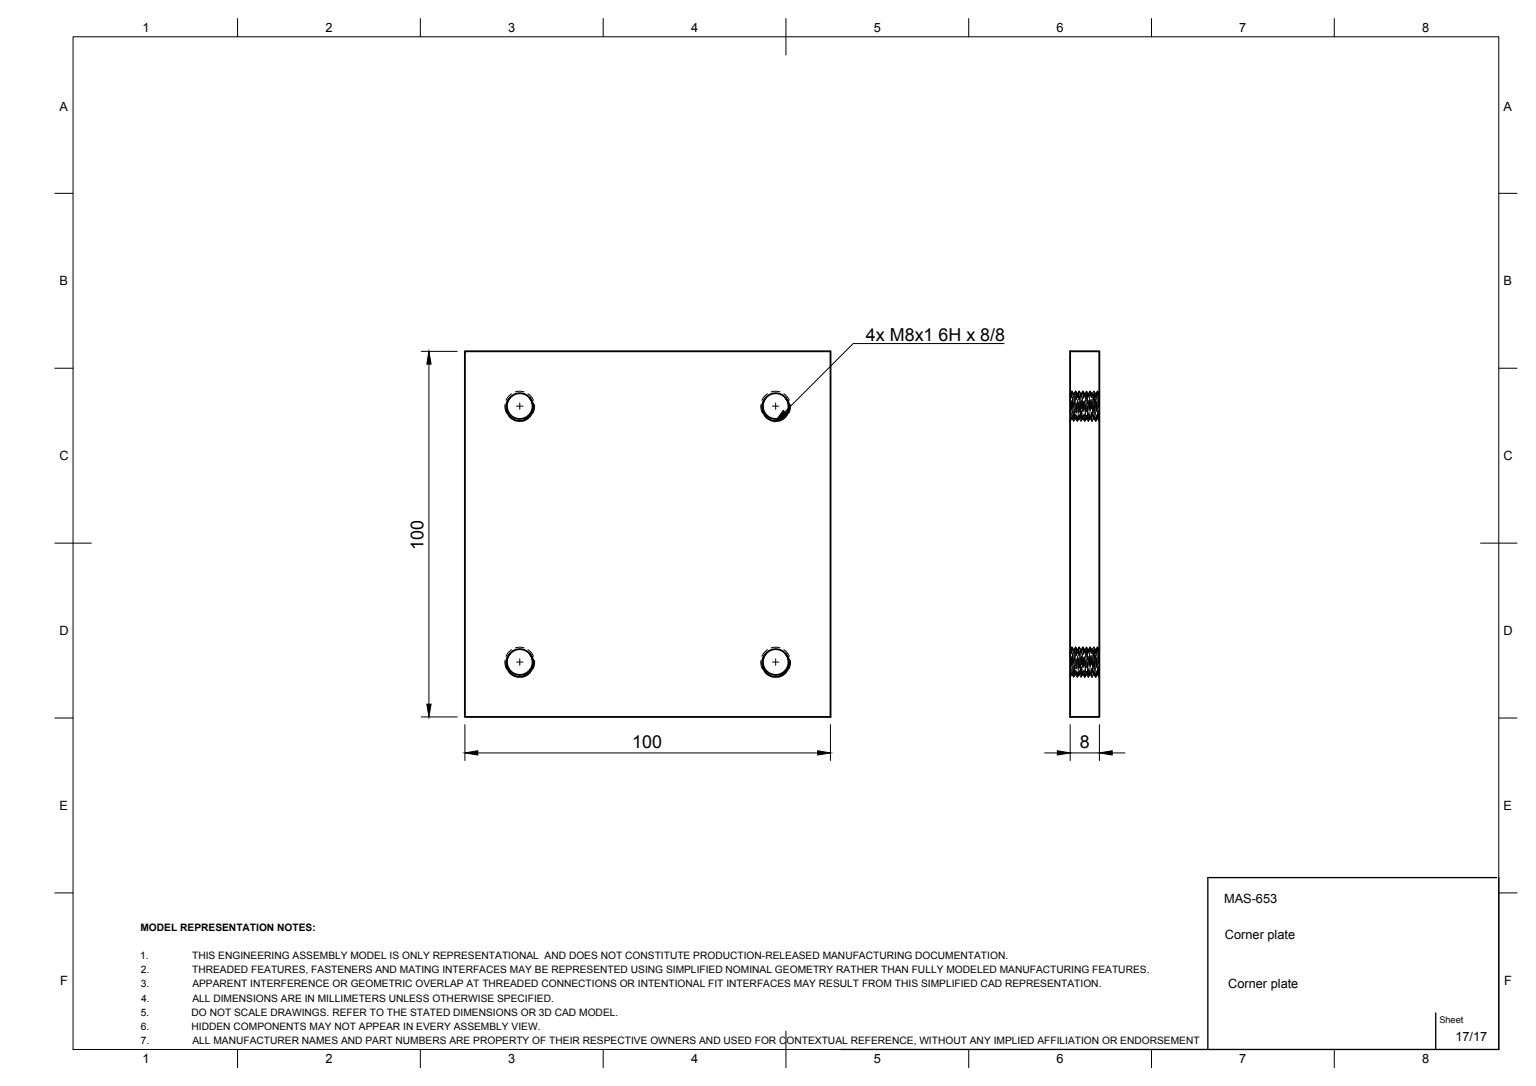
ISO-10303-21;
HEADER;
/* Generated by software containing ST-Developer
 * from STEP Tools, Inc. (www.steptools.com) 
 */

FILE_DESCRIPTION(
/* description */ ('Independent compact industrial fixture table, bolted aluminum worktop
 on connected adjustable support base. Whole-mm nominal dimensions. No
 load rating assigned.'),
/* implementation_level */ '2;1');

FILE_NAME(
/* name */ 'Corner plate.step',
/* time_stamp */ '2026-11-07T17:47:58-08:00',
/* author */ (''),
/* organization */ (''),
/* preprocessor_version */ 'ST-DEVELOPER v20.2',
/* originating_system */ 'Autodesk Translation Framework v15.17.0.0',
/* authorisation */ '');

FILE_SCHEMA (('AUTOMOTIVE_DESIGN { 1 0 10303 214 3 1 1 }'));
ENDSEC;

DATA;
#10=MECHANICAL_DESIGN_GEOMETRIC_PRESENTATION_REPRESENTATION('',(#2252),#97475);
#334=B_SPLINE_SURFACE_WITH_KNOTS('',3,3,((#29999,#30000,#30001,#30002,#30003,
#30004,#30005,#30006,#30007,#30008,#30009,#30010,#30011,#30012,#30013,#30014,
#30015,#30016,#30017,#30018,#30019,#30020,#30021,#30022,#30023,#30024,#30025,
#30026,#30027,#30028,#30029,#30030,#30031,#30032,#30033,#30034,#30035,#30036,
#30037,#30038,#30039,#30040,#30041,#30042,#30043,#30044,#30045,#30046,#30047,
#30048,#30049,#30050,#30051,#30052,#30053,#30054),(#30055,#30056,#30057,
#30058,#30059,#30060,#30061,#30062,#30063,#30064,#30065,#30066,#30067,#30068,
#30069,#30070,#30071,#30072,#30073,#30074,#30075,#30076,#30077,#30078,#30079,
#30080,#30081,#30082,#30083,#30084,#30085,#30086,#30087,#30088,#30089,#30090,
#30091,#30092,#30093,#30094,#30095,#30096,#30097,#30098,#30099,#30100,#30101,
#30102,#30103,#30104,#30105,#30106,#30107,#30108,#30109,#30110),(#30111,
#30112,#30113,#30114,#30115,#30116,#30117,#30118,#30119,#30120,#30121,#30122,
#30123,#30124,#30125,#30126,#30127,#30128,#30129,#30130,#30131,#30132,#30133,
#30134,#30135,#30136,#30137,#30138,#30139,#30140,#30141,#30142,#30143,#30144,
#30145,#30146,#30147,#30148,#30149,#30150,#30151,#30152,#30153,#30154,#30155,
#30156,#30157,#30158,#30159,#30160,#30161,#30162,#30163,#30164,#30165,#30166),
(#30167,#30168,#30169,#30170,#30171,#30172,#30173,#30174,#30175,#30176,
#30177,#30178,#30179,#30180,#30181,#30182,#30183,#30184,#30185,#30186,#30187,
#30188,#30189,#30190,#30191,#30192,#30193,#30194,#30195,#30196,#30197,#30198,
#30199,#30200,#30201,#30202,#30203,#30204,#30205,#30206,#30207,#30208,#30209,
#30210,#30211,#30212,#30213,#30214,#30215,#30216,#30217,#30218,#30219,#30220,
#30221,#30222)),.UNSPECIFIED.,.F.,.F.,.F.,(4,4),(4,1,1,1,1,1,1,1,1,1,1,
1,1,1,1,1,1,1,1,1,1,1,1,1,1,1,1,1,1,1,1,1,1,1,1,1,1,1,1,1,1,1,1,1,1,1,1,
1,1,1,1,1,1,4),(0.,0.0642013499338865),(11.8589888623078,12.8454497557128,
13.8319106491178,14.8183715425228,15.8048324359278,16.7912933293328,17.7777542227378,
18.7642151161428,19.7506760095478,20.7371369029528,21.7235977963578,22.7100586897628,
23.6965195831678,24.6829804765728,25.6694413699778,26.6559022633828,27.6423631567878,
28.6288240501928,29.6152849435978,30.6017458370028,31.5882067304078,32.5746676238129,
33.5611285172179,34.5475894106229,35.5340503040279,36.5205111974329,37.5069720908379,
38.4934329842429,39.4798938776479,40.4663547710529,41.4528156644579,42.4392765578629,
43.4257374512679,44.4121983446729,45.3986592380779,46.3851201314829,47.3715810248879,
48.3580419182929,49.3445028116979,50.3309637051029,51.3174245985079,52.3038854919129,
53.2903463853179,54.2768072787229,55.2632681721279,56.2497290655329,57.2361899589379,
58.2226508523429,59.2091117457479,60.1955726391529,61.1820335325579,62.1684944259629,
63.1549553193679,64.1414162127729),.UNSPECIFIED.);
#335=B_SPLINE_SURFACE_WITH_KNOTS('',3,3,((#30439,#30440,#30441,#30442,#30443,
#30444,#30445,#30446,#30447,#30448,#30449,#30450,#30451,#30452,#30453,#30454,
#30455,#30456,#30457,#30458,#30459,#30460,#30461,#30462,#30463,#30464,#30465,
#30466,#30467,#30468,#30469,#30470,#30471,#30472,#30473,#30474,#30475,#30476,
#30477,#30478,#30479,#30480,#30481,#30482,#30483,#30484,#30485,#30486,#30487,
#30488,#30489,#30490,#30491,#30492,#30493,#30494),(#30495,#30496,#30497,
#30498,#30499,#30500,#30501,#30502,#30503,#30504,#30505,#30506,#30507,#30508,
#30509,#30510,#30511,#30512,#30513,#30514,#30515,#30516,#30517,#30518,#30519,
#30520,#30521,#30522,#30523,#30524,#30525,#30526,#30527,#30528,#30529,#30530,
#30531,#30532,#30533,#30534,#30535,#30536,#30537,#30538,#30539,#30540,#30541,
#30542,#30543,#30544,#30545,#30546,#30547,#30548,#30549,#30550),(#30551,
#30552,#30553,#30554,#30555,#30556,#30557,#30558,#30559,#30560,#30561,#30562,
#30563,#30564,#30565,#30566,#30567,#30568,#30569,#30570,#30571,#30572,#30573,
#30574,#30575,#30576,#30577,#30578,#30579,#30580,#30581,#30582,#30583,#30584,
#30585,#30586,#30587,#30588,#30589,#30590,#30591,#30592,#30593,#30594,#30595,
#30596,#30597,#30598,#30599,#30600,#30601,#30602,#30603,#30604,#30605,#30606),
(#30607,#30608,#30609,#30610,#30611,#30612,#30613,#30614,#30615,#30616,
#30617,#30618,#30619,#30620,#30621,#30622,#30623,#30624,#30625,#30626,#30627,
#30628,#30629,#30630,#30631,#30632,#30633,#30634,#30635,#30636,#30637,#30638,
#30639,#30640,#30641,#30642,#30643,#30644,#30645,#30646,#30647,#30648,#30649,
#30650,#30651,#30652,#30653,#30654,#30655,#30656,#30657,#30658,#30659,#30660,
#30661,#30662)),.UNSPECIFIED.,.F.,.F.,.F.,(4,4),(4,1,1,1,1,1,1,1,1,1,1,
1,1,1,1,1,1,1,1,1,1,1,1,1,1,1,1,1,1,1,1,1,1,1,1,1,1,1,1,1,1,1,1,1,1,1,1,
1,1,1,1,1,1,4),(0.,0.0642013499338865),(14.3984001269718,15.3848610203768,
16.3713219137818,17.3577828071868,18.3442437005918,19.3307045939968,20.3171654874019,
21.3036263808069,22.2900872742119,23.2765481676169,24.2630090610219,25.2494699544269,
26.2359308478319,27.2223917412369,28.2088526346419,29.1953135280469,30.1817744214519,
31.1682353148569,32.1546962082619,33.1411571016669,34.1276179950719,35.1140788884769,
36.1005397818819,37.0870006752869,38.0734615686919,39.0599224620969,40.0463833555019,
41.0328442489069,42.0193051423119,43.0057660357169,43.9922269291219,44.9786878225269,
45.9651487159319,46.9516096093369,47.9380705027419,48.9245313961469,49.9109922895519,
50.8974531829569,51.8839140763619,52.8703749697669,53.856835863172,54.843296756577,
55.829757649982,56.816218543387,57.802679436792,58.789140330197,59.775601223602,
60.762062117007,61.748523010412,62.734983903817,63.721444797222,64.707905690627,
65.694366584032,66.680827477437),.UNSPECIFIED.);
#336=B_SPLINE_SURFACE_WITH_KNOTS('',3,3,((#31483,#31484,#31485,#31486,#31487,
#31488,#31489,#31490,#31491,#31492,#31493,#31494,#31495,#31496,#31497,#31498,
#31499,#31500,#31501,#31502,#31503,#31504,#31505,#31506,#31507,#31508,#31509,
#31510,#31511,#31512,#31513,#31514,#31515,#31516,#31517,#31518,#31519,#31520,
#31521,#31522,#31523,#31524,#31525,#31526,#31527,#31528,#31529,#31530,#31531,
#31532,#31533,#31534,#31535,#31536,#31537,#31538),(#31539,#31540,#31541,
#31542,#31543,#31544,#31545,#31546,#31547,#31548,#31549,#31550,#31551,#31552,
#31553,#31554,#31555,#31556,#31557,#31558,#31559,#31560,#31561,#31562,#31563,
#31564,#31565,#31566,#31567,#31568,#31569,#31570,#31571,#31572,#31573,#31574,
#31575,#31576,#31577,#31578,#31579,#31580,#31581,#31582,#31583,#31584,#31585,
#31586,#31587,#31588,#31589,#31590,#31591,#31592,#31593,#31594),(#31595,
#31596,#31597,#31598,#31599,#31600,#31601,#31602,#31603,#31604,#31605,#31606,
#31607,#31608,#31609,#31610,#31611,#31612,#31613,#31614,#31615,#31616,#31617,
#31618,#31619,#31620,#31621,#31622,#31623,#31624,#31625,#31626,#31627,#31628,
#31629,#31630,#31631,#31632,#31633,#31634,#31635,#31636,#31637,#31638,#31639,
#31640,#31641,#31642,#31643,#31644,#31645,#31646,#31647,#31648,#31649,#31650),
(#31651,#31652,#31653,#31654,#31655,#31656,#31657,#31658,#31659,#31660,
#31661,#31662,#31663,#31664,#31665,#31666,#31667,#31668,#31669,#31670,#31671,
#31672,#31673,#31674,#31675,#31676,#31677,#31678,#31679,#31680,#31681,#31682,
#31683,#31684,#31685,#31686,#31687,#31688,#31689,#31690,#31691,#31692,#31693,
#31694,#31695,#31696,#31697,#31698,#31699,#31700,#31701,#31702,#31703,#31704,
#31705,#31706)),.UNSPECIFIED.,.F.,.F.,.F.,(4,4),(4,1,1,1,1,1,1,1,1,1,1,
1,1,1,1,1,1,1,1,1,1,1,1,1,1,1,1,1,1,1,1,1,1,1,1,1,1,1,1,1,1,1,1,1,1,1,1,
1,1,1,1,1,1,4),(0.,0.0642013499338865),(11.8589888623078,12.8454497557128,
13.8319106491178,14.8183715425228,15.8048324359278,16.7912933293328,17.7777542227378,
18.7642151161428,19.7506760095478,20.7371369029528,21.7235977963578,22.7100586897628,
23.6965195831678,24.6829804765728,25.6694413699778,26.6559022633828,27.6423631567879,
28.6288240501929,29.6152849435979,30.6017458370029,31.5882067304079,32.5746676238129,
33.5611285172179,34.5475894106229,35.5340503040279,36.5205111974329,37.5069720908379,
38.4934329842429,39.4798938776479,40.4663547710529,41.4528156644579,42.4392765578629,
43.4257374512679,44.4121983446729,45.3986592380779,46.3851201314829,47.3715810248879,
48.3580419182929,49.3445028116979,50.3309637051029,51.3174245985079,52.3038854919129,
53.2903463853179,54.2768072787229,55.2632681721279,56.2497290655329,57.2361899589379,
58.2226508523429,59.2091117457479,60.1955726391529,61.1820335325579,62.1684944259629,
63.154955319368,64.141416212773),.UNSPECIFIED.);
#337=B_SPLINE_SURFACE_WITH_KNOTS('',3,3,((#31829,#31830,#31831,#31832,#31833,
#31834,#31835,#31836,#31837,#31838,#31839,#31840,#31841,#31842,#31843,#31844,
#31845,#31846,#31847,#31848,#31849,#31850,#31851,#31852,#31853,#31854,#31855,
#31856,#31857,#31858,#31859,#31860,#31861,#31862,#31863,#31864,#31865,#31866,
#31867,#31868,#31869,#31870,#31871,#31872,#31873,#31874,#31875,#31876,#31877,
#31878,#31879,#31880,#31881,#31882,#31883,#31884),(#31885,#31886,#31887,
#31888,#31889,#31890,#31891,#31892,#31893,#31894,#31895,#31896,#31897,#31898,
#31899,#31900,#31901,#31902,#31903,#31904,#31905,#31906,#31907,#31908,#31909,
#31910,#31911,#31912,#31913,#31914,#31915,#31916,#31917,#31918,#31919,#31920,
#31921,#31922,#31923,#31924,#31925,#31926,#31927,#31928,#31929,#31930,#31931,
#31932,#31933,#31934,#31935,#31936,#31937,#31938,#31939,#31940),(#31941,
#31942,#31943,#31944,#31945,#31946,#31947,#31948,#31949,#31950,#31951,#31952,
#31953,#31954,#31955,#31956,#31957,#31958,#31959,#31960,#31961,#31962,#31963,
#31964,#31965,#31966,#31967,#31968,#31969,#31970,#31971,#31972,#31973,#31974,
#31975,#31976,#31977,#31978,#31979,#31980,#31981,#31982,#31983,#31984,#31985,
#31986,#31987,#31988,#31989,#31990,#31991,#31992,#31993,#31994,#31995,#31996),
(#31997,#31998,#31999,#32000,#32001,#32002,#32003,#32004,#32005,#32006,
#32007,#32008,#32009,#32010,#32011,#32012,#32013,#32014,#32015,#32016,#32017,
#32018,#32019,#32020,#32021,#32022,#32023,#32024,#32025,#32026,#32027,#32028,
#32029,#32030,#32031,#32032,#32033,#32034,#32035,#32036,#32037,#32038,#32039,
#32040,#32041,#32042,#32043,#32044,#32045,#32046,#32047,#32048,#32049,#32050,
#32051,#32052)),.UNSPECIFIED.,.F.,.F.,.F.,(4,4),(4,1,1,1,1,1,1,1,1,1,1,
1,1,1,1,1,1,1,1,1,1,1,1,1,1,1,1,1,1,1,1,1,1,1,1,1,1,1,1,1,1,1,1,1,1,1,1,
1,1,1,1,1,1,4),(0.,0.0642013499338865),(14.3984001269718,15.3848610203768,
16.3713219137818,17.3577828071869,18.3442437005919,19.3307045939969,20.3171654874019,
21.3036263808069,22.2900872742119,23.2765481676169,24.2630090610219,25.2494699544269,
26.2359308478319,27.2223917412369,28.2088526346419,29.1953135280469,30.1817744214519,
31.1682353148569,32.1546962082619,33.1411571016669,34.1276179950719,35.1140788884769,
36.1005397818819,37.0870006752869,38.0734615686919,39.0599224620969,40.0463833555019,
41.0328442489069,42.0193051423119,43.0057660357169,43.9922269291219,44.9786878225269,
45.9651487159319,46.9516096093369,47.9380705027419,48.9245313961469,49.9109922895519,
50.8974531829569,51.8839140763619,52.8703749697669,53.856835863172,54.843296756577,
55.829757649982,56.816218543387,57.802679436792,58.789140330197,59.775601223602,
60.762062117007,61.748523010412,62.734983903817,63.721444797222,64.707905690627,
65.694366584032,66.680827477437),.UNSPECIFIED.);
#338=B_SPLINE_SURFACE_WITH_KNOTS('',3,3,((#32194,#32195,#32196,#32197,#32198,
#32199,#32200,#32201,#32202,#32203,#32204,#32205,#32206,#32207,#32208,#32209,
#32210,#32211,#32212,#32213,#32214,#32215,#32216,#32217,#32218,#32219,#32220,
#32221,#32222,#32223,#32224,#32225,#32226,#32227,#32228,#32229,#32230,#32231,
#32232,#32233,#32234,#32235,#32236,#32237,#32238,#32239,#32240,#32241,#32242,
#32243,#32244,#32245,#32246,#32247,#32248,#32249),(#32250,#32251,#32252,
#32253,#32254,#32255,#32256,#32257,#32258,#32259,#32260,#32261,#32262,#32263,
#32264,#32265,#32266,#32267,#32268,#32269,#32270,#32271,#32272,#32273,#32274,
#32275,#32276,#32277,#32278,#32279,#32280,#32281,#32282,#32283,#32284,#32285,
#32286,#32287,#32288,#32289,#32290,#32291,#32292,#32293,#32294,#32295,#32296,
#32297,#32298,#32299,#32300,#32301,#32302,#32303,#32304,#32305),(#32306,
#32307,#32308,#32309,#32310,#32311,#32312,#32313,#32314,#32315,#32316,#32317,
#32318,#32319,#32320,#32321,#32322,#32323,#32324,#32325,#32326,#32327,#32328,
#32329,#32330,#32331,#32332,#32333,#32334,#32335,#32336,#32337,#32338,#32339,
#32340,#32341,#32342,#32343,#32344,#32345,#32346,#32347,#32348,#32349,#32350,
#32351,#32352,#32353,#32354,#32355,#32356,#32357,#32358,#32359,#32360,#32361),
(#32362,#32363,#32364,#32365,#32366,#32367,#32368,#32369,#32370,#32371,
#32372,#32373,#32374,#32375,#32376,#32377,#32378,#32379,#32380,#32381,#32382,
#32383,#32384,#32385,#32386,#32387,#32388,#32389,#32390,#32391,#32392,#32393,
#32394,#32395,#32396,#32397,#32398,#32399,#32400,#32401,#32402,#32403,#32404,
#32405,#32406,#32407,#32408,#32409,#32410,#32411,#32412,#32413,#32414,#32415,
#32416,#32417)),.UNSPECIFIED.,.F.,.F.,.F.,(4,4),(4,1,1,1,1,1,1,1,1,1,1,
1,1,1,1,1,1,1,1,1,1,1,1,1,1,1,1,1,1,1,1,1,1,1,1,1,1,1,1,1,1,1,1,1,1,1,1,
1,1,1,1,1,1,4),(0.,0.0642013499338865),(11.8589888623078,12.8454497557128,
13.8319106491178,14.8183715425228,15.8048324359278,16.7912933293328,17.7777542227378,
18.7642151161428,19.7506760095478,20.7371369029528,21.7235977963578,22.7100586897628,
23.6965195831678,24.6829804765728,25.6694413699778,26.6559022633828,27.6423631567878,
28.6288240501928,29.6152849435978,30.6017458370028,31.5882067304078,32.5746676238129,
33.5611285172179,34.5475894106229,35.5340503040279,36.5205111974329,37.5069720908379,
38.4934329842429,39.4798938776479,40.4663547710529,41.4528156644579,42.4392765578629,
43.4257374512679,44.4121983446729,45.3986592380779,46.3851201314829,47.3715810248879,
48.3580419182929,49.3445028116979,50.3309637051029,51.3174245985079,52.3038854919129,
53.2903463853179,54.2768072787229,55.2632681721279,56.2497290655329,57.2361899589379,
58.2226508523429,59.2091117457479,60.1955726391529,61.1820335325579,62.1684944259629,
63.1549553193679,64.1414162127729),.UNSPECIFIED.);
#339=B_SPLINE_SURFACE_WITH_KNOTS('',3,3,((#32540,#32541,#32542,#32543,#32544,
#32545,#32546,#32547,#32548,#32549,#32550,#32551,#32552,#32553,#32554,#32555,
#32556,#32557,#32558,#32559,#32560,#32561,#32562,#32563,#32564,#32565,#32566,
#32567,#32568,#32569,#32570,#32571,#32572,#32573,#32574,#32575,#32576,#32577,
#32578,#32579,#32580,#32581,#32582,#32583,#32584,#32585,#32586,#32587,#32588,
#32589,#32590,#32591,#32592,#32593,#32594,#32595),(#32596,#32597,#32598,
#32599,#32600,#32601,#32602,#32603,#32604,#32605,#32606,#32607,#32608,#32609,
#32610,#32611,#32612,#32613,#32614,#32615,#32616,#32617,#32618,#32619,#32620,
#32621,#32622,#32623,#32624,#32625,#32626,#32627,#32628,#32629,#32630,#32631,
#32632,#32633,#32634,#32635,#32636,#32637,#32638,#32639,#32640,#32641,#32642,
#32643,#32644,#32645,#32646,#32647,#32648,#32649,#32650,#32651),(#32652,
#32653,#32654,#32655,#32656,#32657,#32658,#32659,#32660,#32661,#32662,#32663,
#32664,#32665,#32666,#32667,#32668,#32669,#32670,#32671,#32672,#32673,#32674,
#32675,#32676,#32677,#32678,#32679,#32680,#32681,#32682,#32683,#32684,#32685,
#32686,#32687,#32688,#32689,#32690,#32691,#32692,#32693,#32694,#32695,#32696,
#32697,#32698,#32699,#32700,#32701,#32702,#32703,#32704,#32705,#32706,#32707),
(#32708,#32709,#32710,#32711,#32712,#32713,#32714,#32715,#32716,#32717,
#32718,#32719,#32720,#32721,#32722,#32723,#32724,#32725,#32726,#32727,#32728,
#32729,#32730,#32731,#32732,#32733,#32734,#32735,#32736,#32737,#32738,#32739,
#32740,#32741,#32742,#32743,#32744,#32745,#32746,#32747,#32748,#32749,#32750,
#32751,#32752,#32753,#32754,#32755,#32756,#32757,#32758,#32759,#32760,#32761,
#32762,#32763)),.UNSPECIFIED.,.F.,.F.,.F.,(4,4),(4,1,1,1,1,1,1,1,1,1,1,
1,1,1,1,1,1,1,1,1,1,1,1,1,1,1,1,1,1,1,1,1,1,1,1,1,1,1,1,1,1,1,1,1,1,1,1,
1,1,1,1,1,1,4),(0.,0.0642013499338865),(14.3984001269718,15.3848610203768,
16.3713219137818,17.3577828071868,18.3442437005918,19.3307045939968,20.3171654874019,
21.3036263808069,22.2900872742119,23.2765481676169,24.2630090610219,25.2494699544269,
26.2359308478319,27.2223917412369,28.2088526346419,29.1953135280469,30.1817744214519,
31.1682353148569,32.1546962082619,33.1411571016669,34.1276179950719,35.1140788884769,
36.1005397818819,37.0870006752869,38.0734615686919,39.0599224620969,40.0463833555019,
41.0328442489069,42.0193051423119,43.0057660357169,43.9922269291219,44.9786878225269,
45.9651487159319,46.9516096093369,47.9380705027419,48.9245313961469,49.9109922895519,
50.8974531829569,51.8839140763619,52.8703749697669,53.856835863172,54.843296756577,
55.829757649982,56.816218543387,57.802679436792,58.789140330197,59.775601223602,
60.762062117007,61.748523010412,62.734983903817,63.721444797222,64.707905690627,
65.694366584032,66.680827477437),.UNSPECIFIED.);
#340=B_SPLINE_SURFACE_WITH_KNOTS('',3,3,((#32905,#32906,#32907,#32908,#32909,
#32910,#32911,#32912,#32913,#32914,#32915,#32916,#32917,#32918,#32919,#32920,
#32921,#32922,#32923,#32924,#32925,#32926,#32927,#32928,#32929,#32930,#32931,
#32932,#32933,#32934,#32935,#32936,#32937,#32938,#32939,#32940,#32941,#32942,
#32943,#32944,#32945,#32946,#32947,#32948,#32949,#32950,#32951,#32952,#32953,
#32954,#32955,#32956,#32957,#32958,#32959,#32960),(#32961,#32962,#32963,
#32964,#32965,#32966,#32967,#32968,#32969,#32970,#32971,#32972,#32973,#32974,
#32975,#32976,#32977,#32978,#32979,#32980,#32981,#32982,#32983,#32984,#32985,
#32986,#32987,#32988,#32989,#32990,#32991,#32992,#32993,#32994,#32995,#32996,
#32997,#32998,#32999,#33000,#33001,#33002,#33003,#33004,#33005,#33006,#33007,
#33008,#33009,#33010,#33011,#33012,#33013,#33014,#33015,#33016),(#33017,
#33018,#33019,#33020,#33021,#33022,#33023,#33024,#33025,#33026,#33027,#33028,
#33029,#33030,#33031,#33032,#33033,#33034,#33035,#33036,#33037,#33038,#33039,
#33040,#33041,#33042,#33043,#33044,#33045,#33046,#33047,#33048,#33049,#33050,
#33051,#33052,#33053,#33054,#33055,#33056,#33057,#33058,#33059,#33060,#33061,
#33062,#33063,#33064,#33065,#33066,#33067,#33068,#33069,#33070,#33071,#33072),
(#33073,#33074,#33075,#33076,#33077,#33078,#33079,#33080,#33081,#33082,
#33083,#33084,#33085,#33086,#33087,#33088,#33089,#33090,#33091,#33092,#33093,
#33094,#33095,#33096,#33097,#33098,#33099,#33100,#33101,#33102,#33103,#33104,
#33105,#33106,#33107,#33108,#33109,#33110,#33111,#33112,#33113,#33114,#33115,
#33116,#33117,#33118,#33119,#33120,#33121,#33122,#33123,#33124,#33125,#33126,
#33127,#33128)),.UNSPECIFIED.,.F.,.F.,.F.,(4,4),(4,1,1,1,1,1,1,1,1,1,1,
1,1,1,1,1,1,1,1,1,1,1,1,1,1,1,1,1,1,1,1,1,1,1,1,1,1,1,1,1,1,1,1,1,1,1,1,
1,1,1,1,1,1,4),(0.,0.0642013499338865),(11.8589888623078,12.8454497557128,
13.8319106491178,14.8183715425228,15.8048324359278,16.7912933293328,17.7777542227378,
18.7642151161428,19.7506760095478,20.7371369029528,21.7235977963578,22.7100586897628,
23.6965195831678,24.6829804765728,25.6694413699778,26.6559022633828,27.6423631567879,
28.6288240501929,29.6152849435979,30.6017458370029,31.5882067304079,32.5746676238129,
33.5611285172179,34.5475894106229,35.5340503040279,36.5205111974329,37.5069720908379,
38.4934329842429,39.4798938776479,40.4663547710529,41.4528156644579,42.4392765578629,
43.4257374512679,44.4121983446729,45.3986592380779,46.3851201314829,47.3715810248879,
48.3580419182929,49.3445028116979,50.3309637051029,51.3174245985079,52.3038854919129,
53.2903463853179,54.2768072787229,55.2632681721279,56.2497290655329,57.2361899589379,
58.2226508523429,59.2091117457479,60.1955726391529,61.1820335325579,62.1684944259629,
63.154955319368,64.141416212773),.UNSPECIFIED.);
#341=B_SPLINE_SURFACE_WITH_KNOTS('',3,3,((#33251,#33252,#33253,#33254,#33255,
#33256,#33257,#33258,#33259,#33260,#33261,#33262,#33263,#33264,#33265,#33266,
#33267,#33268,#33269,#33270,#33271,#33272,#33273,#33274,#33275,#33276,#33277,
#33278,#33279,#33280,#33281,#33282,#33283,#33284,#33285,#33286,#33287,#33288,
#33289,#33290,#33291,#33292,#33293,#33294,#33295,#33296,#33297,#33298,#33299,
#33300,#33301,#33302,#33303,#33304,#33305,#33306),(#33307,#33308,#33309,
#33310,#33311,#33312,#33313,#33314,#33315,#33316,#33317,#33318,#33319,#33320,
#33321,#33322,#33323,#33324,#33325,#33326,#33327,#33328,#33329,#33330,#33331,
#33332,#33333,#33334,#33335,#33336,#33337,#33338,#33339,#33340,#33341,#33342,
#33343,#33344,#33345,#33346,#33347,#33348,#33349,#33350,#33351,#33352,#33353,
#33354,#33355,#33356,#33357,#33358,#33359,#33360,#33361,#33362),(#33363,
#33364,#33365,#33366,#33367,#33368,#33369,#33370,#33371,#33372,#33373,#33374,
#33375,#33376,#33377,#33378,#33379,#33380,#33381,#33382,#33383,#33384,#33385,
#33386,#33387,#33388,#33389,#33390,#33391,#33392,#33393,#33394,#33395,#33396,
#33397,#33398,#33399,#33400,#33401,#33402,#33403,#33404,#33405,#33406,#33407,
#33408,#33409,#33410,#33411,#33412,#33413,#33414,#33415,#33416,#33417,#33418),
(#33419,#33420,#33421,#33422,#33423,#33424,#33425,#33426,#33427,#33428,
#33429,#33430,#33431,#33432,#33433,#33434,#33435,#33436,#33437,#33438,#33439,
#33440,#33441,#33442,#33443,#33444,#33445,#33446,#33447,#33448,#33449,#33450,
#33451,#33452,#33453,#33454,#33455,#33456,#33457,#33458,#33459,#33460,#33461,
#33462,#33463,#33464,#33465,#33466,#33467,#33468,#33469,#33470,#33471,#33472,
#33473,#33474)),.UNSPECIFIED.,.F.,.F.,.F.,(4,4),(4,1,1,1,1,1,1,1,1,1,1,
1,1,1,1,1,1,1,1,1,1,1,1,1,1,1,1,1,1,1,1,1,1,1,1,1,1,1,1,1,1,1,1,1,1,1,1,
1,1,1,1,1,1,4),(0.,0.0642013499338865),(14.3984001269718,15.3848610203768,
16.3713219137818,17.3577828071869,18.3442437005919,19.3307045939969,20.3171654874019,
21.3036263808069,22.2900872742119,23.2765481676169,24.2630090610219,25.2494699544269,
26.2359308478319,27.2223917412369,28.2088526346419,29.1953135280469,30.1817744214519,
31.1682353148569,32.1546962082619,33.1411571016669,34.1276179950719,35.1140788884769,
36.1005397818819,37.0870006752869,38.0734615686919,39.0599224620969,40.0463833555019,
41.0328442489069,42.0193051423119,43.0057660357169,43.9922269291219,44.9786878225269,
45.9651487159319,46.9516096093369,47.9380705027419,48.9245313961469,49.9109922895519,
50.8974531829569,51.8839140763619,52.8703749697669,53.856835863172,54.843296756577,
55.829757649982,56.816218543387,57.802679436792,58.789140330197,59.775601223602,
60.762062117007,61.748523010412,62.734983903817,63.721444797222,64.707905690627,
65.694366584032,66.680827477437),.UNSPECIFIED.);
#376=B_SPLINE_CURVE_WITH_KNOTS('',3,(#27786,#27787,#27788,#27789),
 .UNSPECIFIED.,.F.,.F.,(4,4),(51.5750455984138,52.2824273504652),
 .UNSPECIFIED.);
#377=B_SPLINE_CURVE_WITH_KNOTS('',3,(#27792,#27793,#27794,#27795,#27796,
#27797,#27798,#27799,#27800,#27801),.UNSPECIFIED.,.F.,.F.,(4,3,3,4),(-50.2654824574367,
-49.3230446702501,-48.3365837768451,-47.8312715558983),.UNSPECIFIED.);
#378=B_SPLINE_CURVE_WITH_KNOTS('',3,(#27806,#27807,#27808,#27809,#27810,
#27811,#27812,#27813,#27814,#27815,#27816,#27817,#27818,#27819,#27820,#27821,
#27822,#27823,#27824,#27825,#27826,#27827,#27828,#27829,#27830),
 .UNSPECIFIED.,.F.,.F.,(4,3,3,3,3,3,3,3,4),(45.2918602912342,45.3772010966301,
46.3636619900351,47.3501228834401,48.3365837768452,49.3230446702501,50.3095055636552,
51.2959664570602,51.5750455984138),.UNSPECIFIED.);
#379=B_SPLINE_CURVE_WITH_KNOTS('',3,(#27831,#27832,#27833,#27834,#27835,
#27836,#27837,#27838,#27839,#27840,#27841,#27842,#27843,#27844,#27845,#27846,
#27847,#27848,#27849,#27850,#27851,#27852),.UNSPECIFIED.,.F.,.F.,(4,3,3,
3,3,3,3,4),(-47.8312715558983,-47.3501228834401,-46.3636619900351,-45.3772010966301,
-44.3907402032251,-43.4042793098201,-42.4178184164151,-41.5480862487187),
 .UNSPECIFIED.);
#380=B_SPLINE_CURVE_WITH_KNOTS('',3,(#27857,#27858,#27859,#27860,#27861,
#27862,#27863,#27864,#27865,#27866,#27867,#27868,#27869,#27870,#27871,#27872,
#27873,#27874,#27875,#27876,#27877,#27878),.UNSPECIFIED.,.F.,.F.,(4,3,3,
3,3,3,3,4),(39.0086749840546,39.4584357362001,40.4448966296051,41.4313575230101,
42.4178184164151,43.4042793098201,44.3907402032251,45.2918602912342),
 .UNSPECIFIED.);
#381=B_SPLINE_CURVE_WITH_KNOTS('',3,(#27879,#27880,#27881,#27882,#27883,
#27884,#27885,#27886,#27887,#27888,#27889,#27890,#27891,#27892,#27893,#27894,
#27895,#27896,#27897,#27898,#27899,#27900,#27901,#27902,#27903),
 .UNSPECIFIED.,.F.,.F.,(4,3,3,3,3,3,3,3,4),(-41.5480862487187,-41.4313575230101,
-40.4448966296051,-39.4584357362001,-38.4719748427951,-37.4855139493901,
-36.4990530559851,-35.5125921625801,-35.2649009415391),.UNSPECIFIED.);
#382=B_SPLINE_CURVE_WITH_KNOTS('',3,(#27908,#27909,#27910,#27911,#27912,
#27913,#27914,#27915,#27916,#27917,#27918,#27919,#27920,#27921,#27922,#27923,
#27924,#27925,#27926,#27927,#27928,#27929),.UNSPECIFIED.,.F.,.F.,(4,3,3,
3,3,3,3,4),(32.725489676875,33.5396703757701,34.5261312691751,35.5125921625801,
36.4990530559851,37.4855139493901,38.4719748427951,39.0086749840546),
 .UNSPECIFIED.);
#383=B_SPLINE_CURVE_WITH_KNOTS('',3,(#27930,#27931,#27932,#27933,#27934,
#27935,#27936,#27937,#27938,#27939,#27940,#27941,#27942,#27943,#27944,#27945,
#27946,#27947,#27948,#27949,#27950,#27951),.UNSPECIFIED.,.F.,.F.,(4,3,3,
3,3,3,3,4),(-35.2649009415391,-34.5261312691751,-33.5396703757701,-32.5532094823651,
-31.5667485889601,-30.5802876955551,-29.5938268021501,-28.9817156343595),
 .UNSPECIFIED.);
#384=B_SPLINE_CURVE_WITH_KNOTS('',3,(#27956,#27957,#27958,#27959,#27960,
#27961,#27962,#27963,#27964,#27965,#27966,#27967,#27968,#27969,#27970,#27971,
#27972,#27973,#27974,#27975,#27976,#27977,#27978,#27979,#27980),
 .UNSPECIFIED.,.F.,.F.,(4,3,3,3,3,3,3,3,4),(26.4423043696954,26.6344441219351,
27.6209050153401,28.6073659087451,29.5938268021501,30.5802876955551,31.5667485889601,
32.5532094823651,32.725489676875),.UNSPECIFIED.);
#385=B_SPLINE_CURVE_WITH_KNOTS('',3,(#27981,#27982,#27983,#27984,#27985,
#27986,#27987,#27988,#27989,#27990,#27991,#27992,#27993,#27994,#27995,#27996,
#27997,#27998,#27999,#28000,#28001,#28002),.UNSPECIFIED.,.F.,.F.,(4,3,3,
3,3,3,3,4),(-28.9817156343595,-28.6073659087451,-27.6209050153401,-26.6344441219351,
-25.6479832285301,-24.6615223351251,-23.6750614417201,-22.6985303271799),
 .UNSPECIFIED.);
#386=B_SPLINE_CURVE_WITH_KNOTS('',3,(#28007,#28008,#28009,#28010,#28011,
#28012,#28013,#28014,#28015,#28016,#28017,#28018,#28019,#28020,#28021,#28022,
#28023,#28024,#28025,#28026,#28027,#28028),.UNSPECIFIED.,.F.,.F.,(4,3,3,
3,3,3,3,4),(20.1591190625159,20.7156787615051,21.7021396549101,22.6886005483151,
23.6750614417201,24.6615223351251,25.6479832285301,26.4423043696954),
 .UNSPECIFIED.);
#387=B_SPLINE_CURVE_WITH_KNOTS('',3,(#28029,#28030,#28031,#28032,#28033,
#28034,#28035,#28036,#28037,#28038,#28039,#28040,#28041,#28042,#28043,#28044,
#28045,#28046,#28047,#28048,#28049,#28050,#28051,#28052,#28053),
 .UNSPECIFIED.,.F.,.F.,(4,3,3,3,3,3,3,3,4),(-22.6985303271799,-22.6886005483151,
-21.7021396549101,-20.7156787615051,-19.7292178681001,-18.7427569746951,
-17.7562960812901,-16.7698351878851,-16.4153450200003),.UNSPECIFIED.);
#388=B_SPLINE_CURVE_WITH_KNOTS('',3,(#28058,#28059,#28060,#28061,#28062,
#28063,#28064,#28065,#28066,#28067,#28068,#28069,#28070,#28071,#28072,#28073,
#28074,#28075,#28076,#28077,#28078,#28079),.UNSPECIFIED.,.F.,.F.,(4,3,3,
3,3,3,3,4),(13.8759337553363,14.7969134010751,15.78337429448,16.7698351878851,
17.75629608129,18.7427569746951,19.7292178681001,20.1591190625159),
 .UNSPECIFIED.);
#389=B_SPLINE_CURVE_WITH_KNOTS('',3,(#28080,#28081,#28082,#28083,#28084,
#28085,#28086,#28087,#28088,#28089,#28090,#28091,#28092,#28093,#28094,#28095,
#28096,#28097,#28098,#28099,#28100,#28101),.UNSPECIFIED.,.F.,.F.,(4,3,3,
3,3,3,3,4),(-16.4153450200003,-15.78337429448,-14.796913401075,-13.81045250767,
-12.823991614265,-11.83753072086,-10.851069827455,-10.1321597128207),
 .UNSPECIFIED.);
#390=B_SPLINE_CURVE_WITH_KNOTS('',3,(#28107,#28108,#28109,#28110,#28111,
#28112,#28113,#28114,#28115,#28116,#28117,#28118,#28119),.UNSPECIFIED.,
 .F.,.F.,(4,3,3,3,4),(-3.84897440564115,-2.95938268021501,-1.97292178681001,
-0.986460893405001,0.),.UNSPECIFIED.);
#391=B_SPLINE_CURVE_WITH_KNOTS('',3,(#28122,#28123,#28124,#28125,#28126,
#28127,#28128,#28129,#28130,#28131,#28132,#28133,#28134,#28135,#28136,#28137,
#28138,#28139,#28140),.UNSPECIFIED.,.F.,.F.,(4,3,3,3,3,3,4),(2.01694489302848,
2.95938268021501,3.94584357362001,4.93230446702502,5.91876536043002,6.90522625383502,
7.59274844815668),.UNSPECIFIED.);
#392=B_SPLINE_CURVE_WITH_KNOTS('',3,(#28146,#28147,#28148,#28149),
 .UNSPECIFIED.,.F.,.F.,(4,4),(51.5750455984138,52.2824273504652),
 .UNSPECIFIED.);
#393=B_SPLINE_CURVE_WITH_KNOTS('',3,(#28152,#28153,#28154,#28155,#28156,
#28157,#28158,#28159,#28160,#28161),.UNSPECIFIED.,.F.,.F.,(4,3,3,4),(-50.2654824574367,
-49.3230446702501,-48.3365837768451,-47.8312715558982),.UNSPECIFIED.);
#394=B_SPLINE_CURVE_WITH_KNOTS('',3,(#28166,#28167,#28168,#28169,#28170,
#28171,#28172,#28173,#28174,#28175,#28176,#28177,#28178,#28179,#28180,#28181,
#28182,#28183,#28184,#28185,#28186,#28187,#28188,#28189,#28190),
 .UNSPECIFIED.,.F.,.F.,(4,3,3,3,3,3,3,3,4),(45.2918602912342,45.3772010966301,
46.3636619900351,47.3501228834401,48.3365837768451,49.3230446702501,50.3095055636551,
51.2959664570602,51.5750455984138),.UNSPECIFIED.);
#395=B_SPLINE_CURVE_WITH_KNOTS('',3,(#28191,#28192,#28193,#28194,#28195,
#28196,#28197,#28198,#28199,#28200,#28201,#28202,#28203,#28204,#28205,#28206,
#28207,#28208,#28209,#28210,#28211,#28212),.UNSPECIFIED.,.F.,.F.,(4,3,3,
3,3,3,3,4),(-47.8312715558982,-47.3501228834401,-46.3636619900351,-45.3772010966301,
-44.3907402032251,-43.4042793098201,-42.4178184164151,-41.5480862487187),
 .UNSPECIFIED.);
#396=B_SPLINE_CURVE_WITH_KNOTS('',3,(#28217,#28218,#28219,#28220,#28221,
#28222,#28223,#28224,#28225,#28226,#28227,#28228,#28229,#28230,#28231,#28232,
#28233,#28234,#28235,#28236,#28237,#28238),.UNSPECIFIED.,.F.,.F.,(4,3,3,
3,3,3,3,4),(39.0086749840546,39.4584357362001,40.4448966296051,41.4313575230101,
42.4178184164151,43.4042793098201,44.3907402032251,45.2918602912342),
 .UNSPECIFIED.);
#397=B_SPLINE_CURVE_WITH_KNOTS('',3,(#28239,#28240,#28241,#28242,#28243,
#28244,#28245,#28246,#28247,#28248,#28249,#28250,#28251,#28252,#28253,#28254,
#28255,#28256,#28257,#28258,#28259,#28260,#28261,#28262,#28263),
 .UNSPECIFIED.,.F.,.F.,(4,3,3,3,3,3,3,3,4),(-41.5480862487187,-41.4313575230101,
-40.4448966296051,-39.4584357362001,-38.4719748427951,-37.4855139493901,
-36.4990530559851,-35.5125921625801,-35.2649009415391),.UNSPECIFIED.);
#398=B_SPLINE_CURVE_WITH_KNOTS('',3,(#28268,#28269,#28270,#28271,#28272,
#28273,#28274,#28275,#28276,#28277,#28278,#28279,#28280,#28281,#28282,#28283,
#28284,#28285,#28286,#28287,#28288,#28289),.UNSPECIFIED.,.F.,.F.,(4,3,3,
3,3,3,3,4),(32.725489676875,33.5396703757701,34.5261312691751,35.5125921625801,
36.4990530559851,37.4855139493901,38.4719748427951,39.0086749840546),
 .UNSPECIFIED.);
#399=B_SPLINE_CURVE_WITH_KNOTS('',3,(#28290,#28291,#28292,#28293,#28294,
#28295,#28296,#28297,#28298,#28299,#28300,#28301,#28302,#28303,#28304,#28305,
#28306,#28307,#28308,#28309,#28310,#28311),.UNSPECIFIED.,.F.,.F.,(4,3,3,
3,3,3,3,4),(-35.2649009415391,-34.5261312691751,-33.5396703757701,-32.5532094823651,
-31.5667485889601,-30.5802876955551,-29.5938268021501,-28.9817156343595),
 .UNSPECIFIED.);
#400=B_SPLINE_CURVE_WITH_KNOTS('',3,(#28316,#28317,#28318,#28319,#28320,
#28321,#28322,#28323,#28324,#28325,#28326,#28327,#28328,#28329,#28330,#28331,
#28332,#28333,#28334,#28335,#28336,#28337,#28338,#28339,#28340),
 .UNSPECIFIED.,.F.,.F.,(4,3,3,3,3,3,3,3,4),(26.4423043696954,26.6344441219351,
27.6209050153401,28.6073659087451,29.5938268021501,30.5802876955551,31.5667485889601,
32.5532094823651,32.725489676875),.UNSPECIFIED.);
#401=B_SPLINE_CURVE_WITH_KNOTS('',3,(#28341,#28342,#28343,#28344,#28345,
#28346,#28347,#28348,#28349,#28350,#28351,#28352,#28353,#28354,#28355,#28356,
#28357,#28358,#28359,#28360,#28361,#28362),.UNSPECIFIED.,.F.,.F.,(4,3,3,
3,3,3,3,4),(-28.9817156343595,-28.6073659087451,-27.6209050153401,-26.6344441219351,
-25.6479832285301,-24.6615223351251,-23.6750614417201,-22.6985303271799),
 .UNSPECIFIED.);
#402=B_SPLINE_CURVE_WITH_KNOTS('',3,(#28367,#28368,#28369,#28370,#28371,
#28372,#28373,#28374,#28375,#28376,#28377,#28378,#28379,#28380,#28381,#28382,
#28383,#28384,#28385,#28386,#28387,#28388),.UNSPECIFIED.,.F.,.F.,(4,3,3,
3,3,3,3,4),(20.1591190625158,20.7156787615051,21.7021396549101,22.6886005483151,
23.6750614417201,24.6615223351251,25.6479832285301,26.4423043696954),
 .UNSPECIFIED.);
#403=B_SPLINE_CURVE_WITH_KNOTS('',3,(#28389,#28390,#28391,#28392,#28393,
#28394,#28395,#28396,#28397,#28398,#28399,#28400,#28401,#28402,#28403,#28404,
#28405,#28406,#28407,#28408,#28409,#28410,#28411,#28412,#28413),
 .UNSPECIFIED.,.F.,.F.,(4,3,3,3,3,3,3,3,4),(-22.6985303271799,-22.6886005483151,
-21.7021396549101,-20.7156787615051,-19.7292178681001,-18.7427569746951,
-17.7562960812901,-16.7698351878851,-16.4153450200003),.UNSPECIFIED.);
#404=B_SPLINE_CURVE_WITH_KNOTS('',3,(#28418,#28419,#28420,#28421,#28422,
#28423,#28424,#28425,#28426,#28427,#28428,#28429,#28430,#28431,#28432,#28433,
#28434,#28435,#28436,#28437,#28438,#28439),.UNSPECIFIED.,.F.,.F.,(4,3,3,
3,3,3,3,4),(13.8759337553363,14.796913401075,15.78337429448,16.7698351878851,
17.7562960812901,18.7427569746951,19.7292178681001,20.1591190625158),
 .UNSPECIFIED.);
#405=B_SPLINE_CURVE_WITH_KNOTS('',3,(#28440,#28441,#28442,#28443,#28444,
#28445,#28446,#28447,#28448,#28449,#28450,#28451,#28452,#28453,#28454,#28455,
#28456,#28457,#28458,#28459,#28460,#28461),.UNSPECIFIED.,.F.,.F.,(4,3,3,
3,3,3,3,4),(-16.4153450200003,-15.7833742944801,-14.796913401075,-13.81045250767,
-12.823991614265,-11.83753072086,-10.851069827455,-10.1321597128207),
 .UNSPECIFIED.);
#406=B_SPLINE_CURVE_WITH_KNOTS('',3,(#28467,#28468,#28469,#28470,#28471,
#28472,#28473,#28474,#28475,#28476,#28477,#28478,#28479),.UNSPECIFIED.,
 .F.,.F.,(4,3,3,3,4),(-3.84897440564114,-2.95938268021501,-1.97292178681001,
-0.986460893405001,0.),.UNSPECIFIED.);
#407=B_SPLINE_CURVE_WITH_KNOTS('',3,(#28482,#28483,#28484,#28485,#28486,
#28487,#28488,#28489,#28490,#28491,#28492,#28493,#28494,#28495,#28496,#28497,
#28498,#28499,#28500),.UNSPECIFIED.,.F.,.F.,(4,3,3,3,3,3,4),(2.01694489302845,
2.95938268021501,3.94584357362001,4.93230446702501,5.91876536043001,6.90522625383501,
7.59274844815667),.UNSPECIFIED.);
#408=B_SPLINE_CURVE_WITH_KNOTS('',3,(#28506,#28507,#28508,#28509),
 .UNSPECIFIED.,.F.,.F.,(4,4),(51.5750455984138,52.2824273504652),
 .UNSPECIFIED.);
#409=B_SPLINE_CURVE_WITH_KNOTS('',3,(#28512,#28513,#28514,#28515,#28516,
#28517,#28518,#28519,#28520,#28521),.UNSPECIFIED.,.F.,.F.,(4,3,3,4),(-50.2654824574367,
-49.3230446702501,-48.3365837768451,-47.8312715558982),.UNSPECIFIED.);
#410=B_SPLINE_CURVE_WITH_KNOTS('',3,(#28526,#28527,#28528,#28529,#28530,
#28531,#28532,#28533,#28534,#28535,#28536,#28537,#28538,#28539,#28540,#28541,
#28542,#28543,#28544,#28545,#28546,#28547,#28548,#28549,#28550),
 .UNSPECIFIED.,.F.,.F.,(4,3,3,3,3,3,3,3,4),(45.2918602912342,45.3772010966301,
46.3636619900351,47.3501228834401,48.3365837768451,49.3230446702501,50.3095055636552,
51.2959664570602,51.5750455984138),.UNSPECIFIED.);
#411=B_SPLINE_CURVE_WITH_KNOTS('',3,(#28551,#28552,#28553,#28554,#28555,
#28556,#28557,#28558,#28559,#28560,#28561,#28562,#28563,#28564,#28565,#28566,
#28567,#28568,#28569,#28570,#28571,#28572),.UNSPECIFIED.,.F.,.F.,(4,3,3,
3,3,3,3,4),(-47.8312715558982,-47.3501228834401,-46.3636619900351,-45.3772010966301,
-44.3907402032251,-43.4042793098201,-42.4178184164151,-41.5480862487187),
 .UNSPECIFIED.);
#412=B_SPLINE_CURVE_WITH_KNOTS('',3,(#28577,#28578,#28579,#28580,#28581,
#28582,#28583,#28584,#28585,#28586,#28587,#28588,#28589,#28590,#28591,#28592,
#28593,#28594,#28595,#28596,#28597,#28598),.UNSPECIFIED.,.F.,.F.,(4,3,3,
3,3,3,3,4),(39.0086749840546,39.4584357362001,40.4448966296051,41.4313575230101,
42.4178184164151,43.4042793098201,44.3907402032251,45.2918602912342),
 .UNSPECIFIED.);
#413=B_SPLINE_CURVE_WITH_KNOTS('',3,(#28599,#28600,#28601,#28602,#28603,
#28604,#28605,#28606,#28607,#28608,#28609,#28610,#28611,#28612,#28613,#28614,
#28615,#28616,#28617,#28618,#28619,#28620,#28621,#28622,#28623),
 .UNSPECIFIED.,.F.,.F.,(4,3,3,3,3,3,3,3,4),(-41.5480862487187,-41.4313575230101,
-40.4448966296051,-39.4584357362001,-38.4719748427951,-37.4855139493901,
-36.4990530559851,-35.5125921625801,-35.2649009415391),.UNSPECIFIED.);
#414=B_SPLINE_CURVE_WITH_KNOTS('',3,(#28628,#28629,#28630,#28631,#28632,
#28633,#28634,#28635,#28636,#28637,#28638,#28639,#28640,#28641,#28642,#28643,
#28644,#28645,#28646,#28647,#28648,#28649),.UNSPECIFIED.,.F.,.F.,(4,3,3,
3,3,3,3,4),(32.725489676875,33.5396703757701,34.5261312691751,35.5125921625801,
36.4990530559851,37.4855139493901,38.4719748427951,39.0086749840546),
 .UNSPECIFIED.);
#415=B_SPLINE_CURVE_WITH_KNOTS('',3,(#28650,#28651,#28652,#28653,#28654,
#28655,#28656,#28657,#28658,#28659,#28660,#28661,#28662,#28663,#28664,#28665,
#28666,#28667,#28668,#28669,#28670,#28671),.UNSPECIFIED.,.F.,.F.,(4,3,3,
3,3,3,3,4),(-35.2649009415391,-34.5261312691751,-33.5396703757701,-32.5532094823651,
-31.5667485889601,-30.5802876955551,-29.5938268021501,-28.9817156343595),
 .UNSPECIFIED.);
#416=B_SPLINE_CURVE_WITH_KNOTS('',3,(#28676,#28677,#28678,#28679,#28680,
#28681,#28682,#28683,#28684,#28685,#28686,#28687,#28688,#28689,#28690,#28691,
#28692,#28693,#28694,#28695,#28696,#28697,#28698,#28699,#28700),
 .UNSPECIFIED.,.F.,.F.,(4,3,3,3,3,3,3,3,4),(26.4423043696954,26.6344441219351,
27.6209050153401,28.6073659087451,29.5938268021501,30.5802876955551,31.5667485889601,
32.5532094823651,32.725489676875),.UNSPECIFIED.);
#417=B_SPLINE_CURVE_WITH_KNOTS('',3,(#28701,#28702,#28703,#28704,#28705,
#28706,#28707,#28708,#28709,#28710,#28711,#28712,#28713,#28714,#28715,#28716,
#28717,#28718,#28719,#28720,#28721,#28722),.UNSPECIFIED.,.F.,.F.,(4,3,3,
3,3,3,3,4),(-28.9817156343595,-28.6073659087451,-27.6209050153401,-26.6344441219351,
-25.6479832285301,-24.6615223351251,-23.6750614417201,-22.6985303271799),
 .UNSPECIFIED.);
#418=B_SPLINE_CURVE_WITH_KNOTS('',3,(#28727,#28728,#28729,#28730,#28731,
#28732,#28733,#28734,#28735,#28736,#28737,#28738,#28739,#28740,#28741,#28742,
#28743,#28744,#28745,#28746,#28747,#28748),.UNSPECIFIED.,.F.,.F.,(4,3,3,
3,3,3,3,4),(20.1591190625158,20.7156787615051,21.7021396549101,22.6886005483151,
23.6750614417201,24.6615223351251,25.6479832285301,26.4423043696954),
 .UNSPECIFIED.);
#419=B_SPLINE_CURVE_WITH_KNOTS('',3,(#28749,#28750,#28751,#28752,#28753,
#28754,#28755,#28756,#28757,#28758,#28759,#28760,#28761,#28762,#28763,#28764,
#28765,#28766,#28767,#28768,#28769,#28770,#28771,#28772,#28773),
 .UNSPECIFIED.,.F.,.F.,(4,3,3,3,3,3,3,3,4),(-22.6985303271799,-22.6886005483151,
-21.7021396549101,-20.715678761505,-19.7292178681001,-18.742756974695,-17.75629608129,
-16.769835187885,-16.4153450200003),.UNSPECIFIED.);
#420=B_SPLINE_CURVE_WITH_KNOTS('',3,(#28778,#28779,#28780,#28781,#28782,
#28783,#28784,#28785,#28786,#28787,#28788,#28789,#28790,#28791,#28792,#28793,
#28794,#28795,#28796,#28797,#28798,#28799),.UNSPECIFIED.,.F.,.F.,(4,3,3,
3,3,3,3,4),(13.8759337553363,14.796913401075,15.78337429448,16.7698351878851,
17.7562960812901,18.7427569746951,19.7292178681001,20.1591190625158),
 .UNSPECIFIED.);
#421=B_SPLINE_CURVE_WITH_KNOTS('',3,(#28800,#28801,#28802,#28803,#28804,
#28805,#28806,#28807,#28808,#28809,#28810,#28811,#28812,#28813,#28814,#28815,
#28816,#28817,#28818,#28819,#28820,#28821),.UNSPECIFIED.,.F.,.F.,(4,3,3,
3,3,3,3,4),(-16.4153450200003,-15.78337429448,-14.796913401075,-13.81045250767,
-12.823991614265,-11.83753072086,-10.851069827455,-10.1321597128207),
 .UNSPECIFIED.);
#422=B_SPLINE_CURVE_WITH_KNOTS('',3,(#28827,#28828,#28829,#28830,#28831,
#28832,#28833,#28834,#28835,#28836,#28837,#28838,#28839),.UNSPECIFIED.,
 .F.,.F.,(4,3,3,3,4),(-3.84897440564114,-2.95938268021501,-1.97292178681001,
-0.986460893405004,0.),.UNSPECIFIED.);
#423=B_SPLINE_CURVE_WITH_KNOTS('',3,(#28842,#28843,#28844,#28845,#28846,
#28847,#28848,#28849,#28850,#28851,#28852,#28853,#28854,#28855,#28856,#28857,
#28858,#28859,#28860),.UNSPECIFIED.,.F.,.F.,(4,3,3,3,3,3,4),(2.01694489302844,
2.95938268021501,3.94584357362001,4.93230446702501,5.91876536043001,6.90522625383502,
7.59274844815667),.UNSPECIFIED.);
#424=B_SPLINE_CURVE_WITH_KNOTS('',3,(#28866,#28867,#28868,#28869),
 .UNSPECIFIED.,.F.,.F.,(4,4),(51.5750455984138,52.2824273504652),
 .UNSPECIFIED.);
#425=B_SPLINE_CURVE_WITH_KNOTS('',3,(#28872,#28873,#28874,#28875,#28876,
#28877,#28878,#28879,#28880,#28881),.UNSPECIFIED.,.F.,.F.,(4,3,3,4),(-50.2654824574367,
-49.3230446702501,-48.3365837768451,-47.8312715558983),.UNSPECIFIED.);
#426=B_SPLINE_CURVE_WITH_KNOTS('',3,(#28886,#28887,#28888,#28889,#28890,
#28891,#28892,#28893,#28894,#28895,#28896,#28897,#28898,#28899,#28900,#28901,
#28902,#28903,#28904,#28905,#28906,#28907,#28908,#28909,#28910),
 .UNSPECIFIED.,.F.,.F.,(4,3,3,3,3,3,3,3,4),(45.2918602912342,45.3772010966301,
46.3636619900351,47.3501228834401,48.3365837768452,49.3230446702501,50.3095055636552,
51.2959664570602,51.5750455984138),.UNSPECIFIED.);
#427=B_SPLINE_CURVE_WITH_KNOTS('',3,(#28911,#28912,#28913,#28914,#28915,
#28916,#28917,#28918,#28919,#28920,#28921,#28922,#28923,#28924,#28925,#28926,
#28927,#28928,#28929,#28930,#28931,#28932),.UNSPECIFIED.,.F.,.F.,(4,3,3,
3,3,3,3,4),(-47.8312715558983,-47.3501228834401,-46.3636619900351,-45.3772010966301,
-44.3907402032251,-43.4042793098201,-42.4178184164151,-41.5480862487187),
 .UNSPECIFIED.);
#428=B_SPLINE_CURVE_WITH_KNOTS('',3,(#28937,#28938,#28939,#28940,#28941,
#28942,#28943,#28944,#28945,#28946,#28947,#28948,#28949,#28950,#28951,#28952,
#28953,#28954,#28955,#28956,#28957,#28958),.UNSPECIFIED.,.F.,.F.,(4,3,3,
3,3,3,3,4),(39.0086749840546,39.4584357362001,40.4448966296051,41.4313575230101,
42.4178184164151,43.4042793098201,44.3907402032251,45.2918602912342),
 .UNSPECIFIED.);
#429=B_SPLINE_CURVE_WITH_KNOTS('',3,(#28959,#28960,#28961,#28962,#28963,
#28964,#28965,#28966,#28967,#28968,#28969,#28970,#28971,#28972,#28973,#28974,
#28975,#28976,#28977,#28978,#28979,#28980,#28981,#28982,#28983),
 .UNSPECIFIED.,.F.,.F.,(4,3,3,3,3,3,3,3,4),(-41.5480862487187,-41.4313575230101,
-40.4448966296051,-39.4584357362001,-38.4719748427951,-37.4855139493901,
-36.4990530559851,-35.5125921625801,-35.2649009415391),.UNSPECIFIED.);
#430=B_SPLINE_CURVE_WITH_KNOTS('',3,(#28988,#28989,#28990,#28991,#28992,
#28993,#28994,#28995,#28996,#28997,#28998,#28999,#29000,#29001,#29002,#29003,
#29004,#29005,#29006,#29007,#29008,#29009),.UNSPECIFIED.,.F.,.F.,(4,3,3,
3,3,3,3,4),(32.725489676875,33.5396703757701,34.5261312691751,35.5125921625801,
36.4990530559851,37.4855139493901,38.4719748427951,39.0086749840546),
 .UNSPECIFIED.);
#431=B_SPLINE_CURVE_WITH_KNOTS('',3,(#29010,#29011,#29012,#29013,#29014,
#29015,#29016,#29017,#29018,#29019,#29020,#29021,#29022,#29023,#29024,#29025,
#29026,#29027,#29028,#29029,#29030,#29031),.UNSPECIFIED.,.F.,.F.,(4,3,3,
3,3,3,3,4),(-35.2649009415391,-34.5261312691751,-33.5396703757701,-32.5532094823651,
-31.5667485889601,-30.5802876955551,-29.5938268021501,-28.9817156343595),
 .UNSPECIFIED.);
#432=B_SPLINE_CURVE_WITH_KNOTS('',3,(#29036,#29037,#29038,#29039,#29040,
#29041,#29042,#29043,#29044,#29045,#29046,#29047,#29048,#29049,#29050,#29051,
#29052,#29053,#29054,#29055,#29056,#29057,#29058,#29059,#29060),
 .UNSPECIFIED.,.F.,.F.,(4,3,3,3,3,3,3,3,4),(26.4423043696954,26.6344441219351,
27.6209050153401,28.6073659087451,29.5938268021501,30.5802876955551,31.5667485889601,
32.5532094823651,32.725489676875),.UNSPECIFIED.);
#433=B_SPLINE_CURVE_WITH_KNOTS('',3,(#29061,#29062,#29063,#29064,#29065,
#29066,#29067,#29068,#29069,#29070,#29071,#29072,#29073,#29074,#29075,#29076,
#29077,#29078,#29079,#29080,#29081,#29082),.UNSPECIFIED.,.F.,.F.,(4,3,3,
3,3,3,3,4),(-28.9817156343595,-28.6073659087451,-27.6209050153401,-26.6344441219351,
-25.6479832285301,-24.6615223351251,-23.6750614417201,-22.6985303271799),
 .UNSPECIFIED.);
#434=B_SPLINE_CURVE_WITH_KNOTS('',3,(#29087,#29088,#29089,#29090,#29091,
#29092,#29093,#29094,#29095,#29096,#29097,#29098,#29099,#29100,#29101,#29102,
#29103,#29104,#29105,#29106,#29107,#29108),.UNSPECIFIED.,.F.,.F.,(4,3,3,
3,3,3,3,4),(20.1591190625159,20.7156787615051,21.7021396549101,22.6886005483151,
23.6750614417201,24.6615223351251,25.6479832285301,26.4423043696954),
 .UNSPECIFIED.);
#435=B_SPLINE_CURVE_WITH_KNOTS('',3,(#29109,#29110,#29111,#29112,#29113,
#29114,#29115,#29116,#29117,#29118,#29119,#29120,#29121,#29122,#29123,#29124,
#29125,#29126,#29127,#29128,#29129,#29130,#29131,#29132,#29133),
 .UNSPECIFIED.,.F.,.F.,(4,3,3,3,3,3,3,3,4),(-22.6985303271799,-22.6886005483151,
-21.7021396549101,-20.7156787615051,-19.7292178681001,-18.7427569746951,
-17.7562960812901,-16.7698351878851,-16.4153450200003),.UNSPECIFIED.);
#436=B_SPLINE_CURVE_WITH_KNOTS('',3,(#29138,#29139,#29140,#29141,#29142,
#29143,#29144,#29145,#29146,#29147,#29148,#29149,#29150,#29151,#29152,#29153,
#29154,#29155,#29156,#29157,#29158,#29159),.UNSPECIFIED.,.F.,.F.,(4,3,3,
3,3,3,3,4),(13.8759337553363,14.7969134010751,15.78337429448,16.7698351878851,
17.75629608129,18.7427569746951,19.7292178681001,20.1591190625159),
 .UNSPECIFIED.);
#437=B_SPLINE_CURVE_WITH_KNOTS('',3,(#29160,#29161,#29162,#29163,#29164,
#29165,#29166,#29167,#29168,#29169,#29170,#29171,#29172,#29173,#29174,#29175,
#29176,#29177,#29178,#29179,#29180,#29181),.UNSPECIFIED.,.F.,.F.,(4,3,3,
3,3,3,3,4),(-16.4153450200003,-15.78337429448,-14.796913401075,-13.81045250767,
-12.823991614265,-11.83753072086,-10.851069827455,-10.1321597128207),
 .UNSPECIFIED.);
#438=B_SPLINE_CURVE_WITH_KNOTS('',3,(#29187,#29188,#29189,#29190,#29191,
#29192,#29193,#29194,#29195,#29196,#29197,#29198,#29199),.UNSPECIFIED.,
 .F.,.F.,(4,3,3,3,4),(-3.84897440564115,-2.95938268021501,-1.97292178681001,
-0.986460893405001,0.),.UNSPECIFIED.);
#439=B_SPLINE_CURVE_WITH_KNOTS('',3,(#29202,#29203,#29204,#29205,#29206,
#29207,#29208,#29209,#29210,#29211,#29212,#29213,#29214,#29215,#29216,#29217,
#29218,#29219,#29220),.UNSPECIFIED.,.F.,.F.,(4,3,3,3,3,3,4),(2.01694489302845,
2.95938268021501,3.94584357362001,4.93230446702501,5.91876536043001,6.90522625383502,
7.59274844815668),.UNSPECIFIED.);
#440=B_SPLINE_CURVE_WITH_KNOTS('',3,(#29226,#29227,#29228,#29229,#29230,
#29231,#29232,#29233),.UNSPECIFIED.,.F.,.F.,(4,1,1,1,1,4),(59.6902604182061,
60.1955726391529,61.1820335325579,62.1684944259629,63.154955319368,64.141416212773),
 .UNSPECIFIED.);
#441=B_SPLINE_CURVE_WITH_KNOTS('',3,(#29236,#29237,#29238,#29239,#29240,
#29241,#29242,#29243,#29244),.UNSPECIFIED.,.F.,.F.,(4,1,1,1,1,1,4),(59.6902604182061,
59.775601223602,60.762062117007,61.748523010412,62.734983903817,63.721444797222,
64.6638825844085),.UNSPECIFIED.);
#442=B_SPLINE_CURVE_WITH_KNOTS('',3,(#29249,#29250,#29251,#29252,#29253,
#29254,#29255,#29256,#29257,#29258),.UNSPECIFIED.,.F.,.F.,(4,1,1,1,1,1,
1,4),(53.4070751110265,54.2768072787229,55.2632681721279,56.2497290655329,
57.2361899589379,58.2226508523429,59.2091117457479,59.6902604182061),
 .UNSPECIFIED.);
#443=B_SPLINE_CURVE_WITH_KNOTS('',3,(#29259,#29260,#29261,#29262,#29263,
#29264,#29265,#29266,#29267,#29268),.UNSPECIFIED.,.F.,.F.,(4,1,1,1,1,1,
1,4),(53.4070751110265,53.856835863172,54.843296756577,55.829757649982,
56.816218543387,57.802679436792,58.789140330197,59.6902604182061),
 .UNSPECIFIED.);
#444=B_SPLINE_CURVE_WITH_KNOTS('',3,(#29273,#29274,#29275,#29276,#29277,
#29278,#29279,#29280,#29281,#29282,#29283),.UNSPECIFIED.,.F.,.F.,(4,1,1,
1,1,1,1,1,4),(47.1238898038469,47.3715810248879,48.3580419182929,49.3445028116979,
50.3309637051029,51.3174245985079,52.3038854919129,53.2903463853179,53.4070751110265),
 .UNSPECIFIED.);
#445=B_SPLINE_CURVE_WITH_KNOTS('',3,(#29284,#29285,#29286,#29287,#29288,
#29289,#29290,#29291,#29292,#29293),.UNSPECIFIED.,.F.,.F.,(4,1,1,1,1,1,
1,4),(47.1238898038469,47.9380705027419,48.9245313961469,49.9109922895519,
50.8974531829569,51.8839140763619,52.8703749697669,53.4070751110265),
 .UNSPECIFIED.);
#446=B_SPLINE_CURVE_WITH_KNOTS('',3,(#29298,#29299,#29300,#29301,#29302,
#29303,#29304,#29305,#29306,#29307),.UNSPECIFIED.,.F.,.F.,(4,1,1,1,1,1,
1,4),(40.8407044966673,41.4528156644579,42.4392765578629,43.4257374512679,
44.4121983446729,45.3986592380779,46.3851201314829,47.1238898038469),
 .UNSPECIFIED.);
#447=B_SPLINE_CURVE_WITH_KNOTS('',3,(#29308,#29309,#29310,#29311,#29312,
#29313,#29314,#29315,#29316,#29317,#29318),.UNSPECIFIED.,.F.,.F.,(4,1,1,
1,1,1,1,1,4),(40.8407044966673,41.0328442489069,42.0193051423119,43.0057660357169,
43.9922269291219,44.9786878225269,45.9651487159319,46.9516096093369,47.1238898038469),
 .UNSPECIFIED.);
#448=B_SPLINE_CURVE_WITH_KNOTS('',3,(#29323,#29324,#29325,#29326,#29327,
#29328,#29329,#29330,#29331,#29332),.UNSPECIFIED.,.F.,.F.,(4,1,1,1,1,1,
1,4),(34.5575191894877,35.5340503040279,36.5205111974329,37.5069720908379,
38.4934329842429,39.4798938776479,40.4663547710529,40.8407044966673),
 .UNSPECIFIED.);
#449=B_SPLINE_CURVE_WITH_KNOTS('',3,(#29333,#29334,#29335,#29336,#29337,
#29338,#29339,#29340,#29341,#29342),.UNSPECIFIED.,.F.,.F.,(4,1,1,1,1,1,
1,4),(34.5575191894877,35.1140788884769,36.1005397818819,37.0870006752869,
38.0734615686919,39.0599224620969,40.0463833555019,40.8407044966673),
 .UNSPECIFIED.);
#450=B_SPLINE_CURVE_WITH_KNOTS('',3,(#29347,#29348,#29349,#29350,#29351,
#29352,#29353,#29354,#29355,#29356,#29357),.UNSPECIFIED.,.F.,.F.,(4,1,1,
1,1,1,1,1,4),(28.2743338823081,28.6288240501929,29.6152849435979,30.6017458370029,
31.5882067304079,32.5746676238129,33.5611285172179,34.5475894106229,34.5575191894877),
 .UNSPECIFIED.);
#451=B_SPLINE_CURVE_WITH_KNOTS('',3,(#29358,#29359,#29360,#29361,#29362,
#29363,#29364,#29365,#29366,#29367),.UNSPECIFIED.,.F.,.F.,(4,1,1,1,1,1,
1,4),(28.2743338823081,29.1953135280469,30.1817744214519,31.1682353148569,
32.1546962082619,33.1411571016669,34.1276179950719,34.5575191894877),
 .UNSPECIFIED.);
#452=B_SPLINE_CURVE_WITH_KNOTS('',3,(#29372,#29373,#29374,#29375,#29376,
#29377,#29378,#29379,#29380,#29381),.UNSPECIFIED.,.F.,.F.,(4,1,1,1,1,1,
1,4),(21.9911485751285,22.7100586897628,23.6965195831678,24.6829804765728,
25.6694413699778,26.6559022633828,27.6423631567879,28.2743338823081),
 .UNSPECIFIED.);
#453=B_SPLINE_CURVE_WITH_KNOTS('',3,(#29382,#29383,#29384,#29385,#29386,
#29387,#29388,#29389,#29390,#29391,#29392),.UNSPECIFIED.,.F.,.F.,(4,1,1,
1,1,1,1,1,4),(21.9911485751285,22.2900872742119,23.2765481676169,24.2630090610219,
25.2494699544269,26.2359308478319,27.2223917412369,28.2088526346419,28.2743338823081),
 .UNSPECIFIED.);
#454=B_SPLINE_CURVE_WITH_KNOTS('',3,(#29398,#29399,#29400,#29401,#29402),
 .UNSPECIFIED.,.F.,.F.,(4,1,4),(14.3984001269718,15.3848610203768,15.7079632679489),
 .UNSPECIFIED.);
#455=B_SPLINE_CURVE_WITH_KNOTS('',3,(#29405,#29406,#29407,#29408,#29409),
 .UNSPECIFIED.,.F.,.F.,(4,1,4),(13.8759337553363,14.8183715425228,15.7079632679489),
 .UNSPECIFIED.);
#456=B_SPLINE_CURVE_WITH_KNOTS('',3,(#29415,#29416,#29417,#29418,#29419,
#29420,#29421,#29422),.UNSPECIFIED.,.F.,.F.,(4,1,1,1,1,4),(59.6902604182061,
60.1955726391529,61.1820335325579,62.1684944259629,63.1549553193679,64.1414162127729),
 .UNSPECIFIED.);
#457=B_SPLINE_CURVE_WITH_KNOTS('',3,(#29425,#29426,#29427,#29428,#29429,
#29430,#29431,#29432,#29433),.UNSPECIFIED.,.F.,.F.,(4,1,1,1,1,1,4),(59.6902604182061,
59.775601223602,60.762062117007,61.748523010412,62.734983903817,63.721444797222,
64.6638825844085),.UNSPECIFIED.);
#458=B_SPLINE_CURVE_WITH_KNOTS('',3,(#29438,#29439,#29440,#29441,#29442,
#29443,#29444,#29445,#29446,#29447),.UNSPECIFIED.,.F.,.F.,(4,1,1,1,1,1,
1,4),(53.4070751110265,54.2768072787229,55.2632681721279,56.2497290655329,
57.2361899589379,58.2226508523429,59.2091117457479,59.6902604182061),
 .UNSPECIFIED.);
#459=B_SPLINE_CURVE_WITH_KNOTS('',3,(#29448,#29449,#29450,#29451,#29452,
#29453,#29454,#29455,#29456,#29457),.UNSPECIFIED.,.F.,.F.,(4,1,1,1,1,1,
1,4),(53.4070751110265,53.856835863172,54.843296756577,55.829757649982,
56.816218543387,57.802679436792,58.789140330197,59.6902604182061),
 .UNSPECIFIED.);
#460=B_SPLINE_CURVE_WITH_KNOTS('',3,(#29462,#29463,#29464,#29465,#29466,
#29467,#29468,#29469,#29470,#29471,#29472),.UNSPECIFIED.,.F.,.F.,(4,1,1,
1,1,1,1,1,4),(47.1238898038469,47.3715810248879,48.3580419182929,49.3445028116979,
50.3309637051029,51.3174245985079,52.3038854919129,53.2903463853179,53.4070751110265),
 .UNSPECIFIED.);
#461=B_SPLINE_CURVE_WITH_KNOTS('',3,(#29473,#29474,#29475,#29476,#29477,
#29478,#29479,#29480,#29481,#29482),.UNSPECIFIED.,.F.,.F.,(4,1,1,1,1,1,
1,4),(47.1238898038469,47.9380705027419,48.9245313961469,49.9109922895519,
50.8974531829569,51.8839140763619,52.8703749697669,53.4070751110265),
 .UNSPECIFIED.);
#462=B_SPLINE_CURVE_WITH_KNOTS('',3,(#29487,#29488,#29489,#29490,#29491,
#29492,#29493,#29494,#29495,#29496),.UNSPECIFIED.,.F.,.F.,(4,1,1,1,1,1,
1,4),(40.8407044966673,41.4528156644579,42.4392765578629,43.4257374512679,
44.4121983446729,45.3986592380779,46.3851201314829,47.1238898038469),
 .UNSPECIFIED.);
#463=B_SPLINE_CURVE_WITH_KNOTS('',3,(#29497,#29498,#29499,#29500,#29501,
#29502,#29503,#29504,#29505,#29506,#29507),.UNSPECIFIED.,.F.,.F.,(4,1,1,
1,1,1,1,1,4),(40.8407044966673,41.0328442489069,42.0193051423119,43.0057660357169,
43.9922269291219,44.9786878225269,45.9651487159319,46.9516096093369,47.1238898038469),
 .UNSPECIFIED.);
#464=B_SPLINE_CURVE_WITH_KNOTS('',3,(#29512,#29513,#29514,#29515,#29516,
#29517,#29518,#29519,#29520,#29521),.UNSPECIFIED.,.F.,.F.,(4,1,1,1,1,1,
1,4),(34.5575191894877,35.5340503040279,36.5205111974329,37.5069720908379,
38.4934329842429,39.4798938776479,40.4663547710529,40.8407044966673),
 .UNSPECIFIED.);
#465=B_SPLINE_CURVE_WITH_KNOTS('',3,(#29522,#29523,#29524,#29525,#29526,
#29527,#29528,#29529,#29530,#29531),.UNSPECIFIED.,.F.,.F.,(4,1,1,1,1,1,
1,4),(34.5575191894877,35.1140788884769,36.1005397818819,37.0870006752869,
38.0734615686919,39.0599224620969,40.0463833555019,40.8407044966673),
 .UNSPECIFIED.);
#466=B_SPLINE_CURVE_WITH_KNOTS('',3,(#29536,#29537,#29538,#29539,#29540,
#29541,#29542,#29543,#29544,#29545,#29546),.UNSPECIFIED.,.F.,.F.,(4,1,1,
1,1,1,1,1,4),(28.2743338823081,28.6288240501928,29.6152849435978,30.6017458370028,
31.5882067304078,32.5746676238129,33.5611285172179,34.5475894106229,34.5575191894877),
 .UNSPECIFIED.);
#467=B_SPLINE_CURVE_WITH_KNOTS('',3,(#29547,#29548,#29549,#29550,#29551,
#29552,#29553,#29554,#29555,#29556),.UNSPECIFIED.,.F.,.F.,(4,1,1,1,1,1,
1,4),(28.2743338823081,29.1953135280469,30.1817744214519,31.1682353148569,
32.1546962082619,33.1411571016669,34.1276179950719,34.5575191894877),
 .UNSPECIFIED.);
#468=B_SPLINE_CURVE_WITH_KNOTS('',3,(#29561,#29562,#29563,#29564,#29565,
#29566,#29567,#29568,#29569,#29570),.UNSPECIFIED.,.F.,.F.,(4,1,1,1,1,1,
1,4),(21.9911485751285,22.7100586897628,23.6965195831678,24.6829804765728,
25.6694413699778,26.6559022633828,27.6423631567878,28.2743338823081),
 .UNSPECIFIED.);
#469=B_SPLINE_CURVE_WITH_KNOTS('',3,(#29571,#29572,#29573,#29574,#29575,
#29576,#29577,#29578,#29579,#29580,#29581),.UNSPECIFIED.,.F.,.F.,(4,1,1,
1,1,1,1,1,4),(21.9911485751285,22.2900872742119,23.2765481676169,24.2630090610219,
25.2494699544269,26.2359308478319,27.2223917412369,28.2088526346419,28.2743338823081),
 .UNSPECIFIED.);
#470=B_SPLINE_CURVE_WITH_KNOTS('',3,(#29587,#29588,#29589,#29590,#29591),
 .UNSPECIFIED.,.F.,.F.,(4,1,4),(14.3984001269718,15.3848610203768,15.7079632679489),
 .UNSPECIFIED.);
#471=B_SPLINE_CURVE_WITH_KNOTS('',3,(#29594,#29595,#29596,#29597,#29598),
 .UNSPECIFIED.,.F.,.F.,(4,1,4),(13.8759337553362,14.8183715425228,15.707963267949),
 .UNSPECIFIED.);
#472=B_SPLINE_CURVE_WITH_KNOTS('',3,(#29604,#29605,#29606,#29607,#29608,
#29609,#29610,#29611),.UNSPECIFIED.,.F.,.F.,(4,1,1,1,1,4),(59.6902604182061,
60.1955726391529,61.1820335325579,62.1684944259629,63.154955319368,64.141416212773),
 .UNSPECIFIED.);
#473=B_SPLINE_CURVE_WITH_KNOTS('',3,(#29614,#29615,#29616,#29617,#29618,
#29619,#29620,#29621,#29622),.UNSPECIFIED.,.F.,.F.,(4,1,1,1,1,1,4),(59.6902604182061,
59.775601223602,60.762062117007,61.748523010412,62.734983903817,63.721444797222,
64.6638825844085),.UNSPECIFIED.);
#474=B_SPLINE_CURVE_WITH_KNOTS('',3,(#29627,#29628,#29629,#29630,#29631,
#29632,#29633,#29634,#29635,#29636),.UNSPECIFIED.,.F.,.F.,(4,1,1,1,1,1,
1,4),(53.4070751110265,54.2768072787229,55.2632681721279,56.2497290655329,
57.2361899589379,58.2226508523429,59.2091117457479,59.6902604182061),
 .UNSPECIFIED.);
#475=B_SPLINE_CURVE_WITH_KNOTS('',3,(#29637,#29638,#29639,#29640,#29641,
#29642,#29643,#29644,#29645,#29646),.UNSPECIFIED.,.F.,.F.,(4,1,1,1,1,1,
1,4),(53.4070751110265,53.856835863172,54.843296756577,55.829757649982,
56.816218543387,57.802679436792,58.789140330197,59.6902604182061),
 .UNSPECIFIED.);
#476=B_SPLINE_CURVE_WITH_KNOTS('',3,(#29651,#29652,#29653,#29654,#29655,
#29656,#29657,#29658,#29659,#29660,#29661),.UNSPECIFIED.,.F.,.F.,(4,1,1,
1,1,1,1,1,4),(47.1238898038469,47.3715810248879,48.3580419182929,49.3445028116979,
50.3309637051029,51.3174245985079,52.3038854919129,53.2903463853179,53.4070751110265),
 .UNSPECIFIED.);
#477=B_SPLINE_CURVE_WITH_KNOTS('',3,(#29662,#29663,#29664,#29665,#29666,
#29667,#29668,#29669,#29670,#29671),.UNSPECIFIED.,.F.,.F.,(4,1,1,1,1,1,
1,4),(47.1238898038469,47.9380705027419,48.9245313961469,49.9109922895519,
50.8974531829569,51.8839140763619,52.8703749697669,53.4070751110265),
 .UNSPECIFIED.);
#478=B_SPLINE_CURVE_WITH_KNOTS('',3,(#29676,#29677,#29678,#29679,#29680,
#29681,#29682,#29683,#29684,#29685),.UNSPECIFIED.,.F.,.F.,(4,1,1,1,1,1,
1,4),(40.8407044966673,41.4528156644579,42.4392765578629,43.4257374512679,
44.4121983446729,45.3986592380779,46.3851201314829,47.1238898038469),
 .UNSPECIFIED.);
#479=B_SPLINE_CURVE_WITH_KNOTS('',3,(#29686,#29687,#29688,#29689,#29690,
#29691,#29692,#29693,#29694,#29695,#29696),.UNSPECIFIED.,.F.,.F.,(4,1,1,
1,1,1,1,1,4),(40.8407044966673,41.0328442489069,42.0193051423119,43.0057660357169,
43.9922269291219,44.9786878225269,45.9651487159319,46.9516096093369,47.1238898038469),
 .UNSPECIFIED.);
#480=B_SPLINE_CURVE_WITH_KNOTS('',3,(#29701,#29702,#29703,#29704,#29705,
#29706,#29707,#29708,#29709,#29710),.UNSPECIFIED.,.F.,.F.,(4,1,1,1,1,1,
1,4),(34.5575191894877,35.5340503040279,36.5205111974329,37.5069720908379,
38.4934329842429,39.4798938776479,40.4663547710529,40.8407044966673),
 .UNSPECIFIED.);
#481=B_SPLINE_CURVE_WITH_KNOTS('',3,(#29711,#29712,#29713,#29714,#29715,
#29716,#29717,#29718,#29719,#29720),.UNSPECIFIED.,.F.,.F.,(4,1,1,1,1,1,
1,4),(34.5575191894877,35.1140788884769,36.1005397818819,37.0870006752869,
38.0734615686919,39.0599224620969,40.0463833555019,40.8407044966673),
 .UNSPECIFIED.);
#482=B_SPLINE_CURVE_WITH_KNOTS('',3,(#29725,#29726,#29727,#29728,#29729,
#29730,#29731,#29732,#29733,#29734,#29735),.UNSPECIFIED.,.F.,.F.,(4,1,1,
1,1,1,1,1,4),(28.2743338823081,28.6288240501929,29.6152849435979,30.6017458370029,
31.5882067304079,32.5746676238129,33.5611285172179,34.5475894106229,34.5575191894877),
 .UNSPECIFIED.);
#483=B_SPLINE_CURVE_WITH_KNOTS('',3,(#29736,#29737,#29738,#29739,#29740,
#29741,#29742,#29743,#29744,#29745),.UNSPECIFIED.,.F.,.F.,(4,1,1,1,1,1,
1,4),(28.2743338823081,29.1953135280469,30.1817744214519,31.1682353148569,
32.1546962082619,33.1411571016669,34.1276179950719,34.5575191894877),
 .UNSPECIFIED.);
#484=B_SPLINE_CURVE_WITH_KNOTS('',3,(#29750,#29751,#29752,#29753,#29754,
#29755,#29756,#29757,#29758,#29759),.UNSPECIFIED.,.F.,.F.,(4,1,1,1,1,1,
1,4),(21.9911485751285,22.7100586897628,23.6965195831678,24.6829804765728,
25.6694413699778,26.6559022633828,27.6423631567879,28.2743338823081),
 .UNSPECIFIED.);
#485=B_SPLINE_CURVE_WITH_KNOTS('',3,(#29760,#29761,#29762,#29763,#29764,
#29765,#29766,#29767,#29768,#29769,#29770),.UNSPECIFIED.,.F.,.F.,(4,1,1,
1,1,1,1,1,4),(21.9911485751285,22.2900872742119,23.2765481676169,24.2630090610219,
25.2494699544269,26.2359308478319,27.2223917412369,28.2088526346419,28.2743338823081),
 .UNSPECIFIED.);
#486=B_SPLINE_CURVE_WITH_KNOTS('',3,(#29776,#29777,#29778,#29779,#29780),
 .UNSPECIFIED.,.F.,.F.,(4,1,4),(14.3984001269718,15.3848610203768,15.7079632679489),
 .UNSPECIFIED.);
#487=B_SPLINE_CURVE_WITH_KNOTS('',3,(#29783,#29784,#29785,#29786,#29787),
 .UNSPECIFIED.,.F.,.F.,(4,1,4),(13.8759337553363,14.8183715425228,15.707963267949),
 .UNSPECIFIED.);
#488=B_SPLINE_CURVE_WITH_KNOTS('',3,(#29793,#29794,#29795,#29796,#29797,
#29798,#29799,#29800),.UNSPECIFIED.,.F.,.F.,(4,1,1,1,1,4),(59.6902604182061,
60.1955726391529,61.1820335325579,62.1684944259629,63.1549553193679,64.1414162127729),
 .UNSPECIFIED.);
#489=B_SPLINE_CURVE_WITH_KNOTS('',3,(#29803,#29804,#29805,#29806,#29807,
#29808,#29809,#29810,#29811),.UNSPECIFIED.,.F.,.F.,(4,1,1,1,1,1,4),(59.6902604182061,
59.775601223602,60.762062117007,61.748523010412,62.734983903817,63.721444797222,
64.6638825844085),.UNSPECIFIED.);
#490=B_SPLINE_CURVE_WITH_KNOTS('',3,(#29816,#29817,#29818,#29819,#29820,
#29821,#29822,#29823,#29824,#29825),.UNSPECIFIED.,.F.,.F.,(4,1,1,1,1,1,
1,4),(53.4070751110265,54.2768072787229,55.2632681721279,56.2497290655329,
57.2361899589379,58.2226508523429,59.2091117457479,59.6902604182061),
 .UNSPECIFIED.);
#491=B_SPLINE_CURVE_WITH_KNOTS('',3,(#29826,#29827,#29828,#29829,#29830,
#29831,#29832,#29833,#29834,#29835),.UNSPECIFIED.,.F.,.F.,(4,1,1,1,1,1,
1,4),(53.4070751110265,53.856835863172,54.843296756577,55.829757649982,
56.816218543387,57.802679436792,58.789140330197,59.6902604182061),
 .UNSPECIFIED.);
#492=B_SPLINE_CURVE_WITH_KNOTS('',3,(#29840,#29841,#29842,#29843,#29844,
#29845,#29846,#29847,#29848,#29849,#29850),.UNSPECIFIED.,.F.,.F.,(4,1,1,
1,1,1,1,1,4),(47.1238898038469,47.3715810248879,48.3580419182929,49.3445028116979,
50.3309637051029,51.3174245985079,52.3038854919129,53.2903463853179,53.4070751110265),
 .UNSPECIFIED.);
#493=B_SPLINE_CURVE_WITH_KNOTS('',3,(#29851,#29852,#29853,#29854,#29855,
#29856,#29857,#29858,#29859,#29860),.UNSPECIFIED.,.F.,.F.,(4,1,1,1,1,1,
1,4),(47.1238898038469,47.9380705027419,48.9245313961469,49.9109922895519,
50.8974531829569,51.8839140763619,52.8703749697669,53.4070751110265),
 .UNSPECIFIED.);
#494=B_SPLINE_CURVE_WITH_KNOTS('',3,(#29865,#29866,#29867,#29868,#29869,
#29870,#29871,#29872,#29873,#29874),.UNSPECIFIED.,.F.,.F.,(4,1,1,1,1,1,
1,4),(40.8407044966673,41.4528156644579,42.4392765578629,43.4257374512679,
44.4121983446729,45.3986592380779,46.3851201314829,47.1238898038469),
 .UNSPECIFIED.);
#495=B_SPLINE_CURVE_WITH_KNOTS('',3,(#29875,#29876,#29877,#29878,#29879,
#29880,#29881,#29882,#29883,#29884,#29885),.UNSPECIFIED.,.F.,.F.,(4,1,1,
1,1,1,1,1,4),(40.8407044966673,41.0328442489069,42.0193051423119,43.0057660357169,
43.9922269291219,44.9786878225269,45.9651487159319,46.9516096093369,47.1238898038469),
 .UNSPECIFIED.);
#496=B_SPLINE_CURVE_WITH_KNOTS('',3,(#29890,#29891,#29892,#29893,#29894,
#29895,#29896,#29897,#29898,#29899),.UNSPECIFIED.,.F.,.F.,(4,1,1,1,1,1,
1,4),(34.5575191894877,35.5340503040279,36.5205111974329,37.5069720908379,
38.4934329842429,39.4798938776479,40.4663547710529,40.8407044966673),
 .UNSPECIFIED.);
#497=B_SPLINE_CURVE_WITH_KNOTS('',3,(#29900,#29901,#29902,#29903,#29904,
#29905,#29906,#29907,#29908,#29909),.UNSPECIFIED.,.F.,.F.,(4,1,1,1,1,1,
1,4),(34.5575191894877,35.1140788884769,36.1005397818819,37.0870006752869,
38.0734615686919,39.0599224620969,40.0463833555019,40.8407044966673),
 .UNSPECIFIED.);
#498=B_SPLINE_CURVE_WITH_KNOTS('',3,(#29914,#29915,#29916,#29917,#29918,
#29919,#29920,#29921,#29922,#29923,#29924),.UNSPECIFIED.,.F.,.F.,(4,1,1,
1,1,1,1,1,4),(28.2743338823081,28.6288240501928,29.6152849435978,30.6017458370028,
31.5882067304078,32.5746676238129,33.5611285172179,34.5475894106229,34.5575191894877),
 .UNSPECIFIED.);
#499=B_SPLINE_CURVE_WITH_KNOTS('',3,(#29925,#29926,#29927,#29928,#29929,
#29930,#29931,#29932,#29933,#29934),.UNSPECIFIED.,.F.,.F.,(4,1,1,1,1,1,
1,4),(28.2743338823081,29.1953135280469,30.1817744214519,31.1682353148569,
32.1546962082619,33.1411571016669,34.1276179950719,34.5575191894877),
 .UNSPECIFIED.);
#500=B_SPLINE_CURVE_WITH_KNOTS('',3,(#29939,#29940,#29941,#29942,#29943,
#29944,#29945,#29946,#29947,#29948),.UNSPECIFIED.,.F.,.F.,(4,1,1,1,1,1,
1,4),(21.9911485751285,22.7100586897628,23.6965195831678,24.6829804765728,
25.6694413699778,26.6559022633828,27.6423631567878,28.2743338823081),
 .UNSPECIFIED.);
#501=B_SPLINE_CURVE_WITH_KNOTS('',3,(#29949,#29950,#29951,#29952,#29953,
#29954,#29955,#29956,#29957,#29958,#29959),.UNSPECIFIED.,.F.,.F.,(4,1,1,
1,1,1,1,1,4),(21.9911485751285,22.2900872742119,23.2765481676169,24.2630090610219,
25.2494699544269,26.2359308478319,27.2223917412369,28.2088526346419,28.2743338823081),
 .UNSPECIFIED.);
#502=B_SPLINE_CURVE_WITH_KNOTS('',3,(#29965,#29966,#29967,#29968,#29969),
 .UNSPECIFIED.,.F.,.F.,(4,1,4),(14.3984001269718,15.3848610203768,15.7079632679489),
 .UNSPECIFIED.);
#503=B_SPLINE_CURVE_WITH_KNOTS('',3,(#29972,#29973,#29974,#29975,#29976),
 .UNSPECIFIED.,.F.,.F.,(4,1,4),(13.8759337553362,14.8183715425228,15.707963267949),
 .UNSPECIFIED.);
#504=B_SPLINE_CURVE_WITH_KNOTS('',3,(#29978,#29979,#29980,#29981,#29982,
#29983,#29984,#29985,#29986,#29987,#29988),.UNSPECIFIED.,.F.,.F.,(4,1,1,
1,1,1,1,1,4),(15.707963267949,15.8048324359278,16.7912933293328,17.7777542227378,
18.7642151161428,19.7506760095478,20.7371369029528,21.7235977963578,21.9911485751285),
 .UNSPECIFIED.);
#505=B_SPLINE_CURVE_WITH_KNOTS('',3,(#29989,#29990,#29991,#29992,#29993,
#29994,#29995,#29996,#29997,#29998),.UNSPECIFIED.,.F.,.F.,(4,1,1,1,1,1,
1,4),(15.7079632679489,16.3713219137818,17.3577828071868,18.3442437005918,
19.3307045939968,20.3171654874019,21.3036263808069,21.9911485751285),
 .UNSPECIFIED.);
#506=B_SPLINE_CURVE_WITH_KNOTS('',3,(#30223,#30224,#30225,#30226,#30227,
#30228,#30229,#30230,#30231,#30232,#30233,#30234,#30235,#30236,#30237,#30238,
#30239,#30240,#30241,#30242,#30243,#30244,#30245,#30246,#30247,#30248,#30249,
#30250,#30251,#30252,#30253,#30254,#30255,#30256,#30257,#30258,#30259,#30260,
#30261,#30262,#30263,#30264,#30265,#30266,#30267,#30268,#30269,#30270,#30271,
#30272,#30273,#30274,#30275,#30276,#30277,#30278,#30279,#30280,#30281,#30282,
#30283,#30284,#30285,#30286,#30287,#30288,#30289,#30290,#30291,#30292,#30293,
#30294,#30295,#30296,#30297,#30298,#30299,#30300,#30301,#30302,#30303,#30304,
#30305,#30306,#30307,#30308,#30309,#30310,#30311,#30312,#30313,#30314,#30315,
#30316,#30317,#30318,#30319),.UNSPECIFIED.,.F.,.F.,(4,3,3,3,3,3,3,3,3,3,
3,3,3,3,3,3,3,3,3,3,3,3,3,3,3,3,3,3,3,3,3,3,4),(0.,0.0368039558979425,0.074433304608195,
0.113993701727663,0.148609049207197,0.155428774052918,0.160415086629183,
0.19765208124705,0.234804500431717,0.271449068097489,0.301315921464101,
0.308903275242872,0.314301747825082,0.350380426672586,0.385744311753463,
0.390916481563936,0.427339708778546,0.447829010848363,0.457282933923372,
0.462717602197838,0.49927396966006,0.535072007005015,0.570520291726377,
0.593601322997532,0.601390754314479,0.606406537654944,0.641366377472567,
0.669816918578329,0.683592881655056,0.691680493901417,0.725189682307058,
0.755168541895614,0.770777738583641),.UNSPECIFIED.);
#507=B_SPLINE_CURVE_WITH_KNOTS('',3,(#30320,#30321,#30322,#30323,#30324,
#30325,#30326,#30327,#30328,#30329,#30330,#30331,#30332,#30333,#30334,#30335,
#30336,#30337,#30338,#30339,#30340,#30341,#30342,#30343,#30344,#30345,#30346,
#30347,#30348,#30349,#30350,#30351,#30352,#30353,#30354,#30355,#30356,#30357,
#30358,#30359,#30360,#30361,#30362,#30363,#30364,#30365,#30366,#30367,#30368,
#30369,#30370,#30371,#30372,#30373,#30374,#30375,#30376,#30377,#30378,#30379,
#30380,#30381,#30382,#30383,#30384,#30385,#30386,#30387,#30388,#30389,#30390,
#30391,#30392,#30393,#30394,#30395,#30396,#30397,#30398,#30399,#30400,#30401,
#30402,#30403,#30404,#30405,#30406,#30407,#30408,#30409,#30410,#30411,#30412,
#30413),.UNSPECIFIED.,.F.,.F.,(4,3,3,3,3,3,3,3,3,3,3,3,3,3,3,3,3,3,3,3,
3,3,3,3,3,3,3,3,3,3,3,4),(0.,0.0327224441775746,0.0662804107708102,0.100536831058394,
0.133256562666979,0.138568566128973,0.143645838996043,0.178633774293771,
0.214080648720454,0.251134157522108,0.278924289123348,0.285558989031475,
0.321777080052277,0.357762779229756,0.362294683927068,0.397656599693718,
0.419708620040541,0.427245869011975,0.432639317722629,0.468078758515067,
0.504737423019667,0.541741021670041,0.567834509616647,0.5794821004587,0.584482028048437,
0.622064205916635,0.6541703857482,0.668577115889702,0.678363311229139,0.716158211242659,
0.750488925242892,0.768398079192695),.UNSPECIFIED.);
#508=B_SPLINE_CURVE_WITH_KNOTS('',3,(#30414,#30415,#30416,#30417,#30418,
#30419,#30420,#30421,#30422,#30423,#30424,#30425,#30426,#30427,#30428,#30429,
#30430,#30431,#30432,#30433,#30434,#30435,#30436,#30437,#30438),
 .UNSPECIFIED.,.F.,.F.,(4,3,3,3,3,3,3,3,4),(-10.1321597128207,-9.86460893405003,
-8.87814804064502,-7.89168714724003,-6.90522625383502,-5.91876536043002,
-4.93230446702502,-3.94584357362001,-3.84897440564115),.UNSPECIFIED.);
#509=B_SPLINE_CURVE_WITH_KNOTS('',3,(#30663,#30664,#30665,#30666,#30667,
#30668,#30669,#30670,#30671,#30672,#30673,#30674,#30675,#30676,#30677,#30678,
#30679,#30680,#30681,#30682,#30683,#30684,#30685,#30686,#30687,#30688,#30689,
#30690,#30691,#30692,#30693,#30694,#30695,#30696,#30697,#30698,#30699,#30700,
#30701,#30702,#30703,#30704,#30705,#30706,#30707,#30708,#30709,#30710,#30711,
#30712,#30713,#30714,#30715,#30716,#30717,#30718,#30719,#30720,#30721,#30722,
#30723,#30724,#30725,#30726,#30727,#30728,#30729,#30730,#30731,#30732,#30733,
#30734,#30735,#30736,#30737,#30738,#30739,#30740,#30741,#30742,#30743,#30744,
#30745,#30746,#30747,#30748,#30749,#30750,#30751,#30752,#30753,#30754,#30755,
#30756),.UNSPECIFIED.,.F.,.F.,(4,3,3,3,3,3,3,3,3,3,3,3,3,3,3,3,3,3,3,3,
3,3,3,3,3,3,3,3,3,3,3,4),(0.,0.0327225492804934,0.0662806081929849,0.100537094180834,
0.133256792899112,0.138569651942616,0.143645965484312,0.178633966005382,
0.214080867277344,0.251134321439773,0.278924412061594,0.285558992744241,
0.321777089637378,0.35776275463403,0.362294683927058,0.397656555534726,
0.419708578641487,0.427246439006672,0.432639234997264,0.468078611004923,
0.504737248356826,0.541740841146129,0.567834351658225,0.579481449773753,
0.584481041781399,0.622063204762494,0.654169634882595,0.668576564062872,
0.678363413635591,0.716158311359956,0.750488925242897,0.768398079192707),
 .UNSPECIFIED.);
#510=B_SPLINE_CURVE_WITH_KNOTS('',3,(#30757,#30758,#30759,#30760,#30761,
#30762,#30763,#30764,#30765,#30766,#30767,#30768,#30769,#30770,#30771,#30772,
#30773,#30774,#30775,#30776,#30777,#30778,#30779,#30780,#30781),
 .UNSPECIFIED.,.F.,.F.,(4,3,3,3,3,3,3,3,4),(7.59274844815668,7.89168714724002,
8.87814804064503,9.86460893405003,10.851069827455,11.83753072086,12.823991614265,
13.81045250767,13.8759337553363),.UNSPECIFIED.);
#511=B_SPLINE_CURVE_WITH_KNOTS('',3,(#30782,#30783,#30784,#30785,#30786,
#30787,#30788,#30789,#30790,#30791,#30792,#30793,#30794,#30795,#30796,#30797,
#30798,#30799,#30800,#30801,#30802,#30803,#30804,#30805,#30806,#30807,#30808,
#30809,#30810,#30811,#30812,#30813,#30814,#30815,#30816,#30817,#30818,#30819,
#30820,#30821,#30822,#30823,#30824,#30825,#30826,#30827,#30828,#30829,#30830,
#30831,#30832,#30833,#30834,#30835,#30836,#30837,#30838,#30839,#30840,#30841,
#30842,#30843,#30844,#30845,#30846,#30847,#30848,#30849,#30850,#30851,#30852,
#30853,#30854,#30855,#30856,#30857,#30858,#30859,#30860,#30861,#30862,#30863,
#30864,#30865,#30866,#30867,#30868,#30869,#30870,#30871,#30872,#30873,#30874,
#30875,#30876,#30877,#30878),.UNSPECIFIED.,.F.,.F.,(4,3,3,3,3,3,3,3,3,3,
3,3,3,3,3,3,3,3,3,3,3,3,3,3,3,3,3,3,3,3,3,3,4),(0.,0.036804046830165,0.0744334499110545,
0.113993828867664,0.148609160454698,0.155429461366191,0.160415755364031,
0.197652761113477,0.234805154528782,0.271449678901402,0.301316379567035,
0.30890483519103,0.314302031357973,0.350380678677425,0.385744531292533,
0.390916481563933,0.427339707871941,0.447829009998422,0.457282914861488,
0.462717597114684,0.499273965212302,0.535072004716797,0.570520279377824,
0.59360131219255,0.601390713399489,0.606406454642536,0.641366288894707,
0.669816852144937,0.683592817141769,0.691680484574319,0.72518963603372,
0.75516854189563,0.77077773858366),.UNSPECIFIED.);
#512=B_SPLINE_CURVE_WITH_KNOTS('',3,(#30888,#30889,#30890,#30891,#30892,
#30893,#30894,#30895,#30896,#30897,#30898,#30899,#30900,#30901,#30902,#30903,
#30904,#30905,#30906,#30907,#30908,#30909,#30910,#30911,#30912,#30913,#30914,
#30915,#30916,#30917,#30918,#30919,#30920,#30921,#30922,#30923,#30924,#30925,
#30926,#30927,#30928,#30929,#30930,#30931,#30932,#30933,#30934,#30935,#30936,
#30937,#30938,#30939,#30940,#30941,#30942,#30943,#30944,#30945,#30946,#30947,
#30948,#30949,#30950,#30951,#30952,#30953,#30954,#30955,#30956,#30957,#30958,
#30959,#30960,#30961,#30962,#30963,#30964,#30965,#30966,#30967,#30968,#30969,
#30970,#30971,#30972,#30973,#30974,#30975,#30976,#30977,#30978,#30979,#30980,
#30981),.UNSPECIFIED.,.F.,.F.,(4,3,3,3,3,3,3,3,3,3,3,3,3,3,3,3,3,3,3,3,
3,3,3,3,3,3,3,3,3,3,3,4),(0.,0.032722467477059,0.0662804545367435,0.10053688939052,
0.133256613707586,0.138568806761047,0.143645866999149,0.178633816756561,
0.214080697136686,0.251134193834276,0.278924316357469,0.285558989874725,
0.321777082201843,0.35776277380543,0.362294683927046,0.397656589907163,
0.419708610865643,0.427245995316486,0.432639299360784,0.468078725795143,
0.504737384281388,0.54174098163239,0.567834474583697,0.579481956142016,
0.584481809181592,0.622063983748247,0.654170219121896,0.668576993434055,
0.678363333947687,0.716158233455664,0.750488925242844,0.768398079192646),
 .UNSPECIFIED.);
#513=B_SPLINE_CURVE_WITH_KNOTS('',3,(#30982,#30983,#30984,#30985,#30986,
#30987,#30988,#30989,#30990,#30991,#30992,#30993,#30994,#30995,#30996,#30997,
#30998,#30999,#31000,#31001,#31002,#31003,#31004,#31005,#31006,#31007,#31008,
#31009,#31010,#31011,#31012,#31013,#31014,#31015,#31016,#31017,#31018,#31019,
#31020,#31021,#31022,#31023,#31024,#31025,#31026,#31027,#31028,#31029,#31030,
#31031,#31032,#31033,#31034,#31035,#31036,#31037,#31038,#31039,#31040,#31041,
#31042,#31043,#31044,#31045,#31046,#31047,#31048,#31049,#31050,#31051,#31052,
#31053,#31054,#31055,#31056,#31057,#31058,#31059,#31060,#31061,#31062,#31063,
#31064,#31065,#31066,#31067,#31068,#31069,#31070,#31071,#31072,#31073,#31074,
#31075,#31076,#31077,#31078),.UNSPECIFIED.,.F.,.F.,(4,3,3,3,3,3,3,3,3,3,
3,3,3,3,3,3,3,3,3,3,3,3,3,3,3,3,3,3,3,3,3,3,4),(0.,0.0368040733914109,0.0744334923513577,
0.113993866002931,0.148609192948057,0.155429662167008,0.160415950914505,
0.197652959912295,0.23480534579311,0.271449857509325,0.301316513522979,
0.308905291482282,0.314302114409216,0.350380752512021,0.385744595636286,
0.390916481563942,0.427339707606562,0.447829009749629,0.457282909273663,
0.462717595625807,0.499273963909537,0.53507200404104,0.57052027575377,0.593601309021504,
0.60139070143526,0.60640643038342,0.641366263001721,0.669816832725203,0.683592798284754,
0.691680481858046,0.725189622506651,0.755168541895646,0.770777738583679),
 .UNSPECIFIED.);
#514=B_SPLINE_CURVE_WITH_KNOTS('',3,(#31079,#31080,#31081,#31082,#31083,
#31084,#31085,#31086,#31087,#31088,#31089,#31090,#31091,#31092,#31093,#31094,
#31095,#31096,#31097,#31098,#31099,#31100,#31101,#31102,#31103,#31104,#31105,
#31106,#31107,#31108,#31109,#31110,#31111,#31112,#31113,#31114,#31115,#31116,
#31117,#31118,#31119,#31120,#31121,#31122,#31123,#31124,#31125,#31126,#31127,
#31128,#31129,#31130,#31131,#31132,#31133,#31134,#31135,#31136,#31137,#31138,
#31139,#31140,#31141,#31142,#31143,#31144,#31145,#31146,#31147,#31148,#31149,
#31150,#31151,#31152,#31153,#31154,#31155,#31156,#31157,#31158,#31159,#31160,
#31161,#31162,#31163,#31164,#31165,#31166,#31167,#31168,#31169,#31170,#31171,
#31172),.UNSPECIFIED.,.F.,.F.,(4,3,3,3,3,3,3,3,3,3,3,3,3,3,3,3,3,3,3,3,
3,3,3,3,3,3,3,3,3,3,3,4),(0.,0.0327224959120641,0.0662805079475318,0.100536960576692,
0.133256675995489,0.138569100515552,0.143645901206212,0.1786338686101,0.214080756253453,
0.251134238171856,0.278924349610658,0.285558990870915,0.321777084786821,
0.35776276714434,0.362294683927063,0.39765657796237,0.419708599667403,0.427246149485785,
0.432639276975905,0.468078685886249,0.504737337027106,0.541740932792406,
0.567834431848717,0.579481780097231,0.584481542244862,0.622063712786212,
0.654170015900382,0.6685768440841,0.678363361689231,0.716158260579035,0.750488925242892,
0.768398079192696),.UNSPECIFIED.);
#515=B_SPLINE_CURVE_WITH_KNOTS('',3,(#31173,#31174,#31175,#31176,#31177,
#31178,#31179,#31180,#31181,#31182,#31183,#31184,#31185,#31186,#31187,#31188,
#31189,#31190,#31191,#31192,#31193,#31194,#31195,#31196,#31197,#31198,#31199,
#31200,#31201,#31202,#31203,#31204,#31205,#31206,#31207,#31208,#31209,#31210,
#31211,#31212,#31213,#31214,#31215,#31216,#31217,#31218,#31219,#31220,#31221,
#31222,#31223,#31224,#31225,#31226,#31227,#31228,#31229,#31230,#31231,#31232,
#31233,#31234,#31235,#31236,#31237,#31238,#31239,#31240,#31241,#31242,#31243,
#31244,#31245,#31246,#31247,#31248,#31249,#31250,#31251,#31252,#31253,#31254,
#31255,#31256,#31257,#31258,#31259,#31260,#31261,#31262,#31263,#31264,#31265,
#31266,#31267,#31268,#31269),.UNSPECIFIED.,.F.,.F.,(4,3,3,3,3,3,3,3,3,3,
3,3,3,3,3,3,3,3,3,3,3,3,3,3,3,3,3,3,3,3,3,3,4),(0.,0.0368039914157241,0.0744333613634087,
0.113993751388472,0.148609092660403,0.155429042492168,0.160415347695229,
0.197652346662473,0.234804755786334,0.271449306551343,0.301316100304487,
0.308903884150417,0.314301858425386,0.350380524963378,0.385744397367857,
0.390916481563918,0.427339708424226,0.447829010516186,0.457282926489124,
0.462717600214839,0.499273967924932,0.53507200611566,0.570520286913965,
0.593601318786667,0.601390738323114,0.606406505217338,0.64136634286951,
0.669816892626028,0.683592856456032,0.691680490247784,0.725189664234744,
0.75516854189558,0.770777738583609),.UNSPECIFIED.);
#516=B_SPLINE_CURVE_WITH_KNOTS('',3,(#31270,#31271,#31272,#31273,#31274,
#31275,#31276,#31277,#31278,#31279,#31280,#31281,#31282,#31283,#31284,#31285,
#31286,#31287,#31288,#31289,#31290,#31291,#31292,#31293,#31294,#31295,#31296,
#31297,#31298,#31299,#31300,#31301,#31302,#31303,#31304,#31305,#31306,#31307,
#31308,#31309,#31310,#31311,#31312,#31313,#31314,#31315,#31316,#31317,#31318,
#31319,#31320,#31321,#31322,#31323,#31324,#31325,#31326,#31327,#31328,#31329,
#31330,#31331,#31332,#31333,#31334,#31335,#31336,#31337,#31338,#31339,#31340,
#31341,#31342,#31343,#31344,#31345,#31346,#31347,#31348,#31349,#31350,#31351,
#31352,#31353,#31354,#31355,#31356,#31357,#31358,#31359,#31360,#31361,#31362,
#31363),.UNSPECIFIED.,.F.,.F.,(4,3,3,3,3,3,3,3,3,3,3,3,3,3,3,3,3,3,3,3,
3,3,3,3,3,3,3,3,3,3,3,4),(0.,0.0327225294770781,0.0662805709960721,0.100537044605592,
0.133256749520777,0.138569447222746,0.143645941610917,0.17863392984422,
0.214080826059521,0.251134290526409,0.278924388876575,0.285558992053491,
0.321777087844177,0.357762759284444,0.362294683927074,0.397656563857957,
0.419708586444518,0.427246331524387,0.432639250564409,0.468078638783316,
0.50473728125208,0.541740875145429,0.567834381407617,0.579481572313244,
0.584481227357561,0.622063393148413,0.654169776172043,0.668576667903374,
0.678363394448717,0.71615829260595,0.750488925242933,0.768398079192735),
 .UNSPECIFIED.);
#517=B_SPLINE_CURVE_WITH_KNOTS('',3,(#31364,#31365,#31366,#31367,#31368,
#31369,#31370,#31371,#31372,#31373,#31374,#31375,#31376,#31377,#31378,#31379,
#31380,#31381,#31382,#31383,#31384,#31385,#31386,#31387,#31388,#31389,#31390,
#31391,#31392,#31393,#31394,#31395,#31396,#31397,#31398,#31399,#31400,#31401,
#31402,#31403,#31404,#31405,#31406,#31407,#31408,#31409,#31410,#31411,#31412,
#31413,#31414,#31415,#31416,#31417,#31418,#31419,#31420,#31421,#31422,#31423,
#31424,#31425,#31426,#31427,#31428,#31429,#31430,#31431,#31432,#31433,#31434,
#31435,#31436,#31437,#31438,#31439,#31440,#31441,#31442,#31443,#31444,#31445,
#31446,#31447,#31448,#31449,#31450,#31451,#31452,#31453,#31454,#31455,#31456,
#31457,#31458,#31459,#31460),.UNSPECIFIED.,.F.,.F.,(4,3,3,3,3,3,3,3,3,3,
3,3,3,3,3,3,3,3,3,3,3,3,3,3,3,3,3,3,3,3,3,3,4),(0.,0.0368040169038835,0.0744334020924358,
0.11399378702637,0.148609123843563,0.155429235171562,0.160415535189551,
0.197652537277058,0.234804939176668,0.271449477805488,0.301316228745094,
0.308904321525207,0.31430193792665,0.350380595626898,0.385744458930709,
0.390916481563911,0.427339708170469,0.447829010278287,0.45728292112946,
0.462717598788197,0.499273966676618,0.535072005472898,0.570520283450759,
0.593601315756361,0.601390726866048,0.606406481970154,0.641366318060403,
0.669816874019195,0.683592838382448,0.691680487645043,0.725189651274617,
0.75516854189557,0.770777738583599),.UNSPECIFIED.);
#518=B_SPLINE_CURVE_WITH_KNOTS('',3,(#31462,#31463,#31464,#31465,#31466,
#31467,#31468,#31469,#31470,#31471,#31472),.UNSPECIFIED.,.F.,.F.,(4,1,1,
1,1,1,1,1,4),(15.707963267949,15.8048324359278,16.7912933293328,17.7777542227378,
18.7642151161428,19.7506760095478,20.7371369029528,21.7235977963578,21.9911485751285),
 .UNSPECIFIED.);
#519=B_SPLINE_CURVE_WITH_KNOTS('',3,(#31473,#31474,#31475,#31476,#31477,
#31478,#31479,#31480,#31481,#31482),.UNSPECIFIED.,.F.,.F.,(4,1,1,1,1,1,
1,4),(15.7079632679489,16.3713219137818,17.3577828071869,18.3442437005919,
19.3307045939969,20.3171654874019,21.3036263808069,21.9911485751285),
 .UNSPECIFIED.);
#520=B_SPLINE_CURVE_WITH_KNOTS('',3,(#31707,#31708,#31709,#31710,#31711,
#31712,#31713,#31714,#31715,#31716,#31717,#31718,#31719,#31720,#31721,#31722,
#31723,#31724,#31725,#31726,#31727,#31728,#31729,#31730,#31731,#31732,#31733,
#31734,#31735,#31736,#31737,#31738,#31739,#31740,#31741,#31742,#31743,#31744,
#31745,#31746,#31747,#31748,#31749,#31750,#31751,#31752,#31753,#31754,#31755,
#31756,#31757,#31758,#31759,#31760,#31761,#31762,#31763,#31764,#31765,#31766,
#31767,#31768,#31769,#31770,#31771,#31772,#31773,#31774,#31775,#31776,#31777,
#31778,#31779,#31780,#31781,#31782,#31783,#31784,#31785,#31786,#31787,#31788,
#31789,#31790,#31791,#31792,#31793,#31794,#31795,#31796,#31797,#31798,#31799,
#31800,#31801,#31802,#31803),.UNSPECIFIED.,.F.,.F.,(4,3,3,3,3,3,3,3,3,3,
3,3,3,3,3,3,3,3,3,3,3,3,3,3,3,3,3,3,3,3,3,3,4),(0.,0.0368040006584821,0.0744333761311954,
0.113993764310286,0.14860910396699,0.155429112383965,0.160415415803185,
0.19765241590165,0.234804822404722,0.27144936877189,0.301316146969897,0.308904043046986,
0.314301887301155,0.350380550636825,0.385744419741531,0.39091648156392,
0.427339708332513,0.447829010430206,0.45728292453119,0.462717599696291,
0.499273967471206,0.535072005882051,0.570520285658179,0.593601317687859,
0.601390734201157,0.60640649698701,0.641366334082055,0.669816886035445,
0.683592850009941,0.691680489272535,0.725189659504915,0.755168541895614,
0.770777738583643),.UNSPECIFIED.);
#521=B_SPLINE_CURVE_WITH_KNOTS('',3,(#31804,#31805,#31806,#31807,#31808,
#31809,#31810,#31811,#31812,#31813,#31814,#31815,#31816,#31817,#31818,#31819,
#31820,#31821,#31822,#31823,#31824,#31825,#31826,#31827,#31828),
 .UNSPECIFIED.,.F.,.F.,(4,3,3,3,3,3,3,3,4),(-10.1321597128207,-9.86460893405003,
-8.87814804064502,-7.89168714724002,-6.90522625383502,-5.91876536043002,
-4.93230446702501,-3.94584357362001,-3.84897440564114),.UNSPECIFIED.);
#522=B_SPLINE_CURVE_WITH_KNOTS('',3,(#32053,#32054,#32055,#32056,#32057,
#32058,#32059,#32060,#32061,#32062,#32063,#32064,#32065,#32066,#32067,#32068,
#32069,#32070,#32071,#32072,#32073,#32074,#32075,#32076,#32077,#32078,#32079,
#32080,#32081,#32082,#32083,#32084,#32085,#32086,#32087,#32088,#32089,#32090,
#32091,#32092,#32093,#32094,#32095,#32096,#32097,#32098,#32099,#32100,#32101,
#32102,#32103,#32104,#32105,#32106,#32107,#32108,#32109,#32110,#32111,#32112,
#32113,#32114,#32115,#32116,#32117,#32118,#32119,#32120,#32121,#32122,#32123,
#32124,#32125,#32126,#32127,#32128,#32129,#32130,#32131,#32132,#32133,#32134,
#32135,#32136,#32137,#32138,#32139,#32140,#32141,#32142,#32143,#32144,#32145,
#32146),.UNSPECIFIED.,.F.,.F.,(4,3,3,3,3,3,3,3,3,3,3,3,3,3,3,3,3,3,3,3,
3,3,3,3,3,3,3,3,3,3,3,4),(0.,0.0327224852298601,0.0662804878799529,0.100536933829056,
0.133256652591307,0.138568990289855,0.143645888367285,0.178633849142766,
0.214080734056413,0.251134221524075,0.278924337124821,0.285558990484342,
0.321777083808023,0.357762769641534,0.362294683927059,0.397656582449134,
0.419708603873742,0.427246091593913,0.432639285230977,0.468078700718258,
0.504737354615871,0.541740950976496,0.567834447759792,0.579481845655055,
0.584481641657808,0.62206381370368,0.654170091588477,0.668576899729838,
0.678363351333556,0.716158250454694,0.750488925242868,0.768398079192674),
 .UNSPECIFIED.);
#523=B_SPLINE_CURVE_WITH_KNOTS('',3,(#32147,#32148,#32149,#32150,#32151,
#32152,#32153,#32154,#32155,#32156,#32157,#32158,#32159,#32160,#32161,#32162,
#32163,#32164,#32165,#32166,#32167,#32168,#32169,#32170,#32171),
 .UNSPECIFIED.,.F.,.F.,(4,3,3,3,3,3,3,3,4),(7.59274844815667,7.89168714724002,
8.87814804064502,9.86460893405003,10.851069827455,11.83753072086,12.823991614265,
13.81045250767,13.8759337553363),.UNSPECIFIED.);
#524=B_SPLINE_CURVE_WITH_KNOTS('',3,(#32173,#32174,#32175,#32176,#32177,
#32178,#32179,#32180,#32181,#32182,#32183),.UNSPECIFIED.,.F.,.F.,(4,1,1,
1,1,1,1,1,4),(15.707963267949,15.8048324359278,16.7912933293328,17.7777542227378,
18.7642151161428,19.7506760095478,20.7371369029528,21.7235977963578,21.9911485751285),
 .UNSPECIFIED.);
#525=B_SPLINE_CURVE_WITH_KNOTS('',3,(#32184,#32185,#32186,#32187,#32188,
#32189,#32190,#32191,#32192,#32193),.UNSPECIFIED.,.F.,.F.,(4,1,1,1,1,1,
1,4),(15.7079632679489,16.3713219137818,17.3577828071868,18.3442437005918,
19.3307045939968,20.3171654874019,21.3036263808069,21.9911485751285),
 .UNSPECIFIED.);
#526=B_SPLINE_CURVE_WITH_KNOTS('',3,(#32418,#32419,#32420,#32421,#32422,
#32423,#32424,#32425,#32426,#32427,#32428,#32429,#32430,#32431,#32432,#32433,
#32434,#32435,#32436,#32437,#32438,#32439,#32440,#32441,#32442,#32443,#32444,
#32445,#32446,#32447,#32448,#32449,#32450,#32451,#32452,#32453,#32454,#32455,
#32456,#32457,#32458,#32459,#32460,#32461,#32462,#32463,#32464,#32465,#32466,
#32467,#32468,#32469,#32470,#32471,#32472,#32473,#32474,#32475,#32476,#32477,
#32478,#32479,#32480,#32481,#32482,#32483,#32484,#32485,#32486,#32487,#32488,
#32489,#32490,#32491,#32492,#32493,#32494,#32495,#32496,#32497,#32498,#32499,
#32500,#32501,#32502,#32503,#32504,#32505,#32506,#32507,#32508,#32509,#32510,
#32511,#32512,#32513,#32514),.UNSPECIFIED.,.F.,.F.,(4,3,3,3,3,3,3,3,3,3,
3,3,3,3,3,3,3,3,3,3,3,3,3,3,3,3,3,3,3,3,3,3,4),(0.,0.0368039760561726,0.0744333368184212,
0.113993729911609,0.148609073868149,0.155428926386467,0.160415234743925,
0.197652231831378,0.234804645306633,0.271449203389433,0.301316022933056,
0.308903620706599,0.314301810562592,0.350380482429235,0.385744360315095,
0.390916481563925,0.427339708572203,0.447829010654916,0.457282929707203,
0.462717601073039,0.49927396867586,0.535072006502099,0.570520288994985,
0.593601320607563,0.601390745293023,0.606406519246091,0.641366357839995,
0.669816903853899,0.683592867357584,0.691680491796103,0.725189672020684,
0.755168541895609,0.770777738583641),.UNSPECIFIED.);
#527=B_SPLINE_CURVE_WITH_KNOTS('',3,(#32515,#32516,#32517,#32518,#32519,
#32520,#32521,#32522,#32523,#32524,#32525,#32526,#32527,#32528,#32529,#32530,
#32531,#32532,#32533,#32534,#32535,#32536,#32537,#32538,#32539),
 .UNSPECIFIED.,.F.,.F.,(4,3,3,3,3,3,3,3,4),(-10.1321597128207,-9.86460893405003,
-8.87814804064502,-7.89168714724003,-6.90522625383502,-5.91876536043002,
-4.93230446702502,-3.94584357362001,-3.84897440564115),.UNSPECIFIED.);
#528=B_SPLINE_CURVE_WITH_KNOTS('',3,(#32764,#32765,#32766,#32767,#32768,
#32769,#32770,#32771,#32772,#32773,#32774,#32775,#32776,#32777,#32778,#32779,
#32780,#32781,#32782,#32783,#32784,#32785,#32786,#32787,#32788,#32789,#32790,
#32791,#32792,#32793,#32794,#32795,#32796,#32797,#32798,#32799,#32800,#32801,
#32802,#32803,#32804,#32805,#32806,#32807,#32808,#32809,#32810,#32811,#32812,
#32813,#32814,#32815,#32816,#32817,#32818,#32819,#32820,#32821,#32822,#32823,
#32824,#32825,#32826,#32827,#32828,#32829,#32830,#32831,#32832,#32833,#32834,
#32835,#32836,#32837,#32838,#32839,#32840,#32841,#32842,#32843,#32844,#32845,
#32846,#32847,#32848,#32849,#32850,#32851,#32852,#32853,#32854,#32855,#32856,
#32857),.UNSPECIFIED.,.F.,.F.,(4,3,3,3,3,3,3,3,3,3,3,3,3,3,3,3,3,3,3,3,
3,3,3,3,3,3,3,3,3,3,3,4),(0.,0.0327225799773267,0.0662806658545984,0.100537171029244,
0.133256860141472,0.138569969050608,0.143646002487887,0.178634022059388,
0.214080931165366,0.251134369355791,0.27892444799861,0.285558993885552,
0.321777092476967,0.357762747477908,0.362294683927068,0.397656542631737,
0.419708566544936,0.427246605750548,0.432639210952107,0.468078568034648,
0.504737197455354,0.541740788532467,0.567834305621274,0.579481260120421,
0.584480754431237,0.622062913075079,0.654169416117039,0.668576403279121,
0.678363443657298,0.716158340709877,0.750488925242921,0.768398079192729),
 .UNSPECIFIED.);
#529=B_SPLINE_CURVE_WITH_KNOTS('',3,(#32858,#32859,#32860,#32861,#32862,
#32863,#32864,#32865,#32866,#32867,#32868,#32869,#32870,#32871,#32872,#32873,
#32874,#32875,#32876,#32877,#32878,#32879,#32880,#32881,#32882),
 .UNSPECIFIED.,.F.,.F.,(4,3,3,3,3,3,3,3,4),(7.59274844815668,7.89168714724002,
8.87814804064503,9.86460893405003,10.851069827455,11.83753072086,12.823991614265,
13.81045250767,13.8759337553363),.UNSPECIFIED.);
#530=B_SPLINE_CURVE_WITH_KNOTS('',3,(#32884,#32885,#32886,#32887,#32888,
#32889,#32890,#32891,#32892,#32893,#32894),.UNSPECIFIED.,.F.,.F.,(4,1,1,
1,1,1,1,1,4),(15.7079632679489,15.8048324359278,16.7912933293328,17.7777542227378,
18.7642151161428,19.7506760095478,20.7371369029528,21.7235977963578,21.9911485751285),
 .UNSPECIFIED.);
#531=B_SPLINE_CURVE_WITH_KNOTS('',3,(#32895,#32896,#32897,#32898,#32899,
#32900,#32901,#32902,#32903,#32904),.UNSPECIFIED.,.F.,.F.,(4,1,1,1,1,1,
1,4),(15.7079632679489,16.3713219137818,17.3577828071869,18.3442437005919,
19.3307045939969,20.3171654874019,21.3036263808069,21.9911485751285),
 .UNSPECIFIED.);
#532=B_SPLINE_CURVE_WITH_KNOTS('',3,(#33129,#33130,#33131,#33132,#33133,
#33134,#33135,#33136,#33137,#33138,#33139,#33140,#33141,#33142,#33143,#33144,
#33145,#33146,#33147,#33148,#33149,#33150,#33151,#33152,#33153,#33154,#33155,
#33156,#33157,#33158,#33159,#33160,#33161,#33162,#33163,#33164,#33165,#33166,
#33167,#33168,#33169,#33170,#33171,#33172,#33173,#33174,#33175,#33176,#33177,
#33178,#33179,#33180,#33181,#33182,#33183,#33184,#33185,#33186,#33187,#33188,
#33189,#33190,#33191,#33192,#33193,#33194,#33195,#33196,#33197,#33198,#33199,
#33200,#33201,#33202,#33203,#33204,#33205,#33206,#33207,#33208,#33209,#33210,
#33211,#33212,#33213,#33214,#33215,#33216,#33217,#33218,#33219,#33220,#33221,
#33222,#33223,#33224,#33225),.UNSPECIFIED.,.F.,.F.,(4,3,3,3,3,3,3,3,3,3,
3,3,3,3,3,3,3,3,3,3,3,3,3,3,3,3,3,3,3,3,3,3,4),(0.,0.0368040296983295,0.0744334225357169,
0.113993804914242,0.148609139495452,0.155429331856321,0.160415629309949,
0.19765263296232,0.234805031233744,0.271449563770314,0.301316293218716,
0.308904541097941,0.314301977856807,0.350380631124549,0.385744489860858,
0.39091648156392,0.427339708037647,0.447829010153769,0.457282918385807,
0.462717598065727,0.499273966044462,0.535072005142963,0.570520281705417,
0.593601314229191,0.601390721049491,0.606406470197016,0.641366305496701,
0.669816864596427,0.6835928292529,0.691680486306265,0.725189644734797,0.755168541895606,
0.770777738583634),.UNSPECIFIED.);
#533=B_SPLINE_CURVE_WITH_KNOTS('',3,(#33226,#33227,#33228,#33229,#33230,
#33231,#33232,#33233,#33234,#33235,#33236,#33237,#33238,#33239,#33240,#33241,
#33242,#33243,#33244,#33245,#33246,#33247,#33248,#33249,#33250),
 .UNSPECIFIED.,.F.,.F.,(4,3,3,3,3,3,3,3,4),(-10.1321597128207,-9.86460893405003,
-8.87814804064502,-7.89168714724002,-6.90522625383502,-5.91876536043002,
-4.93230446702502,-3.94584357362001,-3.84897440564114),.UNSPECIFIED.);
#534=B_SPLINE_CURVE_WITH_KNOTS('',3,(#33475,#33476,#33477,#33478,#33479,
#33480,#33481,#33482,#33483,#33484,#33485,#33486,#33487,#33488,#33489,#33490,
#33491,#33492,#33493,#33494,#33495,#33496,#33497,#33498,#33499,#33500,#33501,
#33502,#33503,#33504,#33505,#33506,#33507,#33508,#33509,#33510,#33511,#33512,
#33513,#33514,#33515,#33516,#33517,#33518,#33519,#33520,#33521,#33522,#33523,
#33524,#33525,#33526,#33527,#33528,#33529,#33530,#33531,#33532,#33533,#33534,
#33535,#33536,#33537,#33538,#33539,#33540,#33541,#33542,#33543,#33544,#33545,
#33546,#33547,#33548,#33549,#33550,#33551,#33552,#33553,#33554,#33555,#33556,
#33557,#33558,#33559,#33560,#33561,#33562,#33563,#33564,#33565,#33566,#33567,
#33568),.UNSPECIFIED.,.F.,.F.,(4,3,3,3,3,3,3,3,3,3,3,3,3,3,3,3,3,3,3,3,
3,3,3,3,3,3,3,3,3,3,3,4),(0.,0.0327225146876364,0.0662805432171355,0.10053700758566,
0.133256717128334,0.138569294358745,0.143645923792125,0.178633902850418,
0.21408079528951,0.251134267448895,0.278924371568434,0.28555899152832,0.321777086502174,
0.357762762756158,0.36229468392705,0.397656570072467,0.419708592270616,
0.427246251204994,0.432639262274467,0.468078659615991,0.504737305906693,
0.541740900625277,0.567834403702473,0.579481664146009,0.584481366534682,
0.622063534445468,0.654169882144813,0.668576745773135,0.678363380045444,
0.716158278526066,0.750488925242846,0.768398079192654),.UNSPECIFIED.);
#535=B_SPLINE_CURVE_WITH_KNOTS('',3,(#33569,#33570,#33571,#33572,#33573,
#33574,#33575,#33576,#33577,#33578,#33579,#33580,#33581,#33582,#33583,#33584,
#33585,#33586,#33587,#33588,#33589,#33590,#33591,#33592,#33593),
 .UNSPECIFIED.,.F.,.F.,(4,3,3,3,3,3,3,3,4),(7.59274844815667,7.89168714724002,
8.87814804064502,9.86460893405002,10.851069827455,11.83753072086,12.823991614265,
13.81045250767,13.8759337553363),.UNSPECIFIED.);
#2214=SHAPE_REPRESENTATION_RELATIONSHIP('SRR','None',#97607,#2233);
#2233=ADVANCED_BREP_SHAPE_REPRESENTATION('',(#2271),#97457);
#2252=STYLED_ITEM('',(#97719),#2271);
#2271=MANIFOLD_SOLID_BREP('Body1',#21813);
#2304=FACE_BOUND('',#3801,.T.);
#2305=FACE_BOUND('',#3802,.T.);
#2306=FACE_BOUND('',#3803,.T.);
#2307=FACE_BOUND('',#3804,.T.);
#2308=FACE_BOUND('',#3823,.T.);
#2309=FACE_BOUND('',#3824,.T.);
#2310=FACE_BOUND('',#3825,.T.);
#2311=FACE_BOUND('',#3826,.T.);
#2399=PLANE('',#22164);
#2400=PLANE('',#22172);
#2401=PLANE('',#22173);
#2402=PLANE('',#22174);
#2403=PLANE('',#22175);
#2404=PLANE('',#22176);
#2563=FACE_OUTER_BOUND('',#3733,.T.);
#2564=FACE_OUTER_BOUND('',#3734,.T.);
#2565=FACE_OUTER_BOUND('',#3735,.T.);
#2566=FACE_OUTER_BOUND('',#3736,.T.);
#2567=FACE_OUTER_BOUND('',#3737,.T.);
#2568=FACE_OUTER_BOUND('',#3738,.T.);
#2569=FACE_OUTER_BOUND('',#3739,.T.);
#2570=FACE_OUTER_BOUND('',#3740,.T.);
#2571=FACE_OUTER_BOUND('',#3741,.T.);
#2572=FACE_OUTER_BOUND('',#3742,.T.);
#2573=FACE_OUTER_BOUND('',#3743,.T.);
#2574=FACE_OUTER_BOUND('',#3744,.T.);
#2575=FACE_OUTER_BOUND('',#3745,.T.);
#2576=FACE_OUTER_BOUND('',#3746,.T.);
#2577=FACE_OUTER_BOUND('',#3747,.T.);
#2578=FACE_OUTER_BOUND('',#3748,.T.);
#2579=FACE_OUTER_BOUND('',#3749,.T.);
#2580=FACE_OUTER_BOUND('',#3750,.T.);
#2581=FACE_OUTER_BOUND('',#3751,.T.);
#2582=FACE_OUTER_BOUND('',#3752,.T.);
#2583=FACE_OUTER_BOUND('',#3753,.T.);
#2584=FACE_OUTER_BOUND('',#3754,.T.);
#2585=FACE_OUTER_BOUND('',#3755,.T.);
#2586=FACE_OUTER_BOUND('',#3756,.T.);
#2587=FACE_OUTER_BOUND('',#3757,.T.);
#2588=FACE_OUTER_BOUND('',#3758,.T.);
#2589=FACE_OUTER_BOUND('',#3759,.T.);
#2590=FACE_OUTER_BOUND('',#3760,.T.);
#2591=FACE_OUTER_BOUND('',#3761,.T.);
#2592=FACE_OUTER_BOUND('',#3762,.T.);
#2593=FACE_OUTER_BOUND('',#3763,.T.);
#2594=FACE_OUTER_BOUND('',#3764,.T.);
#2595=FACE_OUTER_BOUND('',#3765,.T.);
#2596=FACE_OUTER_BOUND('',#3766,.T.);
#2597=FACE_OUTER_BOUND('',#3767,.T.);
#2598=FACE_OUTER_BOUND('',#3768,.T.);
#2599=FACE_OUTER_BOUND('',#3769,.T.);
#2600=FACE_OUTER_BOUND('',#3770,.T.);
#2601=FACE_OUTER_BOUND('',#3771,.T.);
#2602=FACE_OUTER_BOUND('',#3772,.T.);
#2603=FACE_OUTER_BOUND('',#3773,.T.);
#2604=FACE_OUTER_BOUND('',#3774,.T.);
#2605=FACE_OUTER_BOUND('',#3775,.T.);
#2606=FACE_OUTER_BOUND('',#3776,.T.);
#2607=FACE_OUTER_BOUND('',#3777,.T.);
#2608=FACE_OUTER_BOUND('',#3778,.T.);
#2609=FACE_OUTER_BOUND('',#3779,.T.);
#2610=FACE_OUTER_BOUND('',#3780,.T.);
#2611=FACE_OUTER_BOUND('',#3781,.T.);
#2612=FACE_OUTER_BOUND('',#3782,.T.);
#2613=FACE_OUTER_BOUND('',#3783,.T.);
#2614=FACE_OUTER_BOUND('',#3784,.T.);
#2615=FACE_OUTER_BOUND('',#3785,.T.);
#2616=FACE_OUTER_BOUND('',#3786,.T.);
#2617=FACE_OUTER_BOUND('',#3787,.T.);
#2618=FACE_OUTER_BOUND('',#3788,.T.);
#2619=FACE_OUTER_BOUND('',#3789,.T.);
#2620=FACE_OUTER_BOUND('',#3790,.T.);
#2621=FACE_OUTER_BOUND('',#3791,.T.);
#2622=FACE_OUTER_BOUND('',#3792,.T.);
#2623=FACE_OUTER_BOUND('',#3793,.T.);
#2624=FACE_OUTER_BOUND('',#3794,.T.);
#2625=FACE_OUTER_BOUND('',#3795,.T.);
#2626=FACE_OUTER_BOUND('',#3796,.T.);
#2627=FACE_OUTER_BOUND('',#3797,.T.);
#2628=FACE_OUTER_BOUND('',#3798,.T.);
#2629=FACE_OUTER_BOUND('',#3799,.T.);
#2630=FACE_OUTER_BOUND('',#3800,.T.);
#2631=FACE_OUTER_BOUND('',#3805,.T.);
#2632=FACE_OUTER_BOUND('',#3806,.T.);
#2633=FACE_OUTER_BOUND('',#3807,.T.);
#2634=FACE_OUTER_BOUND('',#3808,.T.);
#2635=FACE_OUTER_BOUND('',#3809,.T.);
#2636=FACE_OUTER_BOUND('',#3810,.T.);
#2637=FACE_OUTER_BOUND('',#3811,.T.);
#2638=FACE_OUTER_BOUND('',#3812,.T.);
#2639=FACE_OUTER_BOUND('',#3813,.T.);
#2640=FACE_OUTER_BOUND('',#3814,.T.);
#2641=FACE_OUTER_BOUND('',#3815,.T.);
#2642=FACE_OUTER_BOUND('',#3816,.T.);
#2643=FACE_OUTER_BOUND('',#3817,.T.);
#2644=FACE_OUTER_BOUND('',#3818,.T.);
#2645=FACE_OUTER_BOUND('',#3819,.T.);
#2646=FACE_OUTER_BOUND('',#3820,.T.);
#2647=FACE_OUTER_BOUND('',#3821,.T.);
#2648=FACE_OUTER_BOUND('',#3822,.T.);
#3733=EDGE_LOOP('',(#13244,#13245,#13246,#13247));
#3734=EDGE_LOOP('',(#13248,#13249,#13250,#13251));
#3735=EDGE_LOOP('',(#13252,#13253,#13254,#13255));
#3736=EDGE_LOOP('',(#13256,#13257,#13258,#13259));
#3737=EDGE_LOOP('',(#13260,#13261,#13262,#13263));
#3738=EDGE_LOOP('',(#13264,#13265,#13266,#13267));
#3739=EDGE_LOOP('',(#13268,#13269,#13270,#13271));
#3740=EDGE_LOOP('',(#13272,#13273,#13274,#13275));
#3741=EDGE_LOOP('',(#13276,#13277,#13278,#13279));
#3742=EDGE_LOOP('',(#13280,#13281,#13282,#13283));
#3743=EDGE_LOOP('',(#13284,#13285,#13286,#13287));
#3744=EDGE_LOOP('',(#13288,#13289,#13290,#13291));
#3745=EDGE_LOOP('',(#13292,#13293,#13294,#13295));
#3746=EDGE_LOOP('',(#13296,#13297,#13298,#13299));
#3747=EDGE_LOOP('',(#13300,#13301,#13302,#13303));
#3748=EDGE_LOOP('',(#13304,#13305,#13306,#13307));
#3749=EDGE_LOOP('',(#13308,#13309,#13310,#13311));
#3750=EDGE_LOOP('',(#13312,#13313,#13314,#13315));
#3751=EDGE_LOOP('',(#13316,#13317,#13318,#13319));
#3752=EDGE_LOOP('',(#13320,#13321,#13322,#13323));
#3753=EDGE_LOOP('',(#13324,#13325,#13326,#13327));
#3754=EDGE_LOOP('',(#13328,#13329,#13330,#13331));
#3755=EDGE_LOOP('',(#13332,#13333,#13334,#13335));
#3756=EDGE_LOOP('',(#13336,#13337,#13338,#13339));
#3757=EDGE_LOOP('',(#13340,#13341,#13342,#13343));
#3758=EDGE_LOOP('',(#13344,#13345,#13346,#13347));
#3759=EDGE_LOOP('',(#13348,#13349,#13350,#13351));
#3760=EDGE_LOOP('',(#13352,#13353,#13354,#13355));
#3761=EDGE_LOOP('',(#13356,#13357,#13358,#13359));
#3762=EDGE_LOOP('',(#13360,#13361,#13362,#13363));
#3763=EDGE_LOOP('',(#13364,#13365,#13366,#13367));
#3764=EDGE_LOOP('',(#13368,#13369,#13370,#13371));
#3765=EDGE_LOOP('',(#13372,#13373,#13374,#13375));
#3766=EDGE_LOOP('',(#13376,#13377,#13378,#13379));
#3767=EDGE_LOOP('',(#13380,#13381,#13382,#13383));
#3768=EDGE_LOOP('',(#13384,#13385,#13386,#13387));
#3769=EDGE_LOOP('',(#13388,#13389,#13390,#13391));
#3770=EDGE_LOOP('',(#13392,#13393,#13394,#13395));
#3771=EDGE_LOOP('',(#13396,#13397,#13398,#13399));
#3772=EDGE_LOOP('',(#13400,#13401,#13402,#13403));
#3773=EDGE_LOOP('',(#13404,#13405,#13406,#13407));
#3774=EDGE_LOOP('',(#13408,#13409,#13410,#13411));
#3775=EDGE_LOOP('',(#13412,#13413,#13414,#13415));
#3776=EDGE_LOOP('',(#13416,#13417,#13418,#13419));
#3777=EDGE_LOOP('',(#13420,#13421,#13422,#13423));
#3778=EDGE_LOOP('',(#13424,#13425,#13426,#13427));
#3779=EDGE_LOOP('',(#13428,#13429,#13430,#13431));
#3780=EDGE_LOOP('',(#13432,#13433,#13434,#13435));
#3781=EDGE_LOOP('',(#13436,#13437,#13438,#13439));
#3782=EDGE_LOOP('',(#13440,#13441,#13442,#13443));
#3783=EDGE_LOOP('',(#13444,#13445,#13446,#13447));
#3784=EDGE_LOOP('',(#13448,#13449,#13450,#13451));
#3785=EDGE_LOOP('',(#13452,#13453,#13454,#13455));
#3786=EDGE_LOOP('',(#13456,#13457,#13458,#13459));
#3787=EDGE_LOOP('',(#13460,#13461,#13462,#13463));
#3788=EDGE_LOOP('',(#13464,#13465,#13466,#13467));
#3789=EDGE_LOOP('',(#13468,#13469,#13470,#13471));
#3790=EDGE_LOOP('',(#13472,#13473,#13474,#13475));
#3791=EDGE_LOOP('',(#13476,#13477,#13478,#13479));
#3792=EDGE_LOOP('',(#13480,#13481,#13482,#13483));
#3793=EDGE_LOOP('',(#13484,#13485,#13486,#13487));
#3794=EDGE_LOOP('',(#13488,#13489,#13490,#13491));
#3795=EDGE_LOOP('',(#13492,#13493,#13494,#13495));
#3796=EDGE_LOOP('',(#13496,#13497,#13498,#13499));
#3797=EDGE_LOOP('',(#13500,#13501,#13502,#13503));
#3798=EDGE_LOOP('',(#13504,#13505,#13506,#13507,#13508,#13509,#13510,#13511,
#13512,#13513,#13514,#13515,#13516,#13517,#13518,#13519,#13520,#13521,#13522,
#13523));
#3799=EDGE_LOOP('',(#13524,#13525,#13526,#13527,#13528,#13529,#13530,#13531,
#13532,#13533,#13534,#13535,#13536,#13537,#13538,#13539,#13540,#13541,#13542,
#13543));
#3800=EDGE_LOOP('',(#13544,#13545,#13546,#13547));
#3801=EDGE_LOOP('',(#13548,#13549,#13550,#13551));
#3802=EDGE_LOOP('',(#13552,#13553,#13554,#13555));
#3803=EDGE_LOOP('',(#13556,#13557,#13558,#13559));
#3804=EDGE_LOOP('',(#13560,#13561,#13562,#13563));
#3805=EDGE_LOOP('',(#13564,#13565,#13566,#13567));
#3806=EDGE_LOOP('',(#13568,#13569,#13570,#13571,#13572,#13573,#13574,#13575,
#13576,#13577,#13578,#13579,#13580,#13581,#13582,#13583,#13584,#13585,#13586,
#13587));
#3807=EDGE_LOOP('',(#13588,#13589,#13590,#13591,#13592,#13593,#13594,#13595,
#13596,#13597,#13598,#13599,#13600,#13601,#13602,#13603,#13604,#13605,#13606,
#13607));
#3808=EDGE_LOOP('',(#13608,#13609,#13610,#13611));
#3809=EDGE_LOOP('',(#13612,#13613,#13614,#13615,#13616,#13617,#13618,#13619,
#13620,#13621,#13622,#13623,#13624,#13625,#13626,#13627,#13628,#13629,#13630,
#13631));
#3810=EDGE_LOOP('',(#13632,#13633,#13634,#13635,#13636,#13637,#13638,#13639,
#13640,#13641,#13642,#13643,#13644,#13645,#13646,#13647,#13648,#13649,#13650,
#13651));
#3811=EDGE_LOOP('',(#13652,#13653,#13654,#13655));
#3812=EDGE_LOOP('',(#13656,#13657,#13658,#13659,#13660,#13661,#13662,#13663,
#13664,#13665,#13666,#13667,#13668,#13669,#13670,#13671,#13672,#13673,#13674,
#13675));
#3813=EDGE_LOOP('',(#13676,#13677,#13678,#13679,#13680,#13681,#13682,#13683,
#13684,#13685,#13686,#13687,#13688,#13689,#13690,#13691,#13692,#13693,#13694,
#13695));
#3814=EDGE_LOOP('',(#13696,#13697,#13698,#13699));
#3815=EDGE_LOOP('',(#13700,#13701,#13702,#13703));
#3816=EDGE_LOOP('',(#13704,#13705,#13706,#13707));
#3817=EDGE_LOOP('',(#13708,#13709,#13710,#13711));
#3818=EDGE_LOOP('',(#13712,#13713,#13714,#13715));
#3819=EDGE_LOOP('',(#13716,#13717,#13718,#13719));
#3820=EDGE_LOOP('',(#13720,#13721,#13722,#13723));
#3821=EDGE_LOOP('',(#13724,#13725,#13726,#13727));
#3822=EDGE_LOOP('',(#13728,#13729,#13730,#13731));
#3823=EDGE_LOOP('',(#13732,#13733,#13734,#13735));
#3824=EDGE_LOOP('',(#13736,#13737,#13738,#13739));
#3825=EDGE_LOOP('',(#13740,#13741,#13742,#13743));
#3826=EDGE_LOOP('',(#13744,#13745,#13746,#13747));
#4990=LINE('',#27784,#6204);
#4991=LINE('',#27805,#6205);
#4992=LINE('',#27856,#6206);
#4993=LINE('',#27907,#6207);
#4994=LINE('',#27955,#6208);
#4995=LINE('',#28006,#6209);
#4996=LINE('',#28057,#6210);
#4997=LINE('',#28105,#6211);
#4998=LINE('',#28144,#6212);
#4999=LINE('',#28165,#6213);
#5000=LINE('',#28216,#6214);
#5001=LINE('',#28267,#6215);
#5002=LINE('',#28315,#6216);
#5003=LINE('',#28366,#6217);
#5004=LINE('',#28417,#6218);
#5005=LINE('',#28465,#6219);
#5006=LINE('',#28504,#6220);
#5007=LINE('',#28525,#6221);
#5008=LINE('',#28576,#6222);
#5009=LINE('',#28627,#6223);
#5010=LINE('',#28675,#6224);
#5011=LINE('',#28726,#6225);
#5012=LINE('',#28777,#6226);
#5013=LINE('',#28825,#6227);
#5014=LINE('',#28864,#6228);
#5015=LINE('',#28885,#6229);
#5016=LINE('',#28936,#6230);
#5017=LINE('',#28987,#6231);
#5018=LINE('',#29035,#6232);
#5019=LINE('',#29086,#6233);
#5020=LINE('',#29137,#6234);
#5021=LINE('',#29185,#6235);
#5022=LINE('',#29224,#6236);
#5023=LINE('',#29248,#6237);
#5024=LINE('',#29272,#6238);
#5025=LINE('',#29297,#6239);
#5026=LINE('',#29322,#6240);
#5027=LINE('',#29346,#6241);
#5028=LINE('',#29371,#6242);
#5029=LINE('',#29396,#6243);
#5030=LINE('',#29413,#6244);
#5031=LINE('',#29437,#6245);
#5032=LINE('',#29461,#6246);
#5033=LINE('',#29486,#6247);
#5034=LINE('',#29511,#6248);
#5035=LINE('',#29535,#6249);
#5036=LINE('',#29560,#6250);
#5037=LINE('',#29585,#6251);
#5038=LINE('',#29602,#6252);
#5039=LINE('',#29626,#6253);
#5040=LINE('',#29650,#6254);
#5041=LINE('',#29675,#6255);
#5042=LINE('',#29700,#6256);
#5043=LINE('',#29724,#6257);
#5044=LINE('',#29749,#6258);
#5045=LINE('',#29774,#6259);
#5046=LINE('',#29791,#6260);
#5047=LINE('',#29815,#6261);
#5048=LINE('',#29839,#6262);
#5049=LINE('',#29864,#6263);
#5050=LINE('',#29889,#6264);
#5051=LINE('',#29913,#6265);
#5052=LINE('',#29938,#6266);
#5053=LINE('',#29963,#6267);
#5054=LINE('',#30882,#6268);
#5055=LINE('',#30884,#6269);
#5056=LINE('',#30886,#6270);
#5057=LINE('',#30887,#6271);
#5058=LINE('',#33601,#6272);
#5059=LINE('',#33602,#6273);
#5060=LINE('',#33603,#6274);
#5061=LINE('',#33606,#6275);
#5062=LINE('',#33607,#6276);
#5063=LINE('',#33610,#6277);
#5064=LINE('',#33611,#6278);
#5065=LINE('',#33613,#6279);
#6204=VECTOR('',#23644,4.);
#6205=VECTOR('',#23649,4.);
#6206=VECTOR('',#23652,4.);
#6207=VECTOR('',#23655,4.);
#6208=VECTOR('',#23658,4.);
#6209=VECTOR('',#23661,4.);
#6210=VECTOR('',#23664,4.);
#6211=VECTOR('',#23667,4.);
#6212=VECTOR('',#23672,4.);
#6213=VECTOR('',#23677,4.);
#6214=VECTOR('',#23680,4.);
#6215=VECTOR('',#23683,4.);
#6216=VECTOR('',#23686,4.);
#6217=VECTOR('',#23689,4.);
#6218=VECTOR('',#23692,4.);
#6219=VECTOR('',#23695,4.);
#6220=VECTOR('',#23700,4.);
#6221=VECTOR('',#23705,4.);
#6222=VECTOR('',#23708,4.);
#6223=VECTOR('',#23711,4.);
#6224=VECTOR('',#23714,4.);
#6225=VECTOR('',#23717,4.);
#6226=VECTOR('',#23720,4.);
#6227=VECTOR('',#23723,4.);
#6228=VECTOR('',#23728,4.);
#6229=VECTOR('',#23733,4.);
#6230=VECTOR('',#23736,4.);
#6231=VECTOR('',#23739,4.);
#6232=VECTOR('',#23742,4.);
#6233=VECTOR('',#23745,4.);
#6234=VECTOR('',#23748,4.);
#6235=VECTOR('',#23751,4.);
#6236=VECTOR('',#23756,4.07350000000001);
#6237=VECTOR('',#23761,4.07350000000001);
#6238=VECTOR('',#23764,4.07350000000001);
#6239=VECTOR('',#23767,4.07350000000001);
#6240=VECTOR('',#23770,4.07350000000001);
#6241=VECTOR('',#23773,4.07350000000001);
#6242=VECTOR('',#23776,4.07350000000001);
#6243=VECTOR('',#23779,4.07350000000001);
#6244=VECTOR('',#23784,4.0735);
#6245=VECTOR('',#23789,4.0735);
#6246=VECTOR('',#23792,4.0735);
#6247=VECTOR('',#23795,4.0735);
#6248=VECTOR('',#23798,4.0735);
#6249=VECTOR('',#23801,4.0735);
#6250=VECTOR('',#23804,4.0735);
#6251=VECTOR('',#23807,4.0735);
#6252=VECTOR('',#23812,4.0735);
#6253=VECTOR('',#23817,4.0735);
#6254=VECTOR('',#23820,4.0735);
#6255=VECTOR('',#23823,4.0735);
#6256=VECTOR('',#23826,4.0735);
#6257=VECTOR('',#23829,4.0735);
#6258=VECTOR('',#23832,4.0735);
#6259=VECTOR('',#23835,4.0735);
#6260=VECTOR('',#23840,4.07350000000001);
#6261=VECTOR('',#23845,4.07350000000001);
#6262=VECTOR('',#23848,4.07350000000001);
#6263=VECTOR('',#23851,4.07350000000001);
#6264=VECTOR('',#23854,4.07350000000001);
#6265=VECTOR('',#23857,4.07350000000001);
#6266=VECTOR('',#23860,4.07350000000001);
#6267=VECTOR('',#23863,4.07350000000001);
#6268=VECTOR('',#23870,10.);
#6269=VECTOR('',#23871,10.);
#6270=VECTOR('',#23872,10.);
#6271=VECTOR('',#23873,10.);
#6272=VECTOR('',#23890,10.);
#6273=VECTOR('',#23891,10.);
#6274=VECTOR('',#23892,10.);
#6275=VECTOR('',#23895,10.);
#6276=VECTOR('',#23896,10.);
#6277=VECTOR('',#23899,10.);
#6278=VECTOR('',#23900,10.);
#6279=VECTOR('',#23903,10.);
#7376=CIRCLE('',#22084,3.5175);
#7377=CIRCLE('',#22092,3.5175);
#7378=CIRCLE('',#22094,3.5175);
#7379=CIRCLE('',#22102,3.5175);
#7380=CIRCLE('',#22104,3.5175);
#7381=CIRCLE('',#22112,3.5175);
#7382=CIRCLE('',#22114,3.5175);
#7383=CIRCLE('',#22122,3.5175);
#7384=CIRCLE('',#22124,4.0735);
#7385=CIRCLE('',#22132,4.07350000000001);
#7386=CIRCLE('',#22134,4.0735);
#7387=CIRCLE('',#22142,4.0735);
#7388=CIRCLE('',#22144,4.0735);
#7389=CIRCLE('',#22152,4.0735);
#7390=CIRCLE('',#22154,4.0735);
#7391=CIRCLE('',#22162,4.07350000000001);
#7657=VERTEX_POINT('',#27782);
#7658=VERTEX_POINT('',#27783);
#7659=VERTEX_POINT('',#27785);
#7660=VERTEX_POINT('',#27790);
#7661=VERTEX_POINT('',#27803);
#7662=VERTEX_POINT('',#27804);
#7663=VERTEX_POINT('',#27854);
#7664=VERTEX_POINT('',#27855);
#7665=VERTEX_POINT('',#27905);
#7666=VERTEX_POINT('',#27906);
#7667=VERTEX_POINT('',#27953);
#7668=VERTEX_POINT('',#27954);
#7669=VERTEX_POINT('',#28004);
#7670=VERTEX_POINT('',#28005);
#7671=VERTEX_POINT('',#28055);
#7672=VERTEX_POINT('',#28056);
#7673=VERTEX_POINT('',#28103);
#7674=VERTEX_POINT('',#28104);
#7675=VERTEX_POINT('',#28106);
#7676=VERTEX_POINT('',#28120);
#7677=VERTEX_POINT('',#28142);
#7678=VERTEX_POINT('',#28143);
#7679=VERTEX_POINT('',#28145);
#7680=VERTEX_POINT('',#28150);
#7681=VERTEX_POINT('',#28163);
#7682=VERTEX_POINT('',#28164);
#7683=VERTEX_POINT('',#28214);
#7684=VERTEX_POINT('',#28215);
#7685=VERTEX_POINT('',#28265);
#7686=VERTEX_POINT('',#28266);
#7687=VERTEX_POINT('',#28313);
#7688=VERTEX_POINT('',#28314);
#7689=VERTEX_POINT('',#28364);
#7690=VERTEX_POINT('',#28365);
#7691=VERTEX_POINT('',#28415);
#7692=VERTEX_POINT('',#28416);
#7693=VERTEX_POINT('',#28463);
#7694=VERTEX_POINT('',#28464);
#7695=VERTEX_POINT('',#28466);
#7696=VERTEX_POINT('',#28480);
#7697=VERTEX_POINT('',#28502);
#7698=VERTEX_POINT('',#28503);
#7699=VERTEX_POINT('',#28505);
#7700=VERTEX_POINT('',#28510);
#7701=VERTEX_POINT('',#28523);
#7702=VERTEX_POINT('',#28524);
#7703=VERTEX_POINT('',#28574);
#7704=VERTEX_POINT('',#28575);
#7705=VERTEX_POINT('',#28625);
#7706=VERTEX_POINT('',#28626);
#7707=VERTEX_POINT('',#28673);
#7708=VERTEX_POINT('',#28674);
#7709=VERTEX_POINT('',#28724);
#7710=VERTEX_POINT('',#28725);
#7711=VERTEX_POINT('',#28775);
#7712=VERTEX_POINT('',#28776);
#7713=VERTEX_POINT('',#28823);
#7714=VERTEX_POINT('',#28824);
#7715=VERTEX_POINT('',#28826);
#7716=VERTEX_POINT('',#28840);
#7717=VERTEX_POINT('',#28862);
#7718=VERTEX_POINT('',#28863);
#7719=VERTEX_POINT('',#28865);
#7720=VERTEX_POINT('',#28870);
#7721=VERTEX_POINT('',#28883);
#7722=VERTEX_POINT('',#28884);
#7723=VERTEX_POINT('',#28934);
#7724=VERTEX_POINT('',#28935);
#7725=VERTEX_POINT('',#28985);
#7726=VERTEX_POINT('',#28986);
#7727=VERTEX_POINT('',#29033);
#7728=VERTEX_POINT('',#29034);
#7729=VERTEX_POINT('',#29084);
#7730=VERTEX_POINT('',#29085);
#7731=VERTEX_POINT('',#29135);
#7732=VERTEX_POINT('',#29136);
#7733=VERTEX_POINT('',#29183);
#7734=VERTEX_POINT('',#29184);
#7735=VERTEX_POINT('',#29186);
#7736=VERTEX_POINT('',#29200);
#7737=VERTEX_POINT('',#29222);
#7738=VERTEX_POINT('',#29223);
#7739=VERTEX_POINT('',#29225);
#7740=VERTEX_POINT('',#29234);
#7741=VERTEX_POINT('',#29246);
#7742=VERTEX_POINT('',#29247);
#7743=VERTEX_POINT('',#29270);
#7744=VERTEX_POINT('',#29271);
#7745=VERTEX_POINT('',#29295);
#7746=VERTEX_POINT('',#29296);
#7747=VERTEX_POINT('',#29320);
#7748=VERTEX_POINT('',#29321);
#7749=VERTEX_POINT('',#29344);
#7750=VERTEX_POINT('',#29345);
#7751=VERTEX_POINT('',#29369);
#7752=VERTEX_POINT('',#29370);
#7753=VERTEX_POINT('',#29394);
#7754=VERTEX_POINT('',#29395);
#7755=VERTEX_POINT('',#29397);
#7756=VERTEX_POINT('',#29403);
#7757=VERTEX_POINT('',#29411);
#7758=VERTEX_POINT('',#29412);
#7759=VERTEX_POINT('',#29414);
#7760=VERTEX_POINT('',#29423);
#7761=VERTEX_POINT('',#29435);
#7762=VERTEX_POINT('',#29436);
#7763=VERTEX_POINT('',#29459);
#7764=VERTEX_POINT('',#29460);
#7765=VERTEX_POINT('',#29484);
#7766=VERTEX_POINT('',#29485);
#7767=VERTEX_POINT('',#29509);
#7768=VERTEX_POINT('',#29510);
#7769=VERTEX_POINT('',#29533);
#7770=VERTEX_POINT('',#29534);
#7771=VERTEX_POINT('',#29558);
#7772=VERTEX_POINT('',#29559);
#7773=VERTEX_POINT('',#29583);
#7774=VERTEX_POINT('',#29584);
#7775=VERTEX_POINT('',#29586);
#7776=VERTEX_POINT('',#29592);
#7777=VERTEX_POINT('',#29600);
#7778=VERTEX_POINT('',#29601);
#7779=VERTEX_POINT('',#29603);
#7780=VERTEX_POINT('',#29612);
#7781=VERTEX_POINT('',#29624);
#7782=VERTEX_POINT('',#29625);
#7783=VERTEX_POINT('',#29648);
#7784=VERTEX_POINT('',#29649);
#7785=VERTEX_POINT('',#29673);
#7786=VERTEX_POINT('',#29674);
#7787=VERTEX_POINT('',#29698);
#7788=VERTEX_POINT('',#29699);
#7789=VERTEX_POINT('',#29722);
#7790=VERTEX_POINT('',#29723);
#7791=VERTEX_POINT('',#29747);
#7792=VERTEX_POINT('',#29748);
#7793=VERTEX_POINT('',#29772);
#7794=VERTEX_POINT('',#29773);
#7795=VERTEX_POINT('',#29775);
#7796=VERTEX_POINT('',#29781);
#7797=VERTEX_POINT('',#29789);
#7798=VERTEX_POINT('',#29790);
#7799=VERTEX_POINT('',#29792);
#7800=VERTEX_POINT('',#29801);
#7801=VERTEX_POINT('',#29813);
#7802=VERTEX_POINT('',#29814);
#7803=VERTEX_POINT('',#29837);
#7804=VERTEX_POINT('',#29838);
#7805=VERTEX_POINT('',#29862);
#7806=VERTEX_POINT('',#29863);
#7807=VERTEX_POINT('',#29887);
#7808=VERTEX_POINT('',#29888);
#7809=VERTEX_POINT('',#29911);
#7810=VERTEX_POINT('',#29912);
#7811=VERTEX_POINT('',#29936);
#7812=VERTEX_POINT('',#29937);
#7813=VERTEX_POINT('',#29961);
#7814=VERTEX_POINT('',#29962);
#7815=VERTEX_POINT('',#29964);
#7816=VERTEX_POINT('',#29970);
#7817=VERTEX_POINT('',#30880);
#7818=VERTEX_POINT('',#30881);
#7819=VERTEX_POINT('',#30883);
#7820=VERTEX_POINT('',#30885);
#7821=VERTEX_POINT('',#33599);
#7822=VERTEX_POINT('',#33600);
#7823=VERTEX_POINT('',#33605);
#7824=VERTEX_POINT('',#33609);
#9879=EDGE_CURVE('',#7657,#7658,#4990,.T.);
#9880=EDGE_CURVE('',#7658,#7659,#376,.T.);
#9881=EDGE_CURVE('',#7660,#7659,#7376,.F.);
#9882=EDGE_CURVE('',#7660,#7657,#377,.T.);
#9883=EDGE_CURVE('',#7661,#7662,#4991,.T.);
#9884=EDGE_CURVE('',#7662,#7658,#378,.T.);
#9885=EDGE_CURVE('',#7657,#7661,#379,.T.);
#9886=EDGE_CURVE('',#7663,#7664,#4992,.T.);
#9887=EDGE_CURVE('',#7664,#7662,#380,.T.);
#9888=EDGE_CURVE('',#7661,#7663,#381,.T.);
#9889=EDGE_CURVE('',#7665,#7666,#4993,.T.);
#9890=EDGE_CURVE('',#7666,#7664,#382,.T.);
#9891=EDGE_CURVE('',#7663,#7665,#383,.T.);
#9892=EDGE_CURVE('',#7667,#7668,#4994,.T.);
#9893=EDGE_CURVE('',#7668,#7666,#384,.T.);
#9894=EDGE_CURVE('',#7665,#7667,#385,.T.);
#9895=EDGE_CURVE('',#7669,#7670,#4995,.T.);
#9896=EDGE_CURVE('',#7670,#7668,#386,.T.);
#9897=EDGE_CURVE('',#7667,#7669,#387,.T.);
#9898=EDGE_CURVE('',#7671,#7672,#4996,.T.);
#9899=EDGE_CURVE('',#7672,#7670,#388,.T.);
#9900=EDGE_CURVE('',#7669,#7671,#389,.T.);
#9901=EDGE_CURVE('',#7673,#7674,#4997,.T.);
#9902=EDGE_CURVE('',#7673,#7675,#390,.T.);
#9903=EDGE_CURVE('',#7676,#7675,#7377,.T.);
#9904=EDGE_CURVE('',#7676,#7674,#391,.T.);
#9905=EDGE_CURVE('',#7677,#7678,#4998,.T.);
#9906=EDGE_CURVE('',#7678,#7679,#392,.T.);
#9907=EDGE_CURVE('',#7680,#7679,#7378,.F.);
#9908=EDGE_CURVE('',#7680,#7677,#393,.T.);
#9909=EDGE_CURVE('',#7681,#7682,#4999,.T.);
#9910=EDGE_CURVE('',#7682,#7678,#394,.T.);
#9911=EDGE_CURVE('',#7677,#7681,#395,.T.);
#9912=EDGE_CURVE('',#7683,#7684,#5000,.T.);
#9913=EDGE_CURVE('',#7684,#7682,#396,.T.);
#9914=EDGE_CURVE('',#7681,#7683,#397,.T.);
#9915=EDGE_CURVE('',#7685,#7686,#5001,.T.);
#9916=EDGE_CURVE('',#7686,#7684,#398,.T.);
#9917=EDGE_CURVE('',#7683,#7685,#399,.T.);
#9918=EDGE_CURVE('',#7687,#7688,#5002,.T.);
#9919=EDGE_CURVE('',#7688,#7686,#400,.T.);
#9920=EDGE_CURVE('',#7685,#7687,#401,.T.);
#9921=EDGE_CURVE('',#7689,#7690,#5003,.T.);
#9922=EDGE_CURVE('',#7690,#7688,#402,.T.);
#9923=EDGE_CURVE('',#7687,#7689,#403,.T.);
#9924=EDGE_CURVE('',#7691,#7692,#5004,.T.);
#9925=EDGE_CURVE('',#7692,#7690,#404,.T.);
#9926=EDGE_CURVE('',#7689,#7691,#405,.T.);
#9927=EDGE_CURVE('',#7693,#7694,#5005,.T.);
#9928=EDGE_CURVE('',#7693,#7695,#406,.T.);
#9929=EDGE_CURVE('',#7696,#7695,#7379,.T.);
#9930=EDGE_CURVE('',#7696,#7694,#407,.T.);
#9931=EDGE_CURVE('',#7697,#7698,#5006,.T.);
#9932=EDGE_CURVE('',#7698,#7699,#408,.T.);
#9933=EDGE_CURVE('',#7700,#7699,#7380,.F.);
#9934=EDGE_CURVE('',#7700,#7697,#409,.T.);
#9935=EDGE_CURVE('',#7701,#7702,#5007,.T.);
#9936=EDGE_CURVE('',#7702,#7698,#410,.T.);
#9937=EDGE_CURVE('',#7697,#7701,#411,.T.);
#9938=EDGE_CURVE('',#7703,#7704,#5008,.T.);
#9939=EDGE_CURVE('',#7704,#7702,#412,.T.);
#9940=EDGE_CURVE('',#7701,#7703,#413,.T.);
#9941=EDGE_CURVE('',#7705,#7706,#5009,.T.);
#9942=EDGE_CURVE('',#7706,#7704,#414,.T.);
#9943=EDGE_CURVE('',#7703,#7705,#415,.T.);
#9944=EDGE_CURVE('',#7707,#7708,#5010,.T.);
#9945=EDGE_CURVE('',#7708,#7706,#416,.T.);
#9946=EDGE_CURVE('',#7705,#7707,#417,.T.);
#9947=EDGE_CURVE('',#7709,#7710,#5011,.T.);
#9948=EDGE_CURVE('',#7710,#7708,#418,.T.);
#9949=EDGE_CURVE('',#7707,#7709,#419,.T.);
#9950=EDGE_CURVE('',#7711,#7712,#5012,.T.);
#9951=EDGE_CURVE('',#7712,#7710,#420,.T.);
#9952=EDGE_CURVE('',#7709,#7711,#421,.T.);
#9953=EDGE_CURVE('',#7713,#7714,#5013,.T.);
#9954=EDGE_CURVE('',#7713,#7715,#422,.T.);
#9955=EDGE_CURVE('',#7716,#7715,#7381,.T.);
#9956=EDGE_CURVE('',#7716,#7714,#423,.T.);
#9957=EDGE_CURVE('',#7717,#7718,#5014,.T.);
#9958=EDGE_CURVE('',#7718,#7719,#424,.T.);
#9959=EDGE_CURVE('',#7720,#7719,#7382,.F.);
#9960=EDGE_CURVE('',#7720,#7717,#425,.T.);
#9961=EDGE_CURVE('',#7721,#7722,#5015,.T.);
#9962=EDGE_CURVE('',#7722,#7718,#426,.T.);
#9963=EDGE_CURVE('',#7717,#7721,#427,.T.);
#9964=EDGE_CURVE('',#7723,#7724,#5016,.T.);
#9965=EDGE_CURVE('',#7724,#7722,#428,.T.);
#9966=EDGE_CURVE('',#7721,#7723,#429,.T.);
#9967=EDGE_CURVE('',#7725,#7726,#5017,.T.);
#9968=EDGE_CURVE('',#7726,#7724,#430,.T.);
#9969=EDGE_CURVE('',#7723,#7725,#431,.T.);
#9970=EDGE_CURVE('',#7727,#7728,#5018,.T.);
#9971=EDGE_CURVE('',#7728,#7726,#432,.T.);
#9972=EDGE_CURVE('',#7725,#7727,#433,.T.);
#9973=EDGE_CURVE('',#7729,#7730,#5019,.T.);
#9974=EDGE_CURVE('',#7730,#7728,#434,.T.);
#9975=EDGE_CURVE('',#7727,#7729,#435,.T.);
#9976=EDGE_CURVE('',#7731,#7732,#5020,.T.);
#9977=EDGE_CURVE('',#7732,#7730,#436,.T.);
#9978=EDGE_CURVE('',#7729,#7731,#437,.T.);
#9979=EDGE_CURVE('',#7733,#7734,#5021,.T.);
#9980=EDGE_CURVE('',#7733,#7735,#438,.T.);
#9981=EDGE_CURVE('',#7736,#7735,#7383,.T.);
#9982=EDGE_CURVE('',#7736,#7734,#439,.T.);
#9983=EDGE_CURVE('',#7737,#7738,#5022,.T.);
#9984=EDGE_CURVE('',#7738,#7739,#440,.T.);
#9985=EDGE_CURVE('',#7740,#7739,#7384,.T.);
#9986=EDGE_CURVE('',#7737,#7740,#441,.T.);
#9987=EDGE_CURVE('',#7741,#7742,#5023,.T.);
#9988=EDGE_CURVE('',#7742,#7738,#442,.T.);
#9989=EDGE_CURVE('',#7741,#7737,#443,.T.);
#9990=EDGE_CURVE('',#7743,#7744,#5024,.T.);
#9991=EDGE_CURVE('',#7744,#7742,#444,.T.);
#9992=EDGE_CURVE('',#7743,#7741,#445,.T.);
#9993=EDGE_CURVE('',#7745,#7746,#5025,.T.);
#9994=EDGE_CURVE('',#7746,#7744,#446,.T.);
#9995=EDGE_CURVE('',#7745,#7743,#447,.T.);
#9996=EDGE_CURVE('',#7747,#7748,#5026,.T.);
#9997=EDGE_CURVE('',#7748,#7746,#448,.T.);
#9998=EDGE_CURVE('',#7747,#7745,#449,.T.);
#9999=EDGE_CURVE('',#7749,#7750,#5027,.T.);
#10000=EDGE_CURVE('',#7750,#7748,#450,.T.);
#10001=EDGE_CURVE('',#7749,#7747,#451,.T.);
#10002=EDGE_CURVE('',#7751,#7752,#5028,.T.);
#10003=EDGE_CURVE('',#7752,#7750,#452,.T.);
#10004=EDGE_CURVE('',#7751,#7749,#453,.T.);
#10005=EDGE_CURVE('',#7753,#7754,#5029,.T.);
#10006=EDGE_CURVE('',#7755,#7753,#454,.T.);
#10007=EDGE_CURVE('',#7756,#7755,#7385,.T.);
#10008=EDGE_CURVE('',#7756,#7754,#455,.T.);
#10009=EDGE_CURVE('',#7757,#7758,#5030,.T.);
#10010=EDGE_CURVE('',#7758,#7759,#456,.T.);
#10011=EDGE_CURVE('',#7760,#7759,#7386,.T.);
#10012=EDGE_CURVE('',#7757,#7760,#457,.T.);
#10013=EDGE_CURVE('',#7761,#7762,#5031,.T.);
#10014=EDGE_CURVE('',#7762,#7758,#458,.T.);
#10015=EDGE_CURVE('',#7761,#7757,#459,.T.);
#10016=EDGE_CURVE('',#7763,#7764,#5032,.T.);
#10017=EDGE_CURVE('',#7764,#7762,#460,.T.);
#10018=EDGE_CURVE('',#7763,#7761,#461,.T.);
#10019=EDGE_CURVE('',#7765,#7766,#5033,.T.);
#10020=EDGE_CURVE('',#7766,#7764,#462,.T.);
#10021=EDGE_CURVE('',#7765,#7763,#463,.T.);
#10022=EDGE_CURVE('',#7767,#7768,#5034,.T.);
#10023=EDGE_CURVE('',#7768,#7766,#464,.T.);
#10024=EDGE_CURVE('',#7767,#7765,#465,.T.);
#10025=EDGE_CURVE('',#7769,#7770,#5035,.T.);
#10026=EDGE_CURVE('',#7770,#7768,#466,.T.);
#10027=EDGE_CURVE('',#7769,#7767,#467,.T.);
#10028=EDGE_CURVE('',#7771,#7772,#5036,.T.);
#10029=EDGE_CURVE('',#7772,#7770,#468,.T.);
#10030=EDGE_CURVE('',#7771,#7769,#469,.T.);
#10031=EDGE_CURVE('',#7773,#7774,#5037,.T.);
#10032=EDGE_CURVE('',#7775,#7773,#470,.T.);
#10033=EDGE_CURVE('',#7776,#7775,#7387,.T.);
#10034=EDGE_CURVE('',#7776,#7774,#471,.T.);
#10035=EDGE_CURVE('',#7777,#7778,#5038,.T.);
#10036=EDGE_CURVE('',#7778,#7779,#472,.T.);
#10037=EDGE_CURVE('',#7780,#7779,#7388,.T.);
#10038=EDGE_CURVE('',#7777,#7780,#473,.T.);
#10039=EDGE_CURVE('',#7781,#7782,#5039,.T.);
#10040=EDGE_CURVE('',#7782,#7778,#474,.T.);
#10041=EDGE_CURVE('',#7781,#7777,#475,.T.);
#10042=EDGE_CURVE('',#7783,#7784,#5040,.T.);
#10043=EDGE_CURVE('',#7784,#7782,#476,.T.);
#10044=EDGE_CURVE('',#7783,#7781,#477,.T.);
#10045=EDGE_CURVE('',#7785,#7786,#5041,.T.);
#10046=EDGE_CURVE('',#7786,#7784,#478,.T.);
#10047=EDGE_CURVE('',#7785,#7783,#479,.T.);
#10048=EDGE_CURVE('',#7787,#7788,#5042,.T.);
#10049=EDGE_CURVE('',#7788,#7786,#480,.T.);
#10050=EDGE_CURVE('',#7787,#7785,#481,.T.);
#10051=EDGE_CURVE('',#7789,#7790,#5043,.T.);
#10052=EDGE_CURVE('',#7790,#7788,#482,.T.);
#10053=EDGE_CURVE('',#7789,#7787,#483,.T.);
#10054=EDGE_CURVE('',#7791,#7792,#5044,.T.);
#10055=EDGE_CURVE('',#7792,#7790,#484,.T.);
#10056=EDGE_CURVE('',#7791,#7789,#485,.T.);
#10057=EDGE_CURVE('',#7793,#7794,#5045,.T.);
#10058=EDGE_CURVE('',#7795,#7793,#486,.T.);
#10059=EDGE_CURVE('',#7796,#7795,#7389,.T.);
#10060=EDGE_CURVE('',#7796,#7794,#487,.T.);
#10061=EDGE_CURVE('',#7797,#7798,#5046,.T.);
#10062=EDGE_CURVE('',#7798,#7799,#488,.T.);
#10063=EDGE_CURVE('',#7800,#7799,#7390,.T.);
#10064=EDGE_CURVE('',#7797,#7800,#489,.T.);
#10065=EDGE_CURVE('',#7801,#7802,#5047,.T.);
#10066=EDGE_CURVE('',#7802,#7798,#490,.T.);
#10067=EDGE_CURVE('',#7801,#7797,#491,.T.);
#10068=EDGE_CURVE('',#7803,#7804,#5048,.T.);
#10069=EDGE_CURVE('',#7804,#7802,#492,.T.);
#10070=EDGE_CURVE('',#7803,#7801,#493,.T.);
#10071=EDGE_CURVE('',#7805,#7806,#5049,.T.);
#10072=EDGE_CURVE('',#7806,#7804,#494,.T.);
#10073=EDGE_CURVE('',#7805,#7803,#495,.T.);
#10074=EDGE_CURVE('',#7807,#7808,#5050,.T.);
#10075=EDGE_CURVE('',#7808,#7806,#496,.T.);
#10076=EDGE_CURVE('',#7807,#7805,#497,.T.);
#10077=EDGE_CURVE('',#7809,#7810,#5051,.T.);
#10078=EDGE_CURVE('',#7810,#7808,#498,.T.);
#10079=EDGE_CURVE('',#7809,#7807,#499,.T.);
#10080=EDGE_CURVE('',#7811,#7812,#5052,.T.);
#10081=EDGE_CURVE('',#7812,#7810,#500,.T.);
#10082=EDGE_CURVE('',#7811,#7809,#501,.T.);
#10083=EDGE_CURVE('',#7813,#7814,#5053,.T.);
#10084=EDGE_CURVE('',#7815,#7813,#502,.T.);
#10085=EDGE_CURVE('',#7816,#7815,#7391,.T.);
#10086=EDGE_CURVE('',#7816,#7814,#503,.T.);
#10087=EDGE_CURVE('',#7814,#7812,#504,.T.);
#10088=EDGE_CURVE('',#7813,#7811,#505,.T.);
#10089=EDGE_CURVE('',#7799,#7660,#506,.T.);
#10090=EDGE_CURVE('',#7675,#7816,#507,.T.);
#10091=EDGE_CURVE('',#7671,#7673,#508,.T.);
#10092=EDGE_CURVE('',#7659,#7800,#509,.T.);
#10093=EDGE_CURVE('',#7674,#7672,#510,.T.);
#10094=EDGE_CURVE('',#7815,#7676,#511,.T.);
#10095=EDGE_CURVE('',#7817,#7818,#5054,.T.);
#10096=EDGE_CURVE('',#7818,#7819,#5055,.T.);
#10097=EDGE_CURVE('',#7819,#7820,#5056,.T.);
#10098=EDGE_CURVE('',#7820,#7817,#5057,.T.);
#10099=EDGE_CURVE('',#7735,#7776,#512,.T.);
#10100=EDGE_CURVE('',#7775,#7736,#513,.T.);
#10101=EDGE_CURVE('',#7715,#7796,#514,.T.);
#10102=EDGE_CURVE('',#7795,#7716,#515,.T.);
#10103=EDGE_CURVE('',#7695,#7756,#516,.T.);
#10104=EDGE_CURVE('',#7755,#7696,#517,.T.);
#10105=EDGE_CURVE('',#7794,#7792,#518,.T.);
#10106=EDGE_CURVE('',#7793,#7791,#519,.T.);
#10107=EDGE_CURVE('',#7779,#7700,#520,.T.);
#10108=EDGE_CURVE('',#7711,#7713,#521,.T.);
#10109=EDGE_CURVE('',#7699,#7780,#522,.T.);
#10110=EDGE_CURVE('',#7714,#7712,#523,.T.);
#10111=EDGE_CURVE('',#7774,#7772,#524,.T.);
#10112=EDGE_CURVE('',#7773,#7771,#525,.T.);
#10113=EDGE_CURVE('',#7759,#7720,#526,.T.);
#10114=EDGE_CURVE('',#7731,#7733,#527,.T.);
#10115=EDGE_CURVE('',#7719,#7760,#528,.T.);
#10116=EDGE_CURVE('',#7734,#7732,#529,.T.);
#10117=EDGE_CURVE('',#7754,#7752,#530,.T.);
#10118=EDGE_CURVE('',#7753,#7751,#531,.T.);
#10119=EDGE_CURVE('',#7739,#7680,#532,.T.);
#10120=EDGE_CURVE('',#7691,#7693,#533,.T.);
#10121=EDGE_CURVE('',#7679,#7740,#534,.T.);
#10122=EDGE_CURVE('',#7694,#7692,#535,.T.);
#10123=EDGE_CURVE('',#7821,#7822,#5058,.T.);
#10124=EDGE_CURVE('',#7822,#7817,#5059,.T.);
#10125=EDGE_CURVE('',#7821,#7820,#5060,.T.);
#10126=EDGE_CURVE('',#7823,#7821,#5061,.T.);
#10127=EDGE_CURVE('',#7823,#7819,#5062,.T.);
#10128=EDGE_CURVE('',#7824,#7823,#5063,.T.);
#10129=EDGE_CURVE('',#7824,#7818,#5064,.T.);
#10130=EDGE_CURVE('',#7822,#7824,#5065,.T.);
#13244=ORIENTED_EDGE('',*,*,#9879,.T.);
#13245=ORIENTED_EDGE('',*,*,#9880,.T.);
#13246=ORIENTED_EDGE('',*,*,#9881,.F.);
#13247=ORIENTED_EDGE('',*,*,#9882,.T.);
#13248=ORIENTED_EDGE('',*,*,#9883,.T.);
#13249=ORIENTED_EDGE('',*,*,#9884,.T.);
#13250=ORIENTED_EDGE('',*,*,#9879,.F.);
#13251=ORIENTED_EDGE('',*,*,#9885,.T.);
#13252=ORIENTED_EDGE('',*,*,#9886,.T.);
#13253=ORIENTED_EDGE('',*,*,#9887,.T.);
#13254=ORIENTED_EDGE('',*,*,#9883,.F.);
#13255=ORIENTED_EDGE('',*,*,#9888,.T.);
#13256=ORIENTED_EDGE('',*,*,#9889,.T.);
#13257=ORIENTED_EDGE('',*,*,#9890,.T.);
#13258=ORIENTED_EDGE('',*,*,#9886,.F.);
#13259=ORIENTED_EDGE('',*,*,#9891,.T.);
#13260=ORIENTED_EDGE('',*,*,#9892,.T.);
#13261=ORIENTED_EDGE('',*,*,#9893,.T.);
#13262=ORIENTED_EDGE('',*,*,#9889,.F.);
#13263=ORIENTED_EDGE('',*,*,#9894,.T.);
#13264=ORIENTED_EDGE('',*,*,#9895,.T.);
#13265=ORIENTED_EDGE('',*,*,#9896,.T.);
#13266=ORIENTED_EDGE('',*,*,#9892,.F.);
#13267=ORIENTED_EDGE('',*,*,#9897,.T.);
#13268=ORIENTED_EDGE('',*,*,#9898,.T.);
#13269=ORIENTED_EDGE('',*,*,#9899,.T.);
#13270=ORIENTED_EDGE('',*,*,#9895,.F.);
#13271=ORIENTED_EDGE('',*,*,#9900,.T.);
#13272=ORIENTED_EDGE('',*,*,#9901,.F.);
#13273=ORIENTED_EDGE('',*,*,#9902,.T.);
#13274=ORIENTED_EDGE('',*,*,#9903,.F.);
#13275=ORIENTED_EDGE('',*,*,#9904,.T.);
#13276=ORIENTED_EDGE('',*,*,#9905,.T.);
#13277=ORIENTED_EDGE('',*,*,#9906,.T.);
#13278=ORIENTED_EDGE('',*,*,#9907,.F.);
#13279=ORIENTED_EDGE('',*,*,#9908,.T.);
#13280=ORIENTED_EDGE('',*,*,#9909,.T.);
#13281=ORIENTED_EDGE('',*,*,#9910,.T.);
#13282=ORIENTED_EDGE('',*,*,#9905,.F.);
#13283=ORIENTED_EDGE('',*,*,#9911,.T.);
#13284=ORIENTED_EDGE('',*,*,#9912,.T.);
#13285=ORIENTED_EDGE('',*,*,#9913,.T.);
#13286=ORIENTED_EDGE('',*,*,#9909,.F.);
#13287=ORIENTED_EDGE('',*,*,#9914,.T.);
#13288=ORIENTED_EDGE('',*,*,#9915,.T.);
#13289=ORIENTED_EDGE('',*,*,#9916,.T.);
#13290=ORIENTED_EDGE('',*,*,#9912,.F.);
#13291=ORIENTED_EDGE('',*,*,#9917,.T.);
#13292=ORIENTED_EDGE('',*,*,#9918,.T.);
#13293=ORIENTED_EDGE('',*,*,#9919,.T.);
#13294=ORIENTED_EDGE('',*,*,#9915,.F.);
#13295=ORIENTED_EDGE('',*,*,#9920,.T.);
#13296=ORIENTED_EDGE('',*,*,#9921,.T.);
#13297=ORIENTED_EDGE('',*,*,#9922,.T.);
#13298=ORIENTED_EDGE('',*,*,#9918,.F.);
#13299=ORIENTED_EDGE('',*,*,#9923,.T.);
#13300=ORIENTED_EDGE('',*,*,#9924,.T.);
#13301=ORIENTED_EDGE('',*,*,#9925,.T.);
#13302=ORIENTED_EDGE('',*,*,#9921,.F.);
#13303=ORIENTED_EDGE('',*,*,#9926,.T.);
#13304=ORIENTED_EDGE('',*,*,#9927,.F.);
#13305=ORIENTED_EDGE('',*,*,#9928,.T.);
#13306=ORIENTED_EDGE('',*,*,#9929,.F.);
#13307=ORIENTED_EDGE('',*,*,#9930,.T.);
#13308=ORIENTED_EDGE('',*,*,#9931,.T.);
#13309=ORIENTED_EDGE('',*,*,#9932,.T.);
#13310=ORIENTED_EDGE('',*,*,#9933,.F.);
#13311=ORIENTED_EDGE('',*,*,#9934,.T.);
#13312=ORIENTED_EDGE('',*,*,#9935,.T.);
#13313=ORIENTED_EDGE('',*,*,#9936,.T.);
#13314=ORIENTED_EDGE('',*,*,#9931,.F.);
#13315=ORIENTED_EDGE('',*,*,#9937,.T.);
#13316=ORIENTED_EDGE('',*,*,#9938,.T.);
#13317=ORIENTED_EDGE('',*,*,#9939,.T.);
#13318=ORIENTED_EDGE('',*,*,#9935,.F.);
#13319=ORIENTED_EDGE('',*,*,#9940,.T.);
#13320=ORIENTED_EDGE('',*,*,#9941,.T.);
#13321=ORIENTED_EDGE('',*,*,#9942,.T.);
#13322=ORIENTED_EDGE('',*,*,#9938,.F.);
#13323=ORIENTED_EDGE('',*,*,#9943,.T.);
#13324=ORIENTED_EDGE('',*,*,#9944,.T.);
#13325=ORIENTED_EDGE('',*,*,#9945,.T.);
#13326=ORIENTED_EDGE('',*,*,#9941,.F.);
#13327=ORIENTED_EDGE('',*,*,#9946,.T.);
#13328=ORIENTED_EDGE('',*,*,#9947,.T.);
#13329=ORIENTED_EDGE('',*,*,#9948,.T.);
#13330=ORIENTED_EDGE('',*,*,#9944,.F.);
#13331=ORIENTED_EDGE('',*,*,#9949,.T.);
#13332=ORIENTED_EDGE('',*,*,#9950,.T.);
#13333=ORIENTED_EDGE('',*,*,#9951,.T.);
#13334=ORIENTED_EDGE('',*,*,#9947,.F.);
#13335=ORIENTED_EDGE('',*,*,#9952,.T.);
#13336=ORIENTED_EDGE('',*,*,#9953,.F.);
#13337=ORIENTED_EDGE('',*,*,#9954,.T.);
#13338=ORIENTED_EDGE('',*,*,#9955,.F.);
#13339=ORIENTED_EDGE('',*,*,#9956,.T.);
#13340=ORIENTED_EDGE('',*,*,#9957,.T.);
#13341=ORIENTED_EDGE('',*,*,#9958,.T.);
#13342=ORIENTED_EDGE('',*,*,#9959,.F.);
#13343=ORIENTED_EDGE('',*,*,#9960,.T.);
#13344=ORIENTED_EDGE('',*,*,#9961,.T.);
#13345=ORIENTED_EDGE('',*,*,#9962,.T.);
#13346=ORIENTED_EDGE('',*,*,#9957,.F.);
#13347=ORIENTED_EDGE('',*,*,#9963,.T.);
#13348=ORIENTED_EDGE('',*,*,#9964,.T.);
#13349=ORIENTED_EDGE('',*,*,#9965,.T.);
#13350=ORIENTED_EDGE('',*,*,#9961,.F.);
#13351=ORIENTED_EDGE('',*,*,#9966,.T.);
#13352=ORIENTED_EDGE('',*,*,#9967,.T.);
#13353=ORIENTED_EDGE('',*,*,#9968,.T.);
#13354=ORIENTED_EDGE('',*,*,#9964,.F.);
#13355=ORIENTED_EDGE('',*,*,#9969,.T.);
#13356=ORIENTED_EDGE('',*,*,#9970,.T.);
#13357=ORIENTED_EDGE('',*,*,#9971,.T.);
#13358=ORIENTED_EDGE('',*,*,#9967,.F.);
#13359=ORIENTED_EDGE('',*,*,#9972,.T.);
#13360=ORIENTED_EDGE('',*,*,#9973,.T.);
#13361=ORIENTED_EDGE('',*,*,#9974,.T.);
#13362=ORIENTED_EDGE('',*,*,#9970,.F.);
#13363=ORIENTED_EDGE('',*,*,#9975,.T.);
#13364=ORIENTED_EDGE('',*,*,#9976,.T.);
#13365=ORIENTED_EDGE('',*,*,#9977,.T.);
#13366=ORIENTED_EDGE('',*,*,#9973,.F.);
#13367=ORIENTED_EDGE('',*,*,#9978,.T.);
#13368=ORIENTED_EDGE('',*,*,#9979,.F.);
#13369=ORIENTED_EDGE('',*,*,#9980,.T.);
#13370=ORIENTED_EDGE('',*,*,#9981,.F.);
#13371=ORIENTED_EDGE('',*,*,#9982,.T.);
#13372=ORIENTED_EDGE('',*,*,#9983,.T.);
#13373=ORIENTED_EDGE('',*,*,#9984,.T.);
#13374=ORIENTED_EDGE('',*,*,#9985,.F.);
#13375=ORIENTED_EDGE('',*,*,#9986,.F.);
#13376=ORIENTED_EDGE('',*,*,#9987,.T.);
#13377=ORIENTED_EDGE('',*,*,#9988,.T.);
#13378=ORIENTED_EDGE('',*,*,#9983,.F.);
#13379=ORIENTED_EDGE('',*,*,#9989,.F.);
#13380=ORIENTED_EDGE('',*,*,#9990,.T.);
#13381=ORIENTED_EDGE('',*,*,#9991,.T.);
#13382=ORIENTED_EDGE('',*,*,#9987,.F.);
#13383=ORIENTED_EDGE('',*,*,#9992,.F.);
#13384=ORIENTED_EDGE('',*,*,#9993,.T.);
#13385=ORIENTED_EDGE('',*,*,#9994,.T.);
#13386=ORIENTED_EDGE('',*,*,#9990,.F.);
#13387=ORIENTED_EDGE('',*,*,#9995,.F.);
#13388=ORIENTED_EDGE('',*,*,#9996,.T.);
#13389=ORIENTED_EDGE('',*,*,#9997,.T.);
#13390=ORIENTED_EDGE('',*,*,#9993,.F.);
#13391=ORIENTED_EDGE('',*,*,#9998,.F.);
#13392=ORIENTED_EDGE('',*,*,#9999,.T.);
#13393=ORIENTED_EDGE('',*,*,#10000,.T.);
#13394=ORIENTED_EDGE('',*,*,#9996,.F.);
#13395=ORIENTED_EDGE('',*,*,#10001,.F.);
#13396=ORIENTED_EDGE('',*,*,#10002,.T.);
#13397=ORIENTED_EDGE('',*,*,#10003,.T.);
#13398=ORIENTED_EDGE('',*,*,#9999,.F.);
#13399=ORIENTED_EDGE('',*,*,#10004,.F.);
#13400=ORIENTED_EDGE('',*,*,#10005,.F.);
#13401=ORIENTED_EDGE('',*,*,#10006,.F.);
#13402=ORIENTED_EDGE('',*,*,#10007,.F.);
#13403=ORIENTED_EDGE('',*,*,#10008,.T.);
#13404=ORIENTED_EDGE('',*,*,#10009,.T.);
#13405=ORIENTED_EDGE('',*,*,#10010,.T.);
#13406=ORIENTED_EDGE('',*,*,#10011,.F.);
#13407=ORIENTED_EDGE('',*,*,#10012,.F.);
#13408=ORIENTED_EDGE('',*,*,#10013,.T.);
#13409=ORIENTED_EDGE('',*,*,#10014,.T.);
#13410=ORIENTED_EDGE('',*,*,#10009,.F.);
#13411=ORIENTED_EDGE('',*,*,#10015,.F.);
#13412=ORIENTED_EDGE('',*,*,#10016,.T.);
#13413=ORIENTED_EDGE('',*,*,#10017,.T.);
#13414=ORIENTED_EDGE('',*,*,#10013,.F.);
#13415=ORIENTED_EDGE('',*,*,#10018,.F.);
#13416=ORIENTED_EDGE('',*,*,#10019,.T.);
#13417=ORIENTED_EDGE('',*,*,#10020,.T.);
#13418=ORIENTED_EDGE('',*,*,#10016,.F.);
#13419=ORIENTED_EDGE('',*,*,#10021,.F.);
#13420=ORIENTED_EDGE('',*,*,#10022,.T.);
#13421=ORIENTED_EDGE('',*,*,#10023,.T.);
#13422=ORIENTED_EDGE('',*,*,#10019,.F.);
#13423=ORIENTED_EDGE('',*,*,#10024,.F.);
#13424=ORIENTED_EDGE('',*,*,#10025,.T.);
#13425=ORIENTED_EDGE('',*,*,#10026,.T.);
#13426=ORIENTED_EDGE('',*,*,#10022,.F.);
#13427=ORIENTED_EDGE('',*,*,#10027,.F.);
#13428=ORIENTED_EDGE('',*,*,#10028,.T.);
#13429=ORIENTED_EDGE('',*,*,#10029,.T.);
#13430=ORIENTED_EDGE('',*,*,#10025,.F.);
#13431=ORIENTED_EDGE('',*,*,#10030,.F.);
#13432=ORIENTED_EDGE('',*,*,#10031,.F.);
#13433=ORIENTED_EDGE('',*,*,#10032,.F.);
#13434=ORIENTED_EDGE('',*,*,#10033,.F.);
#13435=ORIENTED_EDGE('',*,*,#10034,.T.);
#13436=ORIENTED_EDGE('',*,*,#10035,.T.);
#13437=ORIENTED_EDGE('',*,*,#10036,.T.);
#13438=ORIENTED_EDGE('',*,*,#10037,.F.);
#13439=ORIENTED_EDGE('',*,*,#10038,.F.);
#13440=ORIENTED_EDGE('',*,*,#10039,.T.);
#13441=ORIENTED_EDGE('',*,*,#10040,.T.);
#13442=ORIENTED_EDGE('',*,*,#10035,.F.);
#13443=ORIENTED_EDGE('',*,*,#10041,.F.);
#13444=ORIENTED_EDGE('',*,*,#10042,.T.);
#13445=ORIENTED_EDGE('',*,*,#10043,.T.);
#13446=ORIENTED_EDGE('',*,*,#10039,.F.);
#13447=ORIENTED_EDGE('',*,*,#10044,.F.);
#13448=ORIENTED_EDGE('',*,*,#10045,.T.);
#13449=ORIENTED_EDGE('',*,*,#10046,.T.);
#13450=ORIENTED_EDGE('',*,*,#10042,.F.);
#13451=ORIENTED_EDGE('',*,*,#10047,.F.);
#13452=ORIENTED_EDGE('',*,*,#10048,.T.);
#13453=ORIENTED_EDGE('',*,*,#10049,.T.);
#13454=ORIENTED_EDGE('',*,*,#10045,.F.);
#13455=ORIENTED_EDGE('',*,*,#10050,.F.);
#13456=ORIENTED_EDGE('',*,*,#10051,.T.);
#13457=ORIENTED_EDGE('',*,*,#10052,.T.);
#13458=ORIENTED_EDGE('',*,*,#10048,.F.);
#13459=ORIENTED_EDGE('',*,*,#10053,.F.);
#13460=ORIENTED_EDGE('',*,*,#10054,.T.);
#13461=ORIENTED_EDGE('',*,*,#10055,.T.);
#13462=ORIENTED_EDGE('',*,*,#10051,.F.);
#13463=ORIENTED_EDGE('',*,*,#10056,.F.);
#13464=ORIENTED_EDGE('',*,*,#10057,.F.);
#13465=ORIENTED_EDGE('',*,*,#10058,.F.);
#13466=ORIENTED_EDGE('',*,*,#10059,.F.);
#13467=ORIENTED_EDGE('',*,*,#10060,.T.);
#13468=ORIENTED_EDGE('',*,*,#10061,.T.);
#13469=ORIENTED_EDGE('',*,*,#10062,.T.);
#13470=ORIENTED_EDGE('',*,*,#10063,.F.);
#13471=ORIENTED_EDGE('',*,*,#10064,.F.);
#13472=ORIENTED_EDGE('',*,*,#10065,.T.);
#13473=ORIENTED_EDGE('',*,*,#10066,.T.);
#13474=ORIENTED_EDGE('',*,*,#10061,.F.);
#13475=ORIENTED_EDGE('',*,*,#10067,.F.);
#13476=ORIENTED_EDGE('',*,*,#10068,.T.);
#13477=ORIENTED_EDGE('',*,*,#10069,.T.);
#13478=ORIENTED_EDGE('',*,*,#10065,.F.);
#13479=ORIENTED_EDGE('',*,*,#10070,.F.);
#13480=ORIENTED_EDGE('',*,*,#10071,.T.);
#13481=ORIENTED_EDGE('',*,*,#10072,.T.);
#13482=ORIENTED_EDGE('',*,*,#10068,.F.);
#13483=ORIENTED_EDGE('',*,*,#10073,.F.);
#13484=ORIENTED_EDGE('',*,*,#10074,.T.);
#13485=ORIENTED_EDGE('',*,*,#10075,.T.);
#13486=ORIENTED_EDGE('',*,*,#10071,.F.);
#13487=ORIENTED_EDGE('',*,*,#10076,.F.);
#13488=ORIENTED_EDGE('',*,*,#10077,.T.);
#13489=ORIENTED_EDGE('',*,*,#10078,.T.);
#13490=ORIENTED_EDGE('',*,*,#10074,.F.);
#13491=ORIENTED_EDGE('',*,*,#10079,.F.);
#13492=ORIENTED_EDGE('',*,*,#10080,.T.);
#13493=ORIENTED_EDGE('',*,*,#10081,.T.);
#13494=ORIENTED_EDGE('',*,*,#10077,.F.);
#13495=ORIENTED_EDGE('',*,*,#10082,.F.);
#13496=ORIENTED_EDGE('',*,*,#10083,.F.);
#13497=ORIENTED_EDGE('',*,*,#10084,.F.);
#13498=ORIENTED_EDGE('',*,*,#10085,.F.);
#13499=ORIENTED_EDGE('',*,*,#10086,.T.);
#13500=ORIENTED_EDGE('',*,*,#10083,.T.);
#13501=ORIENTED_EDGE('',*,*,#10087,.T.);
#13502=ORIENTED_EDGE('',*,*,#10080,.F.);
#13503=ORIENTED_EDGE('',*,*,#10088,.F.);
#13504=ORIENTED_EDGE('',*,*,#10089,.F.);
#13505=ORIENTED_EDGE('',*,*,#10062,.F.);
#13506=ORIENTED_EDGE('',*,*,#10066,.F.);
#13507=ORIENTED_EDGE('',*,*,#10069,.F.);
#13508=ORIENTED_EDGE('',*,*,#10072,.F.);
#13509=ORIENTED_EDGE('',*,*,#10075,.F.);
#13510=ORIENTED_EDGE('',*,*,#10078,.F.);
#13511=ORIENTED_EDGE('',*,*,#10081,.F.);
#13512=ORIENTED_EDGE('',*,*,#10087,.F.);
#13513=ORIENTED_EDGE('',*,*,#10086,.F.);
#13514=ORIENTED_EDGE('',*,*,#10090,.F.);
#13515=ORIENTED_EDGE('',*,*,#9902,.F.);
#13516=ORIENTED_EDGE('',*,*,#10091,.F.);
#13517=ORIENTED_EDGE('',*,*,#9900,.F.);
#13518=ORIENTED_EDGE('',*,*,#9897,.F.);
#13519=ORIENTED_EDGE('',*,*,#9894,.F.);
#13520=ORIENTED_EDGE('',*,*,#9891,.F.);
#13521=ORIENTED_EDGE('',*,*,#9888,.F.);
#13522=ORIENTED_EDGE('',*,*,#9885,.F.);
#13523=ORIENTED_EDGE('',*,*,#9882,.F.);
#13524=ORIENTED_EDGE('',*,*,#10092,.F.);
#13525=ORIENTED_EDGE('',*,*,#9880,.F.);
#13526=ORIENTED_EDGE('',*,*,#9884,.F.);
#13527=ORIENTED_EDGE('',*,*,#9887,.F.);
#13528=ORIENTED_EDGE('',*,*,#9890,.F.);
#13529=ORIENTED_EDGE('',*,*,#9893,.F.);
#13530=ORIENTED_EDGE('',*,*,#9896,.F.);
#13531=ORIENTED_EDGE('',*,*,#9899,.F.);
#13532=ORIENTED_EDGE('',*,*,#10093,.F.);
#13533=ORIENTED_EDGE('',*,*,#9904,.F.);
#13534=ORIENTED_EDGE('',*,*,#10094,.F.);
#13535=ORIENTED_EDGE('',*,*,#10084,.T.);
#13536=ORIENTED_EDGE('',*,*,#10088,.T.);
#13537=ORIENTED_EDGE('',*,*,#10082,.T.);
#13538=ORIENTED_EDGE('',*,*,#10079,.T.);
#13539=ORIENTED_EDGE('',*,*,#10076,.T.);
#13540=ORIENTED_EDGE('',*,*,#10073,.T.);
#13541=ORIENTED_EDGE('',*,*,#10070,.T.);
#13542=ORIENTED_EDGE('',*,*,#10067,.T.);
#13543=ORIENTED_EDGE('',*,*,#10064,.T.);
#13544=ORIENTED_EDGE('',*,*,#10095,.T.);
#13545=ORIENTED_EDGE('',*,*,#10096,.T.);
#13546=ORIENTED_EDGE('',*,*,#10097,.T.);
#13547=ORIENTED_EDGE('',*,*,#10098,.T.);
#13548=ORIENTED_EDGE('',*,*,#10099,.T.);
#13549=ORIENTED_EDGE('',*,*,#10033,.T.);
#13550=ORIENTED_EDGE('',*,*,#10100,.T.);
#13551=ORIENTED_EDGE('',*,*,#9981,.T.);
#13552=ORIENTED_EDGE('',*,*,#10101,.T.);
#13553=ORIENTED_EDGE('',*,*,#10059,.T.);
#13554=ORIENTED_EDGE('',*,*,#10102,.T.);
#13555=ORIENTED_EDGE('',*,*,#9955,.T.);
#13556=ORIENTED_EDGE('',*,*,#10103,.T.);
#13557=ORIENTED_EDGE('',*,*,#10007,.T.);
#13558=ORIENTED_EDGE('',*,*,#10104,.T.);
#13559=ORIENTED_EDGE('',*,*,#9929,.T.);
#13560=ORIENTED_EDGE('',*,*,#10090,.T.);
#13561=ORIENTED_EDGE('',*,*,#10085,.T.);
#13562=ORIENTED_EDGE('',*,*,#10094,.T.);
#13563=ORIENTED_EDGE('',*,*,#9903,.T.);
#13564=ORIENTED_EDGE('',*,*,#10057,.T.);
#13565=ORIENTED_EDGE('',*,*,#10105,.T.);
#13566=ORIENTED_EDGE('',*,*,#10054,.F.);
#13567=ORIENTED_EDGE('',*,*,#10106,.F.);
#13568=ORIENTED_EDGE('',*,*,#10107,.F.);
#13569=ORIENTED_EDGE('',*,*,#10036,.F.);
#13570=ORIENTED_EDGE('',*,*,#10040,.F.);
#13571=ORIENTED_EDGE('',*,*,#10043,.F.);
#13572=ORIENTED_EDGE('',*,*,#10046,.F.);
#13573=ORIENTED_EDGE('',*,*,#10049,.F.);
#13574=ORIENTED_EDGE('',*,*,#10052,.F.);
#13575=ORIENTED_EDGE('',*,*,#10055,.F.);
#13576=ORIENTED_EDGE('',*,*,#10105,.F.);
#13577=ORIENTED_EDGE('',*,*,#10060,.F.);
#13578=ORIENTED_EDGE('',*,*,#10101,.F.);
#13579=ORIENTED_EDGE('',*,*,#9954,.F.);
#13580=ORIENTED_EDGE('',*,*,#10108,.F.);
#13581=ORIENTED_EDGE('',*,*,#9952,.F.);
#13582=ORIENTED_EDGE('',*,*,#9949,.F.);
#13583=ORIENTED_EDGE('',*,*,#9946,.F.);
#13584=ORIENTED_EDGE('',*,*,#9943,.F.);
#13585=ORIENTED_EDGE('',*,*,#9940,.F.);
#13586=ORIENTED_EDGE('',*,*,#9937,.F.);
#13587=ORIENTED_EDGE('',*,*,#9934,.F.);
#13588=ORIENTED_EDGE('',*,*,#10109,.F.);
#13589=ORIENTED_EDGE('',*,*,#9932,.F.);
#13590=ORIENTED_EDGE('',*,*,#9936,.F.);
#13591=ORIENTED_EDGE('',*,*,#9939,.F.);
#13592=ORIENTED_EDGE('',*,*,#9942,.F.);
#13593=ORIENTED_EDGE('',*,*,#9945,.F.);
#13594=ORIENTED_EDGE('',*,*,#9948,.F.);
#13595=ORIENTED_EDGE('',*,*,#9951,.F.);
#13596=ORIENTED_EDGE('',*,*,#10110,.F.);
#13597=ORIENTED_EDGE('',*,*,#9956,.F.);
#13598=ORIENTED_EDGE('',*,*,#10102,.F.);
#13599=ORIENTED_EDGE('',*,*,#10058,.T.);
#13600=ORIENTED_EDGE('',*,*,#10106,.T.);
#13601=ORIENTED_EDGE('',*,*,#10056,.T.);
#13602=ORIENTED_EDGE('',*,*,#10053,.T.);
#13603=ORIENTED_EDGE('',*,*,#10050,.T.);
#13604=ORIENTED_EDGE('',*,*,#10047,.T.);
#13605=ORIENTED_EDGE('',*,*,#10044,.T.);
#13606=ORIENTED_EDGE('',*,*,#10041,.T.);
#13607=ORIENTED_EDGE('',*,*,#10038,.T.);
#13608=ORIENTED_EDGE('',*,*,#10031,.T.);
#13609=ORIENTED_EDGE('',*,*,#10111,.T.);
#13610=ORIENTED_EDGE('',*,*,#10028,.F.);
#13611=ORIENTED_EDGE('',*,*,#10112,.F.);
#13612=ORIENTED_EDGE('',*,*,#10113,.F.);
#13613=ORIENTED_EDGE('',*,*,#10010,.F.);
#13614=ORIENTED_EDGE('',*,*,#10014,.F.);
#13615=ORIENTED_EDGE('',*,*,#10017,.F.);
#13616=ORIENTED_EDGE('',*,*,#10020,.F.);
#13617=ORIENTED_EDGE('',*,*,#10023,.F.);
#13618=ORIENTED_EDGE('',*,*,#10026,.F.);
#13619=ORIENTED_EDGE('',*,*,#10029,.F.);
#13620=ORIENTED_EDGE('',*,*,#10111,.F.);
#13621=ORIENTED_EDGE('',*,*,#10034,.F.);
#13622=ORIENTED_EDGE('',*,*,#10099,.F.);
#13623=ORIENTED_EDGE('',*,*,#9980,.F.);
#13624=ORIENTED_EDGE('',*,*,#10114,.F.);
#13625=ORIENTED_EDGE('',*,*,#9978,.F.);
#13626=ORIENTED_EDGE('',*,*,#9975,.F.);
#13627=ORIENTED_EDGE('',*,*,#9972,.F.);
#13628=ORIENTED_EDGE('',*,*,#9969,.F.);
#13629=ORIENTED_EDGE('',*,*,#9966,.F.);
#13630=ORIENTED_EDGE('',*,*,#9963,.F.);
#13631=ORIENTED_EDGE('',*,*,#9960,.F.);
#13632=ORIENTED_EDGE('',*,*,#10115,.F.);
#13633=ORIENTED_EDGE('',*,*,#9958,.F.);
#13634=ORIENTED_EDGE('',*,*,#9962,.F.);
#13635=ORIENTED_EDGE('',*,*,#9965,.F.);
#13636=ORIENTED_EDGE('',*,*,#9968,.F.);
#13637=ORIENTED_EDGE('',*,*,#9971,.F.);
#13638=ORIENTED_EDGE('',*,*,#9974,.F.);
#13639=ORIENTED_EDGE('',*,*,#9977,.F.);
#13640=ORIENTED_EDGE('',*,*,#10116,.F.);
#13641=ORIENTED_EDGE('',*,*,#9982,.F.);
#13642=ORIENTED_EDGE('',*,*,#10100,.F.);
#13643=ORIENTED_EDGE('',*,*,#10032,.T.);
#13644=ORIENTED_EDGE('',*,*,#10112,.T.);
#13645=ORIENTED_EDGE('',*,*,#10030,.T.);
#13646=ORIENTED_EDGE('',*,*,#10027,.T.);
#13647=ORIENTED_EDGE('',*,*,#10024,.T.);
#13648=ORIENTED_EDGE('',*,*,#10021,.T.);
#13649=ORIENTED_EDGE('',*,*,#10018,.T.);
#13650=ORIENTED_EDGE('',*,*,#10015,.T.);
#13651=ORIENTED_EDGE('',*,*,#10012,.T.);
#13652=ORIENTED_EDGE('',*,*,#10005,.T.);
#13653=ORIENTED_EDGE('',*,*,#10117,.T.);
#13654=ORIENTED_EDGE('',*,*,#10002,.F.);
#13655=ORIENTED_EDGE('',*,*,#10118,.F.);
#13656=ORIENTED_EDGE('',*,*,#10119,.F.);
#13657=ORIENTED_EDGE('',*,*,#9984,.F.);
#13658=ORIENTED_EDGE('',*,*,#9988,.F.);
#13659=ORIENTED_EDGE('',*,*,#9991,.F.);
#13660=ORIENTED_EDGE('',*,*,#9994,.F.);
#13661=ORIENTED_EDGE('',*,*,#9997,.F.);
#13662=ORIENTED_EDGE('',*,*,#10000,.F.);
#13663=ORIENTED_EDGE('',*,*,#10003,.F.);
#13664=ORIENTED_EDGE('',*,*,#10117,.F.);
#13665=ORIENTED_EDGE('',*,*,#10008,.F.);
#13666=ORIENTED_EDGE('',*,*,#10103,.F.);
#13667=ORIENTED_EDGE('',*,*,#9928,.F.);
#13668=ORIENTED_EDGE('',*,*,#10120,.F.);
#13669=ORIENTED_EDGE('',*,*,#9926,.F.);
#13670=ORIENTED_EDGE('',*,*,#9923,.F.);
#13671=ORIENTED_EDGE('',*,*,#9920,.F.);
#13672=ORIENTED_EDGE('',*,*,#9917,.F.);
#13673=ORIENTED_EDGE('',*,*,#9914,.F.);
#13674=ORIENTED_EDGE('',*,*,#9911,.F.);
#13675=ORIENTED_EDGE('',*,*,#9908,.F.);
#13676=ORIENTED_EDGE('',*,*,#10121,.F.);
#13677=ORIENTED_EDGE('',*,*,#9906,.F.);
#13678=ORIENTED_EDGE('',*,*,#9910,.F.);
#13679=ORIENTED_EDGE('',*,*,#9913,.F.);
#13680=ORIENTED_EDGE('',*,*,#9916,.F.);
#13681=ORIENTED_EDGE('',*,*,#9919,.F.);
#13682=ORIENTED_EDGE('',*,*,#9922,.F.);
#13683=ORIENTED_EDGE('',*,*,#9925,.F.);
#13684=ORIENTED_EDGE('',*,*,#10122,.F.);
#13685=ORIENTED_EDGE('',*,*,#9930,.F.);
#13686=ORIENTED_EDGE('',*,*,#10104,.F.);
#13687=ORIENTED_EDGE('',*,*,#10006,.T.);
#13688=ORIENTED_EDGE('',*,*,#10118,.T.);
#13689=ORIENTED_EDGE('',*,*,#10004,.T.);
#13690=ORIENTED_EDGE('',*,*,#10001,.T.);
#13691=ORIENTED_EDGE('',*,*,#9998,.T.);
#13692=ORIENTED_EDGE('',*,*,#9995,.T.);
#13693=ORIENTED_EDGE('',*,*,#9992,.T.);
#13694=ORIENTED_EDGE('',*,*,#9989,.T.);
#13695=ORIENTED_EDGE('',*,*,#9986,.T.);
#13696=ORIENTED_EDGE('',*,*,#9979,.T.);
#13697=ORIENTED_EDGE('',*,*,#10116,.T.);
#13698=ORIENTED_EDGE('',*,*,#9976,.F.);
#13699=ORIENTED_EDGE('',*,*,#10114,.T.);
#13700=ORIENTED_EDGE('',*,*,#9953,.T.);
#13701=ORIENTED_EDGE('',*,*,#10110,.T.);
#13702=ORIENTED_EDGE('',*,*,#9950,.F.);
#13703=ORIENTED_EDGE('',*,*,#10108,.T.);
#13704=ORIENTED_EDGE('',*,*,#9927,.T.);
#13705=ORIENTED_EDGE('',*,*,#10122,.T.);
#13706=ORIENTED_EDGE('',*,*,#9924,.F.);
#13707=ORIENTED_EDGE('',*,*,#10120,.T.);
#13708=ORIENTED_EDGE('',*,*,#9901,.T.);
#13709=ORIENTED_EDGE('',*,*,#10093,.T.);
#13710=ORIENTED_EDGE('',*,*,#9898,.F.);
#13711=ORIENTED_EDGE('',*,*,#10091,.T.);
#13712=ORIENTED_EDGE('',*,*,#10123,.T.);
#13713=ORIENTED_EDGE('',*,*,#10124,.T.);
#13714=ORIENTED_EDGE('',*,*,#10098,.F.);
#13715=ORIENTED_EDGE('',*,*,#10125,.F.);
#13716=ORIENTED_EDGE('',*,*,#10126,.T.);
#13717=ORIENTED_EDGE('',*,*,#10125,.T.);
#13718=ORIENTED_EDGE('',*,*,#10097,.F.);
#13719=ORIENTED_EDGE('',*,*,#10127,.F.);
#13720=ORIENTED_EDGE('',*,*,#10128,.T.);
#13721=ORIENTED_EDGE('',*,*,#10127,.T.);
#13722=ORIENTED_EDGE('',*,*,#10096,.F.);
#13723=ORIENTED_EDGE('',*,*,#10129,.F.);
#13724=ORIENTED_EDGE('',*,*,#10130,.T.);
#13725=ORIENTED_EDGE('',*,*,#10129,.T.);
#13726=ORIENTED_EDGE('',*,*,#10095,.F.);
#13727=ORIENTED_EDGE('',*,*,#10124,.F.);
#13728=ORIENTED_EDGE('',*,*,#10130,.F.);
#13729=ORIENTED_EDGE('',*,*,#10123,.F.);
#13730=ORIENTED_EDGE('',*,*,#10126,.F.);
#13731=ORIENTED_EDGE('',*,*,#10128,.F.);
#13732=ORIENTED_EDGE('',*,*,#10089,.T.);
#13733=ORIENTED_EDGE('',*,*,#9881,.T.);
#13734=ORIENTED_EDGE('',*,*,#10092,.T.);
#13735=ORIENTED_EDGE('',*,*,#10063,.T.);
#13736=ORIENTED_EDGE('',*,*,#10107,.T.);
#13737=ORIENTED_EDGE('',*,*,#9933,.T.);
#13738=ORIENTED_EDGE('',*,*,#10109,.T.);
#13739=ORIENTED_EDGE('',*,*,#10037,.T.);
#13740=ORIENTED_EDGE('',*,*,#10113,.T.);
#13741=ORIENTED_EDGE('',*,*,#9959,.T.);
#13742=ORIENTED_EDGE('',*,*,#10115,.T.);
#13743=ORIENTED_EDGE('',*,*,#10011,.T.);
#13744=ORIENTED_EDGE('',*,*,#10119,.T.);
#13745=ORIENTED_EDGE('',*,*,#9907,.T.);
#13746=ORIENTED_EDGE('',*,*,#10121,.T.);
#13747=ORIENTED_EDGE('',*,*,#9985,.T.);
#19716=CYLINDRICAL_SURFACE('',#22083,3.5175);
#19717=CYLINDRICAL_SURFACE('',#22085,3.5175);
#19718=CYLINDRICAL_SURFACE('',#22086,3.5175);
#19719=CYLINDRICAL_SURFACE('',#22087,3.5175);
#19720=CYLINDRICAL_SURFACE('',#22088,3.5175);
#19721=CYLINDRICAL_SURFACE('',#22089,3.5175);
#19722=CYLINDRICAL_SURFACE('',#22090,3.5175);
#19723=CYLINDRICAL_SURFACE('',#22091,3.5175);
#19724=CYLINDRICAL_SURFACE('',#22093,3.5175);
#19725=CYLINDRICAL_SURFACE('',#22095,3.5175);
#19726=CYLINDRICAL_SURFACE('',#22096,3.5175);
#19727=CYLINDRICAL_SURFACE('',#22097,3.5175);
#19728=CYLINDRICAL_SURFACE('',#22098,3.5175);
#19729=CYLINDRICAL_SURFACE('',#22099,3.5175);
#19730=CYLINDRICAL_SURFACE('',#22100,3.5175);
#19731=CYLINDRICAL_SURFACE('',#22101,3.5175);
#19732=CYLINDRICAL_SURFACE('',#22103,3.5175);
#19733=CYLINDRICAL_SURFACE('',#22105,3.5175);
#19734=CYLINDRICAL_SURFACE('',#22106,3.5175);
#19735=CYLINDRICAL_SURFACE('',#22107,3.5175);
#19736=CYLINDRICAL_SURFACE('',#22108,3.5175);
#19737=CYLINDRICAL_SURFACE('',#22109,3.5175);
#19738=CYLINDRICAL_SURFACE('',#22110,3.5175);
#19739=CYLINDRICAL_SURFACE('',#22111,3.5175);
#19740=CYLINDRICAL_SURFACE('',#22113,3.5175);
#19741=CYLINDRICAL_SURFACE('',#22115,3.5175);
#19742=CYLINDRICAL_SURFACE('',#22116,3.5175);
#19743=CYLINDRICAL_SURFACE('',#22117,3.5175);
#19744=CYLINDRICAL_SURFACE('',#22118,3.5175);
#19745=CYLINDRICAL_SURFACE('',#22119,3.5175);
#19746=CYLINDRICAL_SURFACE('',#22120,3.5175);
#19747=CYLINDRICAL_SURFACE('',#22121,3.5175);
#19748=CYLINDRICAL_SURFACE('',#22123,4.07350000000001);
#19749=CYLINDRICAL_SURFACE('',#22125,4.07350000000001);
#19750=CYLINDRICAL_SURFACE('',#22126,4.07350000000001);
#19751=CYLINDRICAL_SURFACE('',#22127,4.07350000000001);
#19752=CYLINDRICAL_SURFACE('',#22128,4.07350000000001);
#19753=CYLINDRICAL_SURFACE('',#22129,4.07350000000001);
#19754=CYLINDRICAL_SURFACE('',#22130,4.07350000000001);
#19755=CYLINDRICAL_SURFACE('',#22131,4.07350000000001);
#19756=CYLINDRICAL_SURFACE('',#22133,4.0735);
#19757=CYLINDRICAL_SURFACE('',#22135,4.0735);
#19758=CYLINDRICAL_SURFACE('',#22136,4.0735);
#19759=CYLINDRICAL_SURFACE('',#22137,4.0735);
#19760=CYLINDRICAL_SURFACE('',#22138,4.0735);
#19761=CYLINDRICAL_SURFACE('',#22139,4.0735);
#19762=CYLINDRICAL_SURFACE('',#22140,4.0735);
#19763=CYLINDRICAL_SURFACE('',#22141,4.0735);
#19764=CYLINDRICAL_SURFACE('',#22143,4.0735);
#19765=CYLINDRICAL_SURFACE('',#22145,4.0735);
#19766=CYLINDRICAL_SURFACE('',#22146,4.0735);
#19767=CYLINDRICAL_SURFACE('',#22147,4.0735);
#19768=CYLINDRICAL_SURFACE('',#22148,4.0735);
#19769=CYLINDRICAL_SURFACE('',#22149,4.0735);
#19770=CYLINDRICAL_SURFACE('',#22150,4.0735);
#19771=CYLINDRICAL_SURFACE('',#22151,4.0735);
#19772=CYLINDRICAL_SURFACE('',#22153,4.07350000000001);
#19773=CYLINDRICAL_SURFACE('',#22155,4.07350000000001);
#19774=CYLINDRICAL_SURFACE('',#22156,4.07350000000001);
#19775=CYLINDRICAL_SURFACE('',#22157,4.07350000000001);
#19776=CYLINDRICAL_SURFACE('',#22158,4.07350000000001);
#19777=CYLINDRICAL_SURFACE('',#22159,4.07350000000001);
#19778=CYLINDRICAL_SURFACE('',#22160,4.07350000000001);
#19779=CYLINDRICAL_SURFACE('',#22161,4.07350000000001);
#19780=CYLINDRICAL_SURFACE('',#22163,4.07350000000001);
#19781=CYLINDRICAL_SURFACE('',#22165,4.0735);
#19782=CYLINDRICAL_SURFACE('',#22166,4.0735);
#19783=CYLINDRICAL_SURFACE('',#22167,4.07350000000001);
#19784=CYLINDRICAL_SURFACE('',#22168,3.5175);
#19785=CYLINDRICAL_SURFACE('',#22169,3.5175);
#19786=CYLINDRICAL_SURFACE('',#22170,3.5175);
#19787=CYLINDRICAL_SURFACE('',#22171,3.5175);
#20683=ADVANCED_FACE('',(#2563),#19716,.F.);
#20684=ADVANCED_FACE('',(#2564),#19717,.F.);
#20685=ADVANCED_FACE('',(#2565),#19718,.F.);
#20686=ADVANCED_FACE('',(#2566),#19719,.F.);
#20687=ADVANCED_FACE('',(#2567),#19720,.F.);
#20688=ADVANCED_FACE('',(#2568),#19721,.F.);
#20689=ADVANCED_FACE('',(#2569),#19722,.F.);
#20690=ADVANCED_FACE('',(#2570),#19723,.F.);
#20691=ADVANCED_FACE('',(#2571),#19724,.F.);
#20692=ADVANCED_FACE('',(#2572),#19725,.F.);
#20693=ADVANCED_FACE('',(#2573),#19726,.F.);
#20694=ADVANCED_FACE('',(#2574),#19727,.F.);
#20695=ADVANCED_FACE('',(#2575),#19728,.F.);
#20696=ADVANCED_FACE('',(#2576),#19729,.F.);
#20697=ADVANCED_FACE('',(#2577),#19730,.F.);
#20698=ADVANCED_FACE('',(#2578),#19731,.F.);
#20699=ADVANCED_FACE('',(#2579),#19732,.F.);
#20700=ADVANCED_FACE('',(#2580),#19733,.F.);
#20701=ADVANCED_FACE('',(#2581),#19734,.F.);
#20702=ADVANCED_FACE('',(#2582),#19735,.F.);
#20703=ADVANCED_FACE('',(#2583),#19736,.F.);
#20704=ADVANCED_FACE('',(#2584),#19737,.F.);
#20705=ADVANCED_FACE('',(#2585),#19738,.F.);
#20706=ADVANCED_FACE('',(#2586),#19739,.F.);
#20707=ADVANCED_FACE('',(#2587),#19740,.F.);
#20708=ADVANCED_FACE('',(#2588),#19741,.F.);
#20709=ADVANCED_FACE('',(#2589),#19742,.F.);
#20710=ADVANCED_FACE('',(#2590),#19743,.F.);
#20711=ADVANCED_FACE('',(#2591),#19744,.F.);
#20712=ADVANCED_FACE('',(#2592),#19745,.F.);
#20713=ADVANCED_FACE('',(#2593),#19746,.F.);
#20714=ADVANCED_FACE('',(#2594),#19747,.F.);
#20715=ADVANCED_FACE('',(#2595),#19748,.F.);
#20716=ADVANCED_FACE('',(#2596),#19749,.F.);
#20717=ADVANCED_FACE('',(#2597),#19750,.F.);
#20718=ADVANCED_FACE('',(#2598),#19751,.F.);
#20719=ADVANCED_FACE('',(#2599),#19752,.F.);
#20720=ADVANCED_FACE('',(#2600),#19753,.F.);
#20721=ADVANCED_FACE('',(#2601),#19754,.F.);
#20722=ADVANCED_FACE('',(#2602),#19755,.F.);
#20723=ADVANCED_FACE('',(#2603),#19756,.F.);
#20724=ADVANCED_FACE('',(#2604),#19757,.F.);
#20725=ADVANCED_FACE('',(#2605),#19758,.F.);
#20726=ADVANCED_FACE('',(#2606),#19759,.F.);
#20727=ADVANCED_FACE('',(#2607),#19760,.F.);
#20728=ADVANCED_FACE('',(#2608),#19761,.F.);
#20729=ADVANCED_FACE('',(#2609),#19762,.F.);
#20730=ADVANCED_FACE('',(#2610),#19763,.F.);
#20731=ADVANCED_FACE('',(#2611),#19764,.F.);
#20732=ADVANCED_FACE('',(#2612),#19765,.F.);
#20733=ADVANCED_FACE('',(#2613),#19766,.F.);
#20734=ADVANCED_FACE('',(#2614),#19767,.F.);
#20735=ADVANCED_FACE('',(#2615),#19768,.F.);
#20736=ADVANCED_FACE('',(#2616),#19769,.F.);
#20737=ADVANCED_FACE('',(#2617),#19770,.F.);
#20738=ADVANCED_FACE('',(#2618),#19771,.F.);
#20739=ADVANCED_FACE('',(#2619),#19772,.F.);
#20740=ADVANCED_FACE('',(#2620),#19773,.F.);
#20741=ADVANCED_FACE('',(#2621),#19774,.F.);
#20742=ADVANCED_FACE('',(#2622),#19775,.F.);
#20743=ADVANCED_FACE('',(#2623),#19776,.F.);
#20744=ADVANCED_FACE('',(#2624),#19777,.F.);
#20745=ADVANCED_FACE('',(#2625),#19778,.F.);
#20746=ADVANCED_FACE('',(#2626),#19779,.F.);
#20747=ADVANCED_FACE('',(#2627),#19780,.F.);
#20748=ADVANCED_FACE('',(#2628),#334,.F.);
#20749=ADVANCED_FACE('',(#2629),#335,.F.);
#20750=ADVANCED_FACE('',(#2630,#2304,#2305,#2306,#2307),#2399,.T.);
#20751=ADVANCED_FACE('',(#2631),#19781,.F.);
#20752=ADVANCED_FACE('',(#2632),#336,.F.);
#20753=ADVANCED_FACE('',(#2633),#337,.F.);
#20754=ADVANCED_FACE('',(#2634),#19782,.F.);
#20755=ADVANCED_FACE('',(#2635),#338,.F.);
#20756=ADVANCED_FACE('',(#2636),#339,.F.);
#20757=ADVANCED_FACE('',(#2637),#19783,.F.);
#20758=ADVANCED_FACE('',(#2638),#340,.F.);
#20759=ADVANCED_FACE('',(#2639),#341,.F.);
#20760=ADVANCED_FACE('',(#2640),#19784,.F.);
#20761=ADVANCED_FACE('',(#2641),#19785,.F.);
#20762=ADVANCED_FACE('',(#2642),#19786,.F.);
#20763=ADVANCED_FACE('',(#2643),#19787,.F.);
#20764=ADVANCED_FACE('',(#2644),#2400,.T.);
#20765=ADVANCED_FACE('',(#2645),#2401,.T.);
#20766=ADVANCED_FACE('',(#2646),#2402,.T.);
#20767=ADVANCED_FACE('',(#2647),#2403,.T.);
#20768=ADVANCED_FACE('',(#2648,#2308,#2309,#2310,#2311),#2404,.F.);
#21813=CLOSED_SHELL('',(#20683,#20684,#20685,#20686,#20687,#20688,#20689,
#20690,#20691,#20692,#20693,#20694,#20695,#20696,#20697,#20698,#20699,#20700,
#20701,#20702,#20703,#20704,#20705,#20706,#20707,#20708,#20709,#20710,#20711,
#20712,#20713,#20714,#20715,#20716,#20717,#20718,#20719,#20720,#20721,#20722,
#20723,#20724,#20725,#20726,#20727,#20728,#20729,#20730,#20731,#20732,#20733,
#20734,#20735,#20736,#20737,#20738,#20739,#20740,#20741,#20742,#20743,#20744,
#20745,#20746,#20747,#20748,#20749,#20750,#20751,#20752,#20753,#20754,#20755,
#20756,#20757,#20758,#20759,#20760,#20761,#20762,#20763,#20764,#20765,#20766,
#20767,#20768));
#22082=AXIS2_PLACEMENT_3D('',#27780,#23640,#23641);
#22083=AXIS2_PLACEMENT_3D('',#27781,#23642,#23643);
#22084=AXIS2_PLACEMENT_3D('',#27791,#23645,#23646);
#22085=AXIS2_PLACEMENT_3D('',#27802,#23647,#23648);
#22086=AXIS2_PLACEMENT_3D('',#27853,#23650,#23651);
#22087=AXIS2_PLACEMENT_3D('',#27904,#23653,#23654);
#22088=AXIS2_PLACEMENT_3D('',#27952,#23656,#23657);
#22089=AXIS2_PLACEMENT_3D('',#28003,#23659,#23660);
#22090=AXIS2_PLACEMENT_3D('',#28054,#23662,#23663);
#22091=AXIS2_PLACEMENT_3D('',#28102,#23665,#23666);
#22092=AXIS2_PLACEMENT_3D('',#28121,#23668,#23669);
#22093=AXIS2_PLACEMENT_3D('',#28141,#23670,#23671);
#22094=AXIS2_PLACEMENT_3D('',#28151,#23673,#23674);
#22095=AXIS2_PLACEMENT_3D('',#28162,#23675,#23676);
#22096=AXIS2_PLACEMENT_3D('',#28213,#23678,#23679);
#22097=AXIS2_PLACEMENT_3D('',#28264,#23681,#23682);
#22098=AXIS2_PLACEMENT_3D('',#28312,#23684,#23685);
#22099=AXIS2_PLACEMENT_3D('',#28363,#23687,#23688);
#22100=AXIS2_PLACEMENT_3D('',#28414,#23690,#23691);
#22101=AXIS2_PLACEMENT_3D('',#28462,#23693,#23694);
#22102=AXIS2_PLACEMENT_3D('',#28481,#23696,#23697);
#22103=AXIS2_PLACEMENT_3D('',#28501,#23698,#23699);
#22104=AXIS2_PLACEMENT_3D('',#28511,#23701,#23702);
#22105=AXIS2_PLACEMENT_3D('',#28522,#23703,#23704);
#22106=AXIS2_PLACEMENT_3D('',#28573,#23706,#23707);
#22107=AXIS2_PLACEMENT_3D('',#28624,#23709,#23710);
#22108=AXIS2_PLACEMENT_3D('',#28672,#23712,#23713);
#22109=AXIS2_PLACEMENT_3D('',#28723,#23715,#23716);
#22110=AXIS2_PLACEMENT_3D('',#28774,#23718,#23719);
#22111=AXIS2_PLACEMENT_3D('',#28822,#23721,#23722);
#22112=AXIS2_PLACEMENT_3D('',#28841,#23724,#23725);
#22113=AXIS2_PLACEMENT_3D('',#28861,#23726,#23727);
#22114=AXIS2_PLACEMENT_3D('',#28871,#23729,#23730);
#22115=AXIS2_PLACEMENT_3D('',#28882,#23731,#23732);
#22116=AXIS2_PLACEMENT_3D('',#28933,#23734,#23735);
#22117=AXIS2_PLACEMENT_3D('',#28984,#23737,#23738);
#22118=AXIS2_PLACEMENT_3D('',#29032,#23740,#23741);
#22119=AXIS2_PLACEMENT_3D('',#29083,#23743,#23744);
#22120=AXIS2_PLACEMENT_3D('',#29134,#23746,#23747);
#22121=AXIS2_PLACEMENT_3D('',#29182,#23749,#23750);
#22122=AXIS2_PLACEMENT_3D('',#29201,#23752,#23753);
#22123=AXIS2_PLACEMENT_3D('',#29221,#23754,#23755);
#22124=AXIS2_PLACEMENT_3D('',#29235,#23757,#23758);
#22125=AXIS2_PLACEMENT_3D('',#29245,#23759,#23760);
#22126=AXIS2_PLACEMENT_3D('',#29269,#23762,#23763);
#22127=AXIS2_PLACEMENT_3D('',#29294,#23765,#23766);
#22128=AXIS2_PLACEMENT_3D('',#29319,#23768,#23769);
#22129=AXIS2_PLACEMENT_3D('',#29343,#23771,#23772);
#22130=AXIS2_PLACEMENT_3D('',#29368,#23774,#23775);
#22131=AXIS2_PLACEMENT_3D('',#29393,#23777,#23778);
#22132=AXIS2_PLACEMENT_3D('',#29404,#23780,#23781);
#22133=AXIS2_PLACEMENT_3D('',#29410,#23782,#23783);
#22134=AXIS2_PLACEMENT_3D('',#29424,#23785,#23786);
#22135=AXIS2_PLACEMENT_3D('',#29434,#23787,#23788);
#22136=AXIS2_PLACEMENT_3D('',#29458,#23790,#23791);
#22137=AXIS2_PLACEMENT_3D('',#29483,#23793,#23794);
#22138=AXIS2_PLACEMENT_3D('',#29508,#23796,#23797);
#22139=AXIS2_PLACEMENT_3D('',#29532,#23799,#23800);
#22140=AXIS2_PLACEMENT_3D('',#29557,#23802,#23803);
#22141=AXIS2_PLACEMENT_3D('',#29582,#23805,#23806);
#22142=AXIS2_PLACEMENT_3D('',#29593,#23808,#23809);
#22143=AXIS2_PLACEMENT_3D('',#29599,#23810,#23811);
#22144=AXIS2_PLACEMENT_3D('',#29613,#23813,#23814);
#22145=AXIS2_PLACEMENT_3D('',#29623,#23815,#23816);
#22146=AXIS2_PLACEMENT_3D('',#29647,#23818,#23819);
#22147=AXIS2_PLACEMENT_3D('',#29672,#23821,#23822);
#22148=AXIS2_PLACEMENT_3D('',#29697,#23824,#23825);
#22149=AXIS2_PLACEMENT_3D('',#29721,#23827,#23828);
#22150=AXIS2_PLACEMENT_3D('',#29746,#23830,#23831);
#22151=AXIS2_PLACEMENT_3D('',#29771,#23833,#23834);
#22152=AXIS2_PLACEMENT_3D('',#29782,#23836,#23837);
#22153=AXIS2_PLACEMENT_3D('',#29788,#23838,#23839);
#22154=AXIS2_PLACEMENT_3D('',#29802,#23841,#23842);
#22155=AXIS2_PLACEMENT_3D('',#29812,#23843,#23844);
#22156=AXIS2_PLACEMENT_3D('',#29836,#23846,#23847);
#22157=AXIS2_PLACEMENT_3D('',#29861,#23849,#23850);
#22158=AXIS2_PLACEMENT_3D('',#29886,#23852,#23853);
#22159=AXIS2_PLACEMENT_3D('',#29910,#23855,#23856);
#22160=AXIS2_PLACEMENT_3D('',#29935,#23858,#23859);
#22161=AXIS2_PLACEMENT_3D('',#29960,#23861,#23862);
#22162=AXIS2_PLACEMENT_3D('',#29971,#23864,#23865);
#22163=AXIS2_PLACEMENT_3D('',#29977,#23866,#23867);
#22164=AXIS2_PLACEMENT_3D('',#30879,#23868,#23869);
#22165=AXIS2_PLACEMENT_3D('',#31461,#23874,#23875);
#22166=AXIS2_PLACEMENT_3D('',#32172,#23876,#23877);
#22167=AXIS2_PLACEMENT_3D('',#32883,#23878,#23879);
#22168=AXIS2_PLACEMENT_3D('',#33594,#23880,#23881);
#22169=AXIS2_PLACEMENT_3D('',#33595,#23882,#23883);
#22170=AXIS2_PLACEMENT_3D('',#33596,#23884,#23885);
#22171=AXIS2_PLACEMENT_3D('',#33597,#23886,#23887);
#22172=AXIS2_PLACEMENT_3D('',#33598,#23888,#23889);
#22173=AXIS2_PLACEMENT_3D('',#33604,#23893,#23894);
#22174=AXIS2_PLACEMENT_3D('',#33608,#23897,#23898);
#22175=AXIS2_PLACEMENT_3D('',#33612,#23901,#23902);
#22176=AXIS2_PLACEMENT_3D('',#33614,#23904,#23905);
#23640=DIRECTION('axis',(0.,0.,1.));
#23641=DIRECTION('refdir',(1.,0.,0.));
#23642=DIRECTION('center_axis',(0.,0.,-1.));
#23643=DIRECTION('ref_axis',(-0.34687556303371,0.9379111598494,0.));
#23644=DIRECTION('',(0.,0.,-1.));
#23645=DIRECTION('center_axis',(0.,0.,-1.));
#23646=DIRECTION('ref_axis',(1.,0.,0.));
#23647=DIRECTION('center_axis',(0.,0.,-1.));
#23648=DIRECTION('ref_axis',(1.,0.,0.));
#23649=DIRECTION('',(0.,0.,-1.));
#23650=DIRECTION('center_axis',(0.,0.,-1.));
#23651=DIRECTION('ref_axis',(1.,0.,0.));
#23652=DIRECTION('',(0.,0.,-1.));
#23653=DIRECTION('center_axis',(0.,0.,-1.));
#23654=DIRECTION('ref_axis',(1.,0.,0.));
#23655=DIRECTION('',(0.,0.,-1.));
#23656=DIRECTION('center_axis',(0.,0.,-1.));
#23657=DIRECTION('ref_axis',(1.,0.,0.));
#23658=DIRECTION('',(0.,0.,-1.));
#23659=DIRECTION('center_axis',(0.,0.,-1.));
#23660=DIRECTION('ref_axis',(1.,0.,0.));
#23661=DIRECTION('',(0.,0.,-1.));
#23662=DIRECTION('center_axis',(0.,0.,-1.));
#23663=DIRECTION('ref_axis',(1.,0.,0.));
#23664=DIRECTION('',(0.,0.,-1.));
#23665=DIRECTION('center_axis',(0.,0.,-1.));
#23666=DIRECTION('ref_axis',(0.938001830644068,-0.346630301197656,0.));
#23667=DIRECTION('',(0.,0.,-1.));
#23668=DIRECTION('center_axis',(0.,0.,-1.));
#23669=DIRECTION('ref_axis',(1.,0.,0.));
#23670=DIRECTION('center_axis',(0.,0.,-1.));
#23671=DIRECTION('ref_axis',(-0.346875820911814,0.937911064476134,0.));
#23672=DIRECTION('',(0.,0.,-1.));
#23673=DIRECTION('center_axis',(0.,0.,-1.));
#23674=DIRECTION('ref_axis',(1.,0.,0.));
#23675=DIRECTION('center_axis',(0.,0.,-1.));
#23676=DIRECTION('ref_axis',(1.,0.,0.));
#23677=DIRECTION('',(0.,0.,-1.));
#23678=DIRECTION('center_axis',(0.,0.,-1.));
#23679=DIRECTION('ref_axis',(1.,0.,0.));
#23680=DIRECTION('',(0.,0.,-1.));
#23681=DIRECTION('center_axis',(0.,0.,-1.));
#23682=DIRECTION('ref_axis',(1.,0.,0.));
#23683=DIRECTION('',(0.,0.,-1.));
#23684=DIRECTION('center_axis',(0.,0.,-1.));
#23685=DIRECTION('ref_axis',(1.,0.,0.));
#23686=DIRECTION('',(0.,0.,-1.));
#23687=DIRECTION('center_axis',(0.,0.,-1.));
#23688=DIRECTION('ref_axis',(1.,0.,0.));
#23689=DIRECTION('',(0.,0.,-1.));
#23690=DIRECTION('center_axis',(0.,0.,-1.));
#23691=DIRECTION('ref_axis',(1.,0.,0.));
#23692=DIRECTION('',(0.,0.,-1.));
#23693=DIRECTION('center_axis',(0.,0.,-1.));
#23694=DIRECTION('ref_axis',(0.938001844837498,-0.346630262789403,0.));
#23695=DIRECTION('',(0.,0.,-1.));
#23696=DIRECTION('center_axis',(0.,0.,-1.));
#23697=DIRECTION('ref_axis',(1.,0.,0.));
#23698=DIRECTION('center_axis',(0.,0.,-1.));
#23699=DIRECTION('ref_axis',(-0.346875921807931,0.937911027160838,0.));
#23700=DIRECTION('',(0.,0.,-1.));
#23701=DIRECTION('center_axis',(0.,0.,-1.));
#23702=DIRECTION('ref_axis',(1.,0.,0.));
#23703=DIRECTION('center_axis',(0.,0.,-1.));
#23704=DIRECTION('ref_axis',(1.,0.,0.));
#23705=DIRECTION('',(0.,0.,-1.));
#23706=DIRECTION('center_axis',(0.,0.,-1.));
#23707=DIRECTION('ref_axis',(1.,0.,0.));
#23708=DIRECTION('',(0.,0.,-1.));
#23709=DIRECTION('center_axis',(0.,0.,-1.));
#23710=DIRECTION('ref_axis',(1.,0.,0.));
#23711=DIRECTION('',(0.,0.,-1.));
#23712=DIRECTION('center_axis',(0.,0.,-1.));
#23713=DIRECTION('ref_axis',(1.,0.,0.));
#23714=DIRECTION('',(0.,0.,-1.));
#23715=DIRECTION('center_axis',(0.,0.,-1.));
#23716=DIRECTION('ref_axis',(1.,0.,0.));
#23717=DIRECTION('',(0.,0.,-1.));
#23718=DIRECTION('center_axis',(0.,0.,-1.));
#23719=DIRECTION('ref_axis',(1.,0.,0.));
#23720=DIRECTION('',(0.,0.,-1.));
#23721=DIRECTION('center_axis',(0.,0.,-1.));
#23722=DIRECTION('ref_axis',(0.93800185687022,-0.346630230228148,0.));
#23723=DIRECTION('',(0.,0.,-1.));
#23724=DIRECTION('center_axis',(0.,0.,-1.));
#23725=DIRECTION('ref_axis',(1.,0.,0.));
#23726=DIRECTION('center_axis',(0.,0.,-1.));
#23727=DIRECTION('ref_axis',(-0.346875444642522,0.937911203634999,0.));
#23728=DIRECTION('',(0.,0.,-1.));
#23729=DIRECTION('center_axis',(0.,0.,-1.));
#23730=DIRECTION('ref_axis',(1.,0.,0.));
#23731=DIRECTION('center_axis',(0.,0.,-1.));
#23732=DIRECTION('ref_axis',(1.,0.,0.));
#23733=DIRECTION('',(0.,0.,-1.));
#23734=DIRECTION('center_axis',(0.,0.,-1.));
#23735=DIRECTION('ref_axis',(1.,0.,0.));
#23736=DIRECTION('',(0.,0.,-1.));
#23737=DIRECTION('center_axis',(0.,0.,-1.));
#23738=DIRECTION('ref_axis',(1.,0.,0.));
#23739=DIRECTION('',(0.,0.,-1.));
#23740=DIRECTION('center_axis',(0.,0.,-1.));
#23741=DIRECTION('ref_axis',(1.,0.,0.));
#23742=DIRECTION('',(0.,0.,-1.));
#23743=DIRECTION('center_axis',(0.,0.,-1.));
#23744=DIRECTION('ref_axis',(1.,0.,0.));
#23745=DIRECTION('',(0.,0.,-1.));
#23746=DIRECTION('center_axis',(0.,0.,-1.));
#23747=DIRECTION('ref_axis',(1.,0.,0.));
#23748=DIRECTION('',(0.,0.,-1.));
#23749=DIRECTION('center_axis',(0.,0.,-1.));
#23750=DIRECTION('ref_axis',(0.938001817986921,-0.346630335448631,0.));
#23751=DIRECTION('',(0.,0.,-1.));
#23752=DIRECTION('center_axis',(0.,0.,-1.));
#23753=DIRECTION('ref_axis',(1.,0.,0.));
#23754=DIRECTION('center_axis',(0.,0.,-1.));
#23755=DIRECTION('ref_axis',(0.793238775227928,0.608910704023913,0.));
#23756=DIRECTION('',(1.22464679914735E-16,-2.81870473344804E-30,-1.));
#23757=DIRECTION('center_axis',(0.,0.,1.));
#23758=DIRECTION('ref_axis',(1.,-2.28940061540476E-14,0.));
#23759=DIRECTION('center_axis',(0.,0.,-1.));
#23760=DIRECTION('ref_axis',(1.,-2.28940061540476E-14,0.));
#23761=DIRECTION('',(1.22464679914735E-16,-2.81870473344804E-30,-1.));
#23762=DIRECTION('center_axis',(0.,0.,-1.));
#23763=DIRECTION('ref_axis',(1.,-2.28940061540476E-14,0.));
#23764=DIRECTION('',(1.22464679914735E-16,-2.81870473344804E-30,-1.));
#23765=DIRECTION('center_axis',(0.,0.,-1.));
#23766=DIRECTION('ref_axis',(1.,-2.28940061540476E-14,0.));
#23767=DIRECTION('',(1.22464679914735E-16,-2.81870473344804E-30,-1.));
#23768=DIRECTION('center_axis',(0.,0.,-1.));
#23769=DIRECTION('ref_axis',(1.,-2.28940061540476E-14,0.));
#23770=DIRECTION('',(1.22464679914735E-16,-2.81870473344804E-30,-1.));
#23771=DIRECTION('center_axis',(0.,0.,-1.));
#23772=DIRECTION('ref_axis',(1.,-2.28940061540476E-14,0.));
#23773=DIRECTION('',(1.22464679914735E-16,-2.81870473344804E-30,-1.));
#23774=DIRECTION('center_axis',(0.,0.,-1.));
#23775=DIRECTION('ref_axis',(1.,-2.28940061540476E-14,0.));
#23776=DIRECTION('',(1.22464679914735E-16,-2.81870473344804E-30,-1.));
#23777=DIRECTION('center_axis',(0.,0.,-1.));
#23778=DIRECTION('ref_axis',(-0.609093973761813,-0.793098058960582,0.));
#23779=DIRECTION('',(1.22464679914735E-16,-2.81870473344804E-30,-1.));
#23780=DIRECTION('center_axis',(0.,0.,-1.));
#23781=DIRECTION('ref_axis',(1.,-2.28940061540476E-14,0.));
#23782=DIRECTION('center_axis',(0.,0.,-1.));
#23783=DIRECTION('ref_axis',(0.79323871288191,0.608910785243167,0.));
#23784=DIRECTION('',(1.22464679914735E-16,-2.55168500624601E-30,-1.));
#23785=DIRECTION('center_axis',(0.,0.,1.));
#23786=DIRECTION('ref_axis',(1.,-2.0713624615567E-14,0.));
#23787=DIRECTION('center_axis',(0.,0.,-1.));
#23788=DIRECTION('ref_axis',(1.,-2.0713624615567E-14,0.));
#23789=DIRECTION('',(1.22464679914735E-16,-2.55168500624601E-30,-1.));
#23790=DIRECTION('center_axis',(0.,0.,-1.));
#23791=DIRECTION('ref_axis',(1.,-2.0713624615567E-14,0.));
#23792=DIRECTION('',(1.22464679914735E-16,-2.55168500624601E-30,-1.));
#23793=DIRECTION('center_axis',(0.,0.,-1.));
#23794=DIRECTION('ref_axis',(1.,-2.0713624615567E-14,0.));
#23795=DIRECTION('',(1.22464679914735E-16,-2.55168500624601E-30,-1.));
#23796=DIRECTION('center_axis',(0.,0.,-1.));
#23797=DIRECTION('ref_axis',(1.,-2.0713624615567E-14,0.));
#23798=DIRECTION('',(1.22464679914735E-16,-2.55168500624601E-30,-1.));
#23799=DIRECTION('center_axis',(0.,0.,-1.));
#23800=DIRECTION('ref_axis',(1.,-2.0713624615567E-14,0.));
#23801=DIRECTION('',(1.22464679914735E-16,-2.55168500624601E-30,-1.));
#23802=DIRECTION('center_axis',(0.,0.,-1.));
#23803=DIRECTION('ref_axis',(1.,-2.0713624615567E-14,0.));
#23804=DIRECTION('',(1.22464679914735E-16,-2.55168500624601E-30,-1.));
#23805=DIRECTION('center_axis',(0.,0.,-1.));
#23806=DIRECTION('ref_axis',(-0.609093936537935,-0.793098087548269,0.));
#23807=DIRECTION('',(1.22464679914735E-16,-2.55168500624601E-30,-1.));
#23808=DIRECTION('center_axis',(0.,0.,-1.));
#23809=DIRECTION('ref_axis',(1.,-2.0713624615567E-14,0.));
#23810=DIRECTION('center_axis',(0.,0.,-1.));
#23811=DIRECTION('ref_axis',(0.793238788726965,0.608910686438477,0.));
#23812=DIRECTION('',(1.22464679914735E-16,-2.55168500624601E-30,-1.));
#23813=DIRECTION('center_axis',(0.,0.,1.));
#23814=DIRECTION('ref_axis',(1.,-2.0713624615567E-14,0.));
#23815=DIRECTION('center_axis',(0.,0.,-1.));
#23816=DIRECTION('ref_axis',(1.,-2.0713624615567E-14,0.));
#23817=DIRECTION('',(1.22464679914735E-16,-2.55168500624601E-30,-1.));
#23818=DIRECTION('center_axis',(0.,0.,-1.));
#23819=DIRECTION('ref_axis',(1.,-2.0713624615567E-14,0.));
#23820=DIRECTION('',(1.22464679914735E-16,-2.55168500624601E-30,-1.));
#23821=DIRECTION('center_axis',(0.,0.,-1.));
#23822=DIRECTION('ref_axis',(1.,-2.0713624615567E-14,0.));
#23823=DIRECTION('',(1.22464679914735E-16,-2.55168500624601E-30,-1.));
#23824=DIRECTION('center_axis',(0.,0.,-1.));
#23825=DIRECTION('ref_axis',(1.,-2.0713624615567E-14,0.));
#23826=DIRECTION('',(1.22464679914735E-16,-2.55168500624601E-30,-1.));
#23827=DIRECTION('center_axis',(0.,0.,-1.));
#23828=DIRECTION('ref_axis',(1.,-2.0713624615567E-14,0.));
#23829=DIRECTION('',(1.22464679914735E-16,-2.55168500624601E-30,-1.));
#23830=DIRECTION('center_axis',(0.,0.,-1.));
#23831=DIRECTION('ref_axis',(1.,-2.0713624615567E-14,0.));
#23832=DIRECTION('',(1.22464679914735E-16,-2.55168500624601E-30,-1.));
#23833=DIRECTION('center_axis',(0.,0.,-1.));
#23834=DIRECTION('ref_axis',(-0.609093953553475,-0.79309807448045,0.));
#23835=DIRECTION('',(1.22464679914735E-16,-2.55168500624601E-30,-1.));
#23836=DIRECTION('center_axis',(0.,0.,-1.));
#23837=DIRECTION('ref_axis',(1.,-2.0713624615567E-14,0.));
#23838=DIRECTION('center_axis',(0.,0.,-1.));
#23839=DIRECTION('ref_axis',(0.793238729919907,0.608910763047471,0.));
#23840=DIRECTION('',(1.22464679914735E-16,-2.551685006246E-30,-1.));
#23841=DIRECTION('center_axis',(0.,0.,1.));
#23842=DIRECTION('ref_axis',(1.,-2.07136246155669E-14,0.));
#23843=DIRECTION('center_axis',(0.,0.,-1.));
#23844=DIRECTION('ref_axis',(1.,-2.07136246155669E-14,0.));
#23845=DIRECTION('',(1.22464679914735E-16,-2.551685006246E-30,-1.));
#23846=DIRECTION('center_axis',(0.,0.,-1.));
#23847=DIRECTION('ref_axis',(1.,-2.07136246155669E-14,0.));
#23848=DIRECTION('',(1.22464679914735E-16,-2.551685006246E-30,-1.));
#23849=DIRECTION('center_axis',(0.,0.,-1.));
#23850=DIRECTION('ref_axis',(1.,-2.07136246155669E-14,0.));
#23851=DIRECTION('',(1.22464679914735E-16,-2.551685006246E-30,-1.));
#23852=DIRECTION('center_axis',(0.,0.,-1.));
#23853=DIRECTION('ref_axis',(1.,-2.07136246155669E-14,0.));
#23854=DIRECTION('',(1.22464679914735E-16,-2.551685006246E-30,-1.));
#23855=DIRECTION('center_axis',(0.,0.,-1.));
#23856=DIRECTION('ref_axis',(1.,-2.07136246155669E-14,0.));
#23857=DIRECTION('',(1.22464679914735E-16,-2.551685006246E-30,-1.));
#23858=DIRECTION('center_axis',(0.,0.,-1.));
#23859=DIRECTION('ref_axis',(1.,-2.07136246155669E-14,0.));
#23860=DIRECTION('',(1.22464679914735E-16,-2.551685006246E-30,-1.));
#23861=DIRECTION('center_axis',(0.,0.,-1.));
#23862=DIRECTION('ref_axis',(-0.609093922666122,-0.793098098201727,0.));
#23863=DIRECTION('',(1.22464679914735E-16,-2.551685006246E-30,-1.));
#23864=DIRECTION('center_axis',(0.,0.,-1.));
#23865=DIRECTION('ref_axis',(1.,-2.07136246155669E-14,0.));
#23866=DIRECTION('center_axis',(0.,0.,-1.));
#23867=DIRECTION('ref_axis',(1.,-2.07136246155669E-14,0.));
#23868=DIRECTION('center_axis',(0.,0.,1.));
#23869=DIRECTION('ref_axis',(1.,0.,0.));
#23870=DIRECTION('',(0.,-1.,0.));
#23871=DIRECTION('',(1.,0.,0.));
#23872=DIRECTION('',(0.,1.,0.));
#23873=DIRECTION('',(-1.,0.,0.));
#23874=DIRECTION('center_axis',(0.,0.,-1.));
#23875=DIRECTION('ref_axis',(1.,-2.0713624615567E-14,0.));
#23876=DIRECTION('center_axis',(0.,0.,-1.));
#23877=DIRECTION('ref_axis',(1.,-2.0713624615567E-14,0.));
#23878=DIRECTION('center_axis',(0.,0.,-1.));
#23879=DIRECTION('ref_axis',(1.,-2.28940061540476E-14,0.));
#23880=DIRECTION('center_axis',(0.,0.,-1.));
#23881=DIRECTION('ref_axis',(1.,0.,0.));
#23882=DIRECTION('center_axis',(0.,0.,-1.));
#23883=DIRECTION('ref_axis',(1.,0.,0.));
#23884=DIRECTION('center_axis',(0.,0.,-1.));
#23885=DIRECTION('ref_axis',(1.,0.,0.));
#23886=DIRECTION('center_axis',(0.,0.,-1.));
#23887=DIRECTION('ref_axis',(1.,0.,0.));
#23888=DIRECTION('center_axis',(0.,1.,0.));
#23889=DIRECTION('ref_axis',(-1.,0.,0.));
#23890=DIRECTION('',(-1.,0.,0.));
#23891=DIRECTION('',(0.,0.,1.));
#23892=DIRECTION('',(0.,0.,1.));
#23893=DIRECTION('center_axis',(1.,0.,0.));
#23894=DIRECTION('ref_axis',(0.,1.,0.));
#23895=DIRECTION('',(0.,1.,0.));
#23896=DIRECTION('',(0.,0.,1.));
#23897=DIRECTION('center_axis',(0.,-1.,0.));
#23898=DIRECTION('ref_axis',(1.,0.,0.));
#23899=DIRECTION('',(1.,0.,0.));
#23900=DIRECTION('',(0.,0.,1.));
#23901=DIRECTION('center_axis',(-1.,0.,0.));
#23902=DIRECTION('ref_axis',(0.,-1.,0.));
#23903=DIRECTION('',(0.,-1.,0.));
#23904=DIRECTION('center_axis',(0.,0.,1.));
#23905=DIRECTION('ref_axis',(1.,0.,0.));
#27780=CARTESIAN_POINT('',(0.,0.,0.));
#27781=CARTESIAN_POINT('Origin',(35.,35.,4.));
#27782=CARTESIAN_POINT('',(31.4879724201494,34.9998624352662,0.387416697508018));
#27783=CARTESIAN_POINT('',(31.4848003100606,34.9953496614248,0.112583302491981));
#27784=CARTESIAN_POINT('',(31.4825,35.,4.));
#27785=CARTESIAN_POINT('',(32.3264680662286,37.2858331630075,0.));
#27786=CARTESIAN_POINT('Ctrl Pts',(31.4848003100606,34.9953496614248,0.112583302491981));
#27787=CARTESIAN_POINT('Ctrl Pts',(31.491976688325,35.8232723665277,0.0750555349946529));
#27788=CARTESIAN_POINT('Ctrl Pts',(31.7874825103136,36.6554305951821,0.0375277674973252));
#27789=CARTESIAN_POINT('Ctrl Pts',(32.3264680662287,37.2858331630075,-2.22044604925031E-15));
#27790=CARTESIAN_POINT('',(37.6785012740241,37.2890246412443,7.00840805882243E-15));
#27791=CARTESIAN_POINT('Origin',(35.,35.,0.));
#27792=CARTESIAN_POINT('Ctrl Pts',(37.6785244495407,37.2890395253442,4.78783679369599E-15));
#27793=CARTESIAN_POINT('Ctrl Pts',(36.9607517209778,38.1233243316157,0.0499978774624456));
#27794=CARTESIAN_POINT('Ctrl Pts',(35.818670130213,38.598920544762,0.0999957549248864));
#27795=CARTESIAN_POINT('Ctrl Pts',(34.7217021974699,38.5118549254553,0.149993632387327));
#27796=CARTESIAN_POINT('Ctrl Pts',(33.5734927541699,38.4207223013458,0.202327008171411));
#27797=CARTESIAN_POINT('Ctrl Pts',(32.4747101009944,37.7131340510847,0.254660383955495));
#27798=CARTESIAN_POINT('Ctrl Pts',(31.9173289273845,36.7055535968161,0.306993759739579));
#27799=CARTESIAN_POINT('Ctrl Pts',(31.6318117612872,36.1894229315936,0.333801405662392));
#27800=CARTESIAN_POINT('Ctrl Pts',(31.4883570437126,35.5945750322157,0.360609051585205));
#27801=CARTESIAN_POINT('Ctrl Pts',(31.4879724201494,34.9998624352662,0.387416697508018));
#27802=CARTESIAN_POINT('Origin',(35.,35.,4.));
#27803=CARTESIAN_POINT('',(31.4787691259179,34.9978480355345,1.38741669750802));
#27804=CARTESIAN_POINT('',(31.4779837004207,35.0016823853973,1.11258330249198));
#27805=CARTESIAN_POINT('',(31.4825,35.,4.));
#27806=CARTESIAN_POINT('Ctrl Pts',(31.4779837004207,35.0016823853973,1.11258330249198));
#27807=CARTESIAN_POINT('Ctrl Pts',(31.4773936874682,35.1013890235937,1.10805583214991));
#27808=CARTESIAN_POINT('Ctrl Pts',(31.4812693590031,35.201048825548,1.10352836180784));
#27809=CARTESIAN_POINT('Ctrl Pts',(31.4897612702936,35.3003133216161,1.09900089146578));
#27810=CARTESIAN_POINT('Ctrl Pts',(31.5879199220602,36.4477192198909,1.04666751568169));
#27811=CARTESIAN_POINT('Ctrl Pts',(32.3028647460417,37.5423074099748,0.994334139897606));
#27812=CARTESIAN_POINT('Ctrl Pts',(33.3140597553874,38.0934397445863,0.942000764113521));
#27813=CARTESIAN_POINT('Ctrl Pts',(34.3252547647332,38.6445720791978,0.889667388329437));
#27814=CARTESIAN_POINT('Ctrl Pts',(35.632699959443,38.652248558337,0.837334012545353));
#27815=CARTESIAN_POINT('Ctrl Pts',(36.6501699298679,38.1127741860318,0.785000636761269));
#27816=CARTESIAN_POINT('Ctrl Pts',(37.6676399002927,37.5732998137267,0.732667260977184));
#27817=CARTESIAN_POINT('Ctrl Pts',(38.3951346464326,36.4866745899774,0.680333885193099));
#27818=CARTESIAN_POINT('Ctrl Pts',(38.5065308772508,35.3406022936711,0.628000509409014));
#27819=CARTESIAN_POINT('Ctrl Pts',(38.617927108069,34.1945299973649,0.57566713362493));
#27820=CARTESIAN_POINT('Ctrl Pts',(38.1132248235656,32.9890106285018,0.523333757840846));
#27821=CARTESIAN_POINT('Ctrl Pts',(37.2186051779362,32.2635143561234,0.471000382056762));
#27822=CARTESIAN_POINT('Ctrl Pts',(36.3239855323068,31.538018083745,0.418667006272677));
#27823=CARTESIAN_POINT('Ctrl Pts',(35.0394485255514,31.2925449078513,0.366333630488592));
#27824=CARTESIAN_POINT('Ctrl Pts',(33.9411234140671,31.6392615363868,0.314000254704508));
#27825=CARTESIAN_POINT('Ctrl Pts',(32.8427983025828,31.9859781649222,0.261666878920424));
#27826=CARTESIAN_POINT('Ctrl Pts',(31.9306850863697,32.9248845978868,0.20933350313634));
#27827=CARTESIAN_POINT('Ctrl Pts',(31.6136954419349,34.0300704557469,0.157000127352256));
#27828=CARTESIAN_POINT('Ctrl Pts',(31.5240160655112,34.3427380154138,0.142194519065497));
#27829=CARTESIAN_POINT('Ctrl Pts',(31.481969055963,34.6687142103727,0.127388910778739));
#27830=CARTESIAN_POINT('Ctrl Pts',(31.4848003100606,34.9953496614248,0.112583302491981));
#27831=CARTESIAN_POINT('Ctrl Pts',(31.4879724201494,34.9998624352662,0.387416697508018));
#27832=CARTESIAN_POINT('Ctrl Pts',(31.4876061889182,34.4335884275247,0.41294242736929));
#27833=CARTESIAN_POINT('Ctrl Pts',(31.6169542536305,33.8674370915364,0.438468157230561));
#27834=CARTESIAN_POINT('Ctrl Pts',(31.8768865080858,33.3694813094911,0.463993887091832));
#27835=CARTESIAN_POINT('Ctrl Pts',(32.4098049564414,32.3485621347107,0.516327262875917));
#27836=CARTESIAN_POINT('Ctrl Pts',(33.4916215471969,31.6142964434261,0.568660638660002));
#27837=CARTESIAN_POINT('Ctrl Pts',(34.6371338346999,31.4957027110504,0.620994014444087));
#27838=CARTESIAN_POINT('Ctrl Pts',(35.7826461222029,31.3771089786747,0.673327390228171));
#27839=CARTESIAN_POINT('Ctrl Pts',(36.9918541064533,31.8741872052079,0.725660766012256));
#27840=CARTESIAN_POINT('Ctrl Pts',(37.7226853676378,32.7641657941898,0.77799414179634));
#27841=CARTESIAN_POINT('Ctrl Pts',(38.4535166288223,33.6541443831717,0.830327517580425));
#27842=CARTESIAN_POINT('Ctrl Pts',(38.7059711669407,34.9370233346023,0.882660893364508));
#27843=CARTESIAN_POINT('Ctrl Pts',(38.3668191926393,36.0375701678912,0.934994269148593));
#27844=CARTESIAN_POINT('Ctrl Pts',(38.0276672183379,37.13811700118,0.987327644932677));
#27845=CARTESIAN_POINT('Ctrl Pts',(37.0969087316166,38.0563317163271,1.03966102071676));
#27846=CARTESIAN_POINT('Ctrl Pts',(35.9918739069821,38.3805519391724,1.09199439650085));
#27847=CARTESIAN_POINT('Ctrl Pts',(34.8868390823475,38.7047721620176,1.14432777228493));
#27848=CARTESIAN_POINT('Ctrl Pts',(33.6075279197997,38.4349978925611,1.19666114806902));
#27849=CARTESIAN_POINT('Ctrl Pts',(32.727515719297,37.6921720072953,1.2489945238531));
#27850=CARTESIAN_POINT('Ctrl Pts',(31.9516360834601,37.0372453176186,1.29513524840474));
#27851=CARTESIAN_POINT('Ctrl Pts',(31.4861477200874,36.0145964274628,1.34127597295638));
#27852=CARTESIAN_POINT('Ctrl Pts',(31.4787691259179,34.9978480355345,1.38741669750802));
#27853=CARTESIAN_POINT('Origin',(35.,35.,4.));
#27854=CARTESIAN_POINT('',(31.4830373600778,35.0030273041289,2.38741669750802));
#27855=CARTESIAN_POINT('',(31.4877387493273,35.0007919718047,2.11258330249198));
#27856=CARTESIAN_POINT('',(31.4825,35.,4.));
#27857=CARTESIAN_POINT('Ctrl Pts',(31.4877387493273,35.0007919718047,2.11258330249198));
#27858=CARTESIAN_POINT('Ctrl Pts',(31.4866495532798,35.5300199293211,2.08872275352109));
#27859=CARTESIAN_POINT('Ctrl Pts',(31.5990326814287,36.0588086783673,2.06486220455019));
#27860=CARTESIAN_POINT('Ctrl Pts',(31.8273024854561,36.5316518026084,2.0410016555793));
#27861=CARTESIAN_POINT('Ctrl Pts',(32.3279669692824,37.5687392953569,1.98866827979521));
#27862=CARTESIAN_POINT('Ctrl Pts',(33.3861125458452,38.3366963827873,1.93633490401113));
#27863=CARTESIAN_POINT('Ctrl Pts',(34.5273147643209,38.4912077048459,1.88400152822704));
#27864=CARTESIAN_POINT('Ctrl Pts',(35.6685169827965,38.6457190269045,1.83166815244296));
#27865=CARTESIAN_POINT('Ctrl Pts',(36.8927758431849,38.1867845835912,1.77933477665887));
#27866=CARTESIAN_POINT('Ctrl Pts',(37.6511886219643,37.3201660399649,1.72700140087479));
#27867=CARTESIAN_POINT('Ctrl Pts',(38.4096014007438,36.4535474963386,1.6746680250907));
#27868=CARTESIAN_POINT('Ctrl Pts',(38.7021680979142,35.1792448523993,1.62233464930662));
#27869=CARTESIAN_POINT('Ctrl Pts',(38.3977158188189,34.0686054522412,1.57000127352253));
#27870=CARTESIAN_POINT('Ctrl Pts',(38.0932635397237,32.9579660520831,1.51766789773845));
#27871=CARTESIAN_POINT('Ctrl Pts',(37.1917922843629,32.0109898957062,1.46533452195437));
#27872=CARTESIAN_POINT('Ctrl Pts',(36.0974794284194,31.6522428960312,1.41300114617028));
#27873=CARTESIAN_POINT('Ctrl Pts',(35.0031665724759,31.2934958963563,1.3606677703862));
#27874=CARTESIAN_POINT('Ctrl Pts',(33.7160121159498,31.5229780533832,1.30833439460211));
#27875=CARTESIAN_POINT('Ctrl Pts',(32.8131211274626,32.2378309351295,1.25600101881803));
#27876=CARTESIAN_POINT('Ctrl Pts',(31.9883411362357,32.8908403914793,1.20819511337601));
#27877=CARTESIAN_POINT('Ctrl Pts',(31.4842136922894,33.9488723706596,1.160389207934));
#27878=CARTESIAN_POINT('Ctrl Pts',(31.4779837004207,35.0016823853973,1.11258330249198));
#27879=CARTESIAN_POINT('Ctrl Pts',(31.4787691259179,34.9978480355345,1.38741669750802));
#27880=CARTESIAN_POINT('Ctrl Pts',(31.4777788280689,34.86138792912,1.39360934874046));
#27881=CARTESIAN_POINT('Ctrl Pts',(31.4850404305936,34.725034107982,1.39980199997291));
#27882=CARTESIAN_POINT('Ctrl Pts',(31.5009110513053,34.5896898261078,1.40599465120535));
#27883=CARTESIAN_POINT('Ctrl Pts',(31.6350318222736,33.445911031261,1.45832802698944));
#27884=CARTESIAN_POINT('Ctrl Pts',(32.3839866026675,32.3742309426426,1.51066140277352));
#27885=CARTESIAN_POINT('Ctrl Pts',(33.411975462032,31.855139584126,1.56299477855761));
#27886=CARTESIAN_POINT('Ctrl Pts',(34.4399643213965,31.3360482256093,1.61532815434169));
#27887=CARTESIAN_POINT('Ctrl Pts',(35.7469872597314,31.3695455971944,1.66766153012578));
#27888=CARTESIAN_POINT('Ctrl Pts',(36.7470354950296,31.9406144231743,1.71999490590986));
#27889=CARTESIAN_POINT('Ctrl Pts',(37.7470837303277,32.5116832491543,1.77232828169395));
#27890=CARTESIAN_POINT('Ctrl Pts',(38.4401572625891,33.620323529529,1.82466165747803));
#27891=CARTESIAN_POINT('Ctrl Pts',(38.5155126426898,34.7694703662421,1.87699503326212));
#27892=CARTESIAN_POINT('Ctrl Pts',(38.5908680227905,35.9186172029552,1.9293284090462));
#27893=CARTESIAN_POINT('Ctrl Pts',(38.0485052507305,37.1082705960066,1.98166178483028));
#27894=CARTESIAN_POINT('Ctrl Pts',(37.1315955779125,37.8050440926957,2.03399516061437));
#27895=CARTESIAN_POINT('Ctrl Pts',(36.2146859050945,38.5018175893848,2.08632853639845));
#27896=CARTESIAN_POINT('Ctrl Pts',(34.9232293315183,38.7057111897115,2.13866191218254));
#27897=CARTESIAN_POINT('Ctrl Pts',(33.836256457425,38.3253080449544,2.19099528796662));
#27898=CARTESIAN_POINT('Ctrl Pts',(32.7492835833317,37.9449049001973,2.24332866375071));
#27899=CARTESIAN_POINT('Ctrl Pts',(31.8667944087212,36.9802050103563,2.29566203953479));
#27900=CARTESIAN_POINT('Ctrl Pts',(31.5844572622636,35.8637362853384,2.34799541531888));
#27901=CARTESIAN_POINT('Ctrl Pts',(31.5135650119789,35.583401298313,2.36113584271526));
#27902=CARTESIAN_POINT('Ctrl Pts',(31.4805102901148,35.2934978064005,2.37427627011164));
#27903=CARTESIAN_POINT('Ctrl Pts',(31.4830373600778,35.0030273041289,2.38741669750802));
#27904=CARTESIAN_POINT('Origin',(35.,35.,4.));
#27905=CARTESIAN_POINT('',(31.4866348863052,34.9979909502101,3.38741669750802));
#27906=CARTESIAN_POINT('',(31.48047694743,34.9972296622465,3.11258330249198));
#27907=CARTESIAN_POINT('',(31.4825,35.,4.));
#27908=CARTESIAN_POINT('Ctrl Pts',(31.48047694743,34.9972296622465,3.11258330249198));
#27909=CARTESIAN_POINT('Ctrl Pts',(31.4887007318231,35.9502403897084,3.06938967489226));
#27910=CARTESIAN_POINT('Ctrl Pts',(31.8903810058125,36.9093635615769,3.02619604729254));
#27911=CARTESIAN_POINT('Ctrl Pts',(32.5815433671812,37.5618418521763,2.98300241969282));
#27912=CARTESIAN_POINT('Ctrl Pts',(33.4189553095288,38.352384195351,2.93066904390873));
#27913=CARTESIAN_POINT('Ctrl Pts',(34.6813192114488,38.6927800566904,2.87833566812465));
#27914=CARTESIAN_POINT('Ctrl Pts',(35.8026481651385,38.4304113471867,2.82600229234057));
#27915=CARTESIAN_POINT('Ctrl Pts',(36.9239771188282,38.1680426376829,2.77366891655648));
#27916=CARTESIAN_POINT('Ctrl Pts',(37.9042711242876,37.3029093573359,2.7213355407724));
#27917=CARTESIAN_POINT('Ctrl Pts',(38.3040106560533,36.2228981053939,2.66900216498831));
#27918=CARTESIAN_POINT('Ctrl Pts',(38.703750187819,35.1428868534519,2.61666878920423));
#27919=CARTESIAN_POINT('Ctrl Pts',(38.5229352458909,33.8479976299149,2.56433541342014));
#27920=CARTESIAN_POINT('Ctrl Pts',(37.8426350886114,32.9188003439573,2.51200203763606));
#27921=CARTESIAN_POINT('Ctrl Pts',(37.1623349313319,31.9896030579996,2.45966866185197));
#27922=CARTESIAN_POINT('Ctrl Pts',(35.9825495587008,31.4260977096214,2.40733528606789));
#27923=CARTESIAN_POINT('Ctrl Pts',(34.8322413779487,31.4809343941795,2.3550019102838));
#27924=CARTESIAN_POINT('Ctrl Pts',(33.6819331971966,31.5357710787376,2.30266853449972));
#27925=CARTESIAN_POINT('Ctrl Pts',(32.5611022083236,32.208949796232,2.25033515871564));
#27926=CARTESIAN_POINT('Ctrl Pts',(31.9722784094319,33.1986481040126,2.19800178293155));
#27927=CARTESIAN_POINT('Ctrl Pts',(31.6519192161228,33.7371096133752,2.16952895611836));
#27928=CARTESIAN_POINT('Ctrl Pts',(31.4890384885104,34.3692635020513,2.14105612930517));
#27929=CARTESIAN_POINT('Ctrl Pts',(31.4877387493273,35.0007919718047,2.11258330249198));
#27930=CARTESIAN_POINT('Ctrl Pts',(31.4830373600778,35.0030273041289,2.38741669750802));
#27931=CARTESIAN_POINT('Ctrl Pts',(31.4905746584961,34.1366631395343,2.42660964589572));
#27932=CARTESIAN_POINT('Ctrl Pts',(31.8146491184789,33.2652548262212,2.46580259428343));
#27933=CARTESIAN_POINT('Ctrl Pts',(32.3954080438652,32.6276439552295,2.50499554267113));
#27934=CARTESIAN_POINT('Ctrl Pts',(33.1708810902294,31.7762579103332,2.55732891845521));
#27935=CARTESIAN_POINT('Ctrl Pts',(34.4040123012624,31.3417233807355,2.6096622942393));
#27936=CARTESIAN_POINT('Ctrl Pts',(35.5419214016919,31.5188660285384,2.66199567002338));
#27937=CARTESIAN_POINT('Ctrl Pts',(36.6798305021214,31.6960086763413,2.71432904580747));
#27938=CARTESIAN_POINT('Ctrl Pts',(37.7225174919474,32.4848285015448,2.76666242159155));
#27939=CARTESIAN_POINT('Ctrl Pts',(38.2024886486778,33.5316543411059,2.81899579737563));
#27940=CARTESIAN_POINT('Ctrl Pts',(38.6824598054083,34.5784801806669,2.87132917315972));
#27941=CARTESIAN_POINT('Ctrl Pts',(38.5997151290432,35.8833120345855,2.9236625489438));
#27942=CARTESIAN_POINT('Ctrl Pts',(37.9913535966355,36.8611222874319,2.97599592472789));
#27943=CARTESIAN_POINT('Ctrl Pts',(37.3829920642279,37.8389325402782,3.02832930051197));
#27944=CARTESIAN_POINT('Ctrl Pts',(36.2490136757777,38.4897211920522,3.08066267629606));
#27945=CARTESIAN_POINT('Ctrl Pts',(35.0978430789634,38.5217040264218,3.13299605208014));
#27946=CARTESIAN_POINT('Ctrl Pts',(33.946672482149,38.5536868607913,3.18532942786423));
#27947=CARTESIAN_POINT('Ctrl Pts',(32.7783096769706,37.9668638777563,3.23766280364831));
#27948=CARTESIAN_POINT('Ctrl Pts',(32.1165957326192,37.0243399779266,3.2899961794324));
#27949=CARTESIAN_POINT('Ctrl Pts',(31.7059940575521,36.4394922573,3.3224696854576));
#27950=CARTESIAN_POINT('Ctrl Pts',(31.4904702191063,35.7176870288261,3.35494319148281));
#27951=CARTESIAN_POINT('Ctrl Pts',(31.4866348863052,34.9979909502101,3.38741669750802));
#27952=CARTESIAN_POINT('Origin',(35.,35.,4.));
#27953=CARTESIAN_POINT('',(31.4769533103746,34.9997936499005,4.38741669750802));
#27954=CARTESIAN_POINT('',(31.4811433043907,35.0029051520383,4.11258330249198));
#27955=CARTESIAN_POINT('',(31.4825,35.,4.));
#27956=CARTESIAN_POINT('Ctrl Pts',(31.4811433043907,35.0029051520383,4.11258330249198));
#27957=CARTESIAN_POINT('Ctrl Pts',(31.4791554024968,35.227917919132,4.10238997204752));
#27958=CARTESIAN_POINT('Ctrl Pts',(31.4989360215654,35.4525827818457,4.09219664160306));
#27959=CARTESIAN_POINT('Ctrl Pts',(31.5417697834626,35.6727628942377,4.08200331115859));
#27960=CARTESIAN_POINT('Ctrl Pts',(31.761681751374,36.8031852448886,4.02966993537451));
#27961=CARTESIAN_POINT('Ctrl Pts',(32.5892464227109,37.815395051703,3.97733655959042));
#27962=CARTESIAN_POINT('Ctrl Pts',(33.6534212074435,38.2555631921955,3.92500318380634));
#27963=CARTESIAN_POINT('Ctrl Pts',(34.7175959921761,38.6957313326879,3.87266980802225));
#27964=CARTESIAN_POINT('Ctrl Pts',(36.0183808903044,38.5638578068583,3.82033643223817));
#27965=CARTESIAN_POINT('Ctrl Pts',(36.9725627531969,37.9190687430238,3.76800305645409));
#27966=CARTESIAN_POINT('Ctrl Pts',(37.9267446160893,37.2742796791893,3.71566968067));
#27967=CARTESIAN_POINT('Ctrl Pts',(38.5343234437459,36.1165750773498,3.66333630488592));
#27968=CARTESIAN_POINT('Ctrl Pts',(38.5228883542836,34.965017348136,3.61100292910183));
#27969=CARTESIAN_POINT('Ctrl Pts',(38.5114532648213,33.8134596189221,3.55866955331775));
#27970=CARTESIAN_POINT('Ctrl Pts',(37.8810042582401,32.6680487623339,3.50633617753366));
#27971=CARTESIAN_POINT('Ctrl Pts',(36.9142061709404,32.0423352319303,3.45400280174958));
#27972=CARTESIAN_POINT('Ctrl Pts',(35.9474080836407,31.4166217015266,3.40166942596549));
#27973=CARTESIAN_POINT('Ctrl Pts',(34.6442609156224,31.3106054973076,3.34933605018141));
#27974=CARTESIAN_POINT('Ctrl Pts',(33.5890369502264,31.7718194895137,3.29700267439732));
#27975=CARTESIAN_POINT('Ctrl Pts',(32.5338129848304,32.2330334817198,3.24466929861324));
#27976=CARTESIAN_POINT('Ctrl Pts',(31.7265122220568,33.2614776703508,3.19233592282916));
#27977=CARTESIAN_POINT('Ctrl Pts',(31.5290918320576,34.3960441771713,3.14000254704507));
#27978=CARTESIAN_POINT('Ctrl Pts',(31.4946134017248,34.5941902362662,3.13086279886071));
#27979=CARTESIAN_POINT('Ctrl Pts',(31.4787367991106,34.7955731089531,3.12172305067635));
#27980=CARTESIAN_POINT('Ctrl Pts',(31.48047694743,34.9972296622465,3.11258330249198));
#27981=CARTESIAN_POINT('Ctrl Pts',(31.4866348863052,34.9979909502101,3.38741669750802));
#27982=CARTESIAN_POINT('Ctrl Pts',(31.4842893061927,34.5578453627213,3.4072765672669));
#27983=CARTESIAN_POINT('Ctrl Pts',(31.5611193891505,34.1184886387468,3.42713643702577));
#27984=CARTESIAN_POINT('Ctrl Pts',(31.7209246555095,33.7117308512332,3.44699630678465));
#27985=CARTESIAN_POINT('Ctrl Pts',(32.1420326062756,32.6398704409937,3.49932968256873));
#27986=CARTESIAN_POINT('Ctrl Pts',(33.1393135913321,31.7943744371391,3.55166305835282));
#27987=CARTESIAN_POINT('Ctrl Pts',(34.2656318975588,31.5543250290031,3.6039964341369));
#27988=CARTESIAN_POINT('Ctrl Pts',(35.3919502037855,31.3142756208671,3.65632980992098));
#27989=CARTESIAN_POINT('Ctrl Pts',(36.6473058311824,31.6796728084497,3.70866318570507));
#27990=CARTESIAN_POINT('Ctrl Pts',(37.4688540624077,32.4866890097577,3.76099656148916));
#27991=CARTESIAN_POINT('Ctrl Pts',(38.2904022936331,33.2937052110658,3.81332993727324));
#27992=CARTESIAN_POINT('Ctrl Pts',(38.6781431286869,34.5423404260991,3.86566331305732));
#27993=CARTESIAN_POINT('Ctrl Pts',(38.4582311043207,35.6727630669474,3.91799668884141));
#27994=CARTESIAN_POINT('Ctrl Pts',(38.2383190799545,36.8031857077956,3.97033006462549));
#27995=CARTESIAN_POINT('Ctrl Pts',(37.4107541961682,37.8153957744587,4.02266344040958));
#27996=CARTESIAN_POINT('Ctrl Pts',(36.3465791382448,38.2555640279499,4.07499681619366));
#27997=CARTESIAN_POINT('Ctrl Pts',(35.2824040803214,38.6957322814412,4.12733019197775));
#27998=CARTESIAN_POINT('Ctrl Pts',(33.9816188482609,38.5638587217606,4.17966356776183));
#27999=CARTESIAN_POINT('Ctrl Pts',(33.0274367404146,37.9190694923971,4.23199694354592));
#28000=CARTESIAN_POINT('Ctrl Pts',(32.0828594910996,37.2807707529301,4.28380352819995));
#28001=CARTESIAN_POINT('Ctrl Pts',(31.4779426270586,36.1398304565742,4.33561011285398));
#28002=CARTESIAN_POINT('Ctrl Pts',(31.4769533103746,34.9997936499005,4.38741669750802));
#28003=CARTESIAN_POINT('Origin',(35.,35.,4.));
#28004=CARTESIAN_POINT('',(31.4861926565527,35.0022702467704,5.38741669750802));
#28005=CARTESIAN_POINT('',(31.4875431178521,34.9988611670469,5.11258330249198));
#28006=CARTESIAN_POINT('',(31.4825,35.,4.));
#28007=CARTESIAN_POINT('Ctrl Pts',(31.4875431178521,34.9988611670469,5.11258330249198));
#28008=CARTESIAN_POINT('Ctrl Pts',(31.4894883427227,35.6536666001145,5.08305689341869));
#28009=CARTESIAN_POINT('Ctrl Pts',(31.6654106307538,36.3094429302072,5.0535304843454));
#28010=CARTESIAN_POINT('Ctrl Pts',(32.0086471712983,36.8611218096429,5.02400407527211));
#28011=CARTESIAN_POINT('Ctrl Pts',(32.6170085475347,37.8389318114614,4.97167069948803));
#28012=CARTESIAN_POINT('Ctrl Pts',(33.7509866448637,38.4897202961854,4.91933732370394));
#28013=CARTESIAN_POINT('Ctrl Pts',(34.9021569461515,38.5217031223488,4.86700394791986));
#28014=CARTESIAN_POINT('Ctrl Pts',(36.0533272474394,38.5536859485121,4.81467057213577));
#28015=CARTESIAN_POINT('Ctrl Pts',(37.2216897526861,37.9668631161147,4.76233719635169));
#28016=CARTESIAN_POINT('Ctrl Pts',(37.8834035271664,37.0243394582438,4.71000382056761));
#28017=CARTESIAN_POINT('Ctrl Pts',(38.5451173016466,36.0818158003729,4.65767044478352));
#28018=CARTESIAN_POINT('Ctrl Pts',(38.7001823453603,34.7835913170285,4.60533706899944));
#28019=CARTESIAN_POINT('Ctrl Pts',(38.2790745026986,33.7117311819539,4.55300369321535));
#28020=CARTESIAN_POINT('Ctrl Pts',(37.857966660037,32.6398710468792,4.50067031743127));
#28021=CARTESIAN_POINT('Ctrl Pts',(36.860685931,31.7943752600742,4.44833694164718));
#28022=CARTESIAN_POINT('Ctrl Pts',(35.7343679139176,31.5543259135622,4.3960035658631));
#28023=CARTESIAN_POINT('Ctrl Pts',(34.6080498968352,31.3142765670502,4.34367019007902));
#28024=CARTESIAN_POINT('Ctrl Pts',(33.3526945917074,31.6796736608312,4.29133681429493));
#28025=CARTESIAN_POINT('Ctrl Pts',(32.5311465713864,32.4866896549654,4.23900343851085));
#28026=CARTESIAN_POINT('Ctrl Pts',(31.8696170922289,33.1365176103207,4.19686339317123));
#28027=CARTESIAN_POINT('Ctrl Pts',(31.4893614502066,34.0726843317691,4.15472334783161));
#28028=CARTESIAN_POINT('Ctrl Pts',(31.4811433043907,35.0029051520383,4.11258330249198));
#28029=CARTESIAN_POINT('Ctrl Pts',(31.4769533103746,34.9997936499005,4.38741669750802));
#28030=CARTESIAN_POINT('Ctrl Pts',(31.4769432505867,34.9882012764272,4.38794348863807));
#28031=CARTESIAN_POINT('Ctrl Pts',(31.476995634958,34.9766089963718,4.38847027976812));
#28032=CARTESIAN_POINT('Ctrl Pts',(31.4771107413343,34.9650173391525,4.38899707089817));
#28033=CARTESIAN_POINT('Ctrl Pts',(31.4885458337323,33.8134593143178,4.44133044668225));
#28034=CARTESIAN_POINT('Ctrl Pts',(32.1189950021604,32.6680481636951,4.49366382246634));
#28035=CARTESIAN_POINT('Ctrl Pts',(33.0857933376524,32.0423344726558,4.54599719825042));
#28036=CARTESIAN_POINT('Ctrl Pts',(34.0525916731444,31.4166207816165,4.59833057403451));
#28037=CARTESIAN_POINT('Ctrl Pts',(35.3557391757004,31.3106045501606,4.65066394981859));
#28038=CARTESIAN_POINT('Ctrl Pts',(36.4109634119899,31.7718186607773,4.70299732560267));
#28039=CARTESIAN_POINT('Ctrl Pts',(37.4661876482795,32.233032771394,4.75533070138676));
#28040=CARTESIAN_POINT('Ctrl Pts',(38.2734886183026,33.2614772240832,4.80766407717084));
#28041=CARTESIAN_POINT('Ctrl Pts',(38.4709090589814,34.3960440221467,4.85999745295493));
#28042=CARTESIAN_POINT('Ctrl Pts',(38.6683294996601,35.5306108202102,4.91233082873901));
#28043=CARTESIAN_POINT('Ctrl Pts',(38.2558694109946,36.771299963648,4.9646642045231));
#28044=CARTESIAN_POINT('Ctrl Pts',(37.4184572536729,37.5618425098028,5.01699758030718));
#28045=CARTESIAN_POINT('Ctrl Pts',(36.5810450963513,38.3523850559575,5.06933095609127));
#28046=CARTESIAN_POINT('Ctrl Pts',(35.3186808703736,38.6927810048293,5.12166433187535));
#28047=CARTESIAN_POINT('Ctrl Pts',(34.1973516288142,38.4304122279041,5.17399770765944));
#28048=CARTESIAN_POINT('Ctrl Pts',(33.0760223872548,38.168043450979,5.22633108344352));
#28049=CARTESIAN_POINT('Ctrl Pts',(32.0957281301138,37.302909948257,5.2786644592276));
#28050=CARTESIAN_POINT('Ctrl Pts',(31.6959884957425,36.2228984191863,5.33099783501169));
#28051=CARTESIAN_POINT('Ctrl Pts',(31.5523398513352,35.834790313921,5.34980412251047));
#28052=CARTESIAN_POINT('Ctrl Pts',(31.4836619352111,35.4189336360054,5.36861041000924));
#28053=CARTESIAN_POINT('Ctrl Pts',(31.4861926565527,35.0022702467704,5.38741669750802));
#28054=CARTESIAN_POINT('Origin',(35.,35.,4.));
#28055=CARTESIAN_POINT('',(31.4836963557363,34.997016753135,6.38741669750802));
#28056=CARTESIAN_POINT('',(31.4775764275568,34.998690818207,6.11258330249198));
#28057=CARTESIAN_POINT('',(31.4825,35.,4.));
#28058=CARTESIAN_POINT('Ctrl Pts',(31.4775764275568,34.998690818207,6.11258330249198));
#28059=CARTESIAN_POINT('Ctrl Pts',(31.4827872982739,36.074383472183,6.06372381478987));
#28060=CARTESIAN_POINT('Ctrl Pts',(32.0123599558151,37.1545218488605,6.01486432708775));
#28061=CARTESIAN_POINT('Ctrl Pts',(32.8684049695572,37.8050433721304,5.96600483938563));
#28062=CARTESIAN_POINT('Ctrl Pts',(33.7853144071958,38.5018166895356,5.91367146360154));
#28063=CARTESIAN_POINT('Ctrl Pts',(35.0767706487491,38.7057102384231,5.86133808781746));
#28064=CARTESIAN_POINT('Ctrl Pts',(36.1637432436869,38.3253071915374,5.80900471203338));
#28065=CARTESIAN_POINT('Ctrl Pts',(37.2507158386246,37.9449041446517,5.75667133624929));
#28066=CARTESIAN_POINT('Ctrl Pts',(38.1332047869467,36.9802045019929,5.70433796046521));
#28067=CARTESIAN_POINT('Ctrl Pts',(38.4155418609846,35.8637360634774,5.65200458468113));
#28068=CARTESIAN_POINT('Ctrl Pts',(38.6978789350226,34.7472676249618,5.59967120889704));
#28069=CARTESIAN_POINT('Ctrl Pts',(38.3800641347763,33.4790303905896,5.54733783311296));
#28070=CARTESIAN_POINT('Ctrl Pts',(37.604591287456,32.6276445643168,5.49500445732887));
#28071=CARTESIAN_POINT('Ctrl Pts',(36.8291184401356,31.7762587380439,5.44267108154479));
#28072=CARTESIAN_POINT('Ctrl Pts',(35.595987545741,31.3417243198703,5.3903377057607));
#28073=CARTESIAN_POINT('Ctrl Pts',(34.4580787374483,31.5188669221671,5.33800432997662));
#28074=CARTESIAN_POINT('Ctrl Pts',(33.3201699291557,31.6960095244639,5.28567095419254));
#28075=CARTESIAN_POINT('Ctrl Pts',(32.277483206965,32.4848291472311,5.23333757840845));
#28076=CARTESIAN_POINT('Ctrl Pts',(31.7975121734416,33.5316547180712,5.18100420262437));
#28077=CARTESIAN_POINT('Ctrl Pts',(31.5883400491575,33.9878629329714,5.15819723591357));
#28078=CARTESIAN_POINT('Ctrl Pts',(31.4860405755429,34.4930724110572,5.13539026920278));
#28079=CARTESIAN_POINT('Ctrl Pts',(31.4875431178521,34.9988611670469,5.11258330249198));
#28080=CARTESIAN_POINT('Ctrl Pts',(31.4861926565527,35.0022702467704,5.38741669750802));
#28081=CARTESIAN_POINT('Ctrl Pts',(31.4907043241454,34.2594596183014,5.42094378579333));
#28082=CARTESIAN_POINT('Ctrl Pts',(31.7215335296905,33.5140850744687,5.45447087407864));
#28083=CARTESIAN_POINT('Ctrl Pts',(32.1573641816635,32.9187998099572,5.48799796236395));
#28084=CARTESIAN_POINT('Ctrl Pts',(32.8376645135573,31.9896022852182,5.54033133814803));
#28085=CARTESIAN_POINT('Ctrl Pts',(34.0174501889464,31.4260967911598,5.59266471393211));
#28086=CARTESIAN_POINT('Ctrl Pts',(35.1677586650642,31.4809334902507,5.64499808971619));
#28087=CARTESIAN_POINT('Ctrl Pts',(36.318067141182,31.5357701893416,5.69733146550028));
#28088=CARTESIAN_POINT('Ctrl Pts',(37.4388984180285,32.2089490815819,5.74966484128437));
#28089=CARTESIAN_POINT('Ctrl Pts',(38.027722367947,33.1986476425792,5.80199821706845));
#28090=CARTESIAN_POINT('Ctrl Pts',(38.6165463178655,34.1883462035765,5.85433159285254));
#28091=CARTESIAN_POINT('Ctrl Pts',(38.6733629408561,35.4945644333309,5.90666496863662));
#28092=CARTESIAN_POINT('Ctrl Pts',(38.1726983287836,36.5316521939121,5.9589983444207));
#28093=CARTESIAN_POINT('Ctrl Pts',(37.6720337167111,37.5687399544933,6.01133172020479));
#28094=CARTESIAN_POINT('Ctrl Pts',(36.6138878695757,38.3366972459014,6.06366509598887));
#28095=CARTESIAN_POINT('Ctrl Pts',(35.4726853575398,38.491208604665,6.11599847177296));
#28096=CARTESIAN_POINT('Ctrl Pts',(34.3314828455038,38.6457199634287,6.16833184755704));
#28097=CARTESIAN_POINT('Ctrl Pts',(33.1072236685675,38.1867853895479,6.22066522334113));
#28098=CARTESIAN_POINT('Ctrl Pts',(32.3488106963438,37.3201666288988,6.27299859912521));
#28099=CARTESIAN_POINT('Ctrl Pts',(31.7960966856348,36.6885947168973,6.31113796525281));
#28100=CARTESIAN_POINT('Ctrl Pts',(31.490801080199,35.8404951819918,6.34927733138042));
#28101=CARTESIAN_POINT('Ctrl Pts',(31.4836963557363,34.997016753135,6.38741669750802));
#28102=CARTESIAN_POINT('Origin',(35.,35.,4.));
#28103=CARTESIAN_POINT('',(31.47826034488,35.0017653187145,7.38741669750802));
#28104=CARTESIAN_POINT('',(31.4846882532079,35.0028111988253,7.11258330249198));
#28105=CARTESIAN_POINT('',(31.4825,35.,4.));
#28106=CARTESIAN_POINT('',(37.6735319337713,37.2858331630075,8.));
#28107=CARTESIAN_POINT('Ctrl Pts',(31.47826034488,35.0017653187145,7.38741669750802));
#28108=CARTESIAN_POINT('Ctrl Pts',(31.4849539836961,33.9623976729958,7.43461100431976));
#28109=CARTESIAN_POINT('Ctrl Pts',(31.9746240526108,32.9177662403339,7.4818053111315));
#28110=CARTESIAN_POINT('Ctrl Pts',(32.7813938443113,32.2635129435208,7.52899961794324));
#28111=CARTESIAN_POINT('Ctrl Pts',(33.6760141816485,31.5380168836533,7.58133299372733));
#28112=CARTESIAN_POINT('Ctrl Pts',(34.9605532865631,31.292545720314,7.63366636951141));
#28113=CARTESIAN_POINT('Ctrl Pts',(36.0588773921206,31.639261394405,7.68599974529549));
#28114=CARTESIAN_POINT('Ctrl Pts',(37.1572014976782,31.985977068496,7.73833312107957));
#28115=CARTESIAN_POINT('Ctrl Pts',(38.0693106038786,32.9248795800174,7.79066649686366));
#28116=CARTESIAN_POINT('Ctrl Pts',(38.3863002982481,34.0300657119841,7.84299987264775));
#28117=CARTESIAN_POINT('Ctrl Pts',(38.7032899926177,35.1352518439507,7.89533324843183));
#28118=CARTESIAN_POINT('Ctrl Pts',(38.4251602751564,36.4067215963626,7.94766662421592));
#28119=CARTESIAN_POINT('Ctrl Pts',(37.6735319337713,37.2858331630076,8.));
#28120=CARTESIAN_POINT('',(32.321499452735,37.2890251664065,7.99999999999999));
#28121=CARTESIAN_POINT('Origin',(35.,35.,8.));
#28122=CARTESIAN_POINT('Ctrl Pts',(32.321476328717,37.2890400220486,8.));
#28123=CARTESIAN_POINT('Ctrl Pts',(33.0392492598742,38.1233257780545,7.95000212253755));
#28124=CARTESIAN_POINT('Ctrl Pts',(34.1813302937714,38.5989193684354,7.90000424507511));
#28125=CARTESIAN_POINT('Ctrl Pts',(35.278297796919,38.5118532074872,7.85000636761267));
#28126=CARTESIAN_POINT('Ctrl Pts',(36.4265067905564,38.4207200164352,7.79767299182859));
#28127=CARTESIAN_POINT('Ctrl Pts',(37.5252891335093,37.7131334793234,7.74533961604451));
#28128=CARTESIAN_POINT('Ctrl Pts',(38.0826702008662,36.7055536192858,7.69300624026042));
#28129=CARTESIAN_POINT('Ctrl Pts',(38.6400512682231,35.6979737592483,7.64067286447634));
#28130=CARTESIAN_POINT('Ctrl Pts',(38.6560310599838,34.390400576285,7.58833948869225));
#28131=CARTESIAN_POINT('Ctrl Pts',(38.1231127521292,33.3694814726124,7.53600611290816));
#28132=CARTESIAN_POINT('Ctrl Pts',(37.5901944442746,32.3485623689397,7.48367273712408));
#28133=CARTESIAN_POINT('Ctrl Pts',(36.5083780368047,31.6142973445577,7.43133936134));
#28134=CARTESIAN_POINT('Ctrl Pts',(35.3628660305036,31.4957037502949,7.37900598555592));
#28135=CARTESIAN_POINT('Ctrl Pts',(34.2173540242026,31.3771101560321,7.32667260977183));
#28136=CARTESIAN_POINT('Ctrl Pts',(33.0081464190704,31.8741879918886,7.27433923398774));
#28137=CARTESIAN_POINT('Ctrl Pts',(32.2773153573829,32.7641662925145,7.22200585820366));
#28138=CARTESIAN_POINT('Ctrl Pts',(31.7679565185591,33.3844441344804,7.18553167296643));
#28139=CARTESIAN_POINT('Ctrl Pts',(31.4909695616634,34.1955737681155,7.14905748772921));
#28140=CARTESIAN_POINT('Ctrl Pts',(31.4846882532079,35.0028111988253,7.11258330249198));
#28141=CARTESIAN_POINT('Origin',(-35.,35.,4.));
#28142=CARTESIAN_POINT('',(-38.5120268522747,34.9998626667344,0.387416697508021));
#28143=CARTESIAN_POINT('',(-38.5151985683976,34.9953484440209,0.112583302491983));
#28144=CARTESIAN_POINT('',(-38.5175,35.,4.));
#28145=CARTESIAN_POINT('',(-37.6735319337713,37.2858331630075,0.));
#28146=CARTESIAN_POINT('Ctrl Pts',(-38.5151985683976,34.9953484440209,0.112583302491983));
#28147=CARTESIAN_POINT('Ctrl Pts',(-38.508022599206,35.8232716101844,0.0750555349946553));
#28148=CARTESIAN_POINT('Ctrl Pts',(-38.2125174896864,36.6554305951821,0.0375277674973274));
#28149=CARTESIAN_POINT('Ctrl Pts',(-37.6735319337713,37.2858331630075,0.));
#28150=CARTESIAN_POINT('',(-32.3214993158099,37.289025066123,6.74947782880687E-15));
#28151=CARTESIAN_POINT('Origin',(-35.,35.,0.));
#28152=CARTESIAN_POINT('Ctrl Pts',(-32.3214761820288,37.2890399271607,4.52762827229947E-15));
#28153=CARTESIAN_POINT('Ctrl Pts',(-33.0392490750158,38.123325504421,0.0499978774624455));
#28154=CARTESIAN_POINT('Ctrl Pts',(-34.1813302139117,38.5989195898449,0.0999957549248864));
#28155=CARTESIAN_POINT('Ctrl Pts',(-35.2782977979761,38.5118535311589,0.149993632387327));
#28156=CARTESIAN_POINT('Ctrl Pts',(-36.42650687631,38.420720447146,0.202327008171411));
#28157=CARTESIAN_POINT('Ctrl Pts',(-37.5252892775753,37.7131335867401,0.254660383955495));
#28158=CARTESIAN_POINT('Ctrl Pts',(-38.0826703648835,36.7055536147166,0.30699375973958));
#28159=CARTESIAN_POINT('Ctrl Pts',(-38.368187486773,36.189423196523,0.333801405662393));
#28160=CARTESIAN_POINT('Ctrl Pts',(-38.511642203595,35.5945753060192,0.360609051585207));
#28161=CARTESIAN_POINT('Ctrl Pts',(-38.5120268522747,34.9998626667344,0.387416697508021));
#28162=CARTESIAN_POINT('Origin',(-35.,35.,4.));
#28163=CARTESIAN_POINT('',(-38.5212301417031,34.9978480330234,1.38741669750802));
#28164=CARTESIAN_POINT('',(-38.5220165881118,35.0016823567161,1.11258330249198));
#28165=CARTESIAN_POINT('',(-38.5175,35.,4.));
#28166=CARTESIAN_POINT('Ctrl Pts',(-38.5220165881118,35.0016823567161,1.11258330249198));
#28167=CARTESIAN_POINT('Ctrl Pts',(-38.5226066014871,35.1013890040059,1.10805583214991));
#28168=CARTESIAN_POINT('Ctrl Pts',(-38.5187309301454,35.2010488154761,1.10352836180785));
#28169=CARTESIAN_POINT('Ctrl Pts',(-38.5102390188272,35.3003133215195,1.09900089146578));
#28170=CARTESIAN_POINT('Ctrl Pts',(-38.4120803667407,36.4477193350987,1.04666751568169));
#28171=CARTESIAN_POINT('Ctrl Pts',(-37.6971355129363,37.5423077018709,0.994334139897609));
#28172=CARTESIAN_POINT('Ctrl Pts',(-36.6859404016511,38.0934400513324,0.942000764113524));
#28173=CARTESIAN_POINT('Ctrl Pts',(-35.6747452903659,38.6445724007939,0.88966738832944));
#28174=CARTESIAN_POINT('Ctrl Pts',(-34.3672999215998,38.6522487329447,0.837334012545356));
#28175=CARTESIAN_POINT('Ctrl Pts',(-33.3498298999919,38.1127743676805,0.785000636761271));
#28176=CARTESIAN_POINT('Ctrl Pts',(-32.332359878384,37.5733000024162,0.732667260977186));
#28177=CARTESIAN_POINT('Ctrl Pts',(-31.6048652039344,36.4866749397369,0.680333885193101));
#28178=CARTESIAN_POINT('Ctrl Pts',(-31.4934688910568,35.3406024624848,0.628000509409016));
#28179=CARTESIAN_POINT('Ctrl Pts',(-31.3820725781792,34.1945299852327,0.575667133624932));
#28180=CARTESIAN_POINT('Ctrl Pts',(-31.8867746268736,32.9890100934079,0.523333757840848));
#28181=CARTESIAN_POINT('Ctrl Pts',(-32.7813945002955,32.26351389125,0.471000382056763));
#28182=CARTESIAN_POINT('Ctrl Pts',(-33.6760143737173,31.5380176890922,0.418667006272678));
#28183=CARTESIAN_POINT('Ctrl Pts',(-34.9605520718666,31.2925451766014,0.366333630488594));
#28184=CARTESIAN_POINT('Ctrl Pts',(-36.0588768524004,31.6392614911932,0.31400025470451));
#28185=CARTESIAN_POINT('Ctrl Pts',(-37.1572016329341,31.9859778057849,0.261666878920425));
#28186=CARTESIAN_POINT('Ctrl Pts',(-38.0693134958523,32.9248829474593,0.209333503136341));
#28187=CARTESIAN_POINT('Ctrl Pts',(-38.3863031564079,34.0300688951037,0.157000127352256));
#28188=CARTESIAN_POINT('Ctrl Pts',(-38.4759825373922,34.3427364801714,0.142194519065498));
#28189=CARTESIAN_POINT('Ctrl Pts',(-38.5180296611061,34.6687128110693,0.127388910778741));
#28190=CARTESIAN_POINT('Ctrl Pts',(-38.5151985683976,34.9953484440209,0.112583302491983));
#28191=CARTESIAN_POINT('Ctrl Pts',(-38.5120268522747,34.9998626667344,0.387416697508021));
#28192=CARTESIAN_POINT('Ctrl Pts',(-38.5123931074215,34.4335886186821,0.412942427369291));
#28193=CARTESIAN_POINT('Ctrl Pts',(-38.3830450900788,33.8674371959539,0.438468157230563));
#28194=CARTESIAN_POINT('Ctrl Pts',(-38.1231128912653,33.3694814421284,0.463993887091834));
#28195=CARTESIAN_POINT('Ctrl Pts',(-37.5901945569878,32.348562325205,0.516327262875918));
#28196=CARTESIAN_POINT('Ctrl Pts',(-36.5083781150815,31.6142971749993,0.568660638660002));
#28197=CARTESIAN_POINT('Ctrl Pts',(-35.3628660558844,31.4957035546786,0.620994014444087));
#28198=CARTESIAN_POINT('Ctrl Pts',(-34.2173539966873,31.3771099343579,0.673327390228171));
#28199=CARTESIAN_POINT('Ctrl Pts',(-33.0081463201995,31.8741878439222,0.725660766012255));
#28200=CARTESIAN_POINT('Ctrl Pts',(-32.2773152209783,32.7641661988384,0.77799414179634));
#28201=CARTESIAN_POINT('Ctrl Pts',(-31.5464841217571,33.6541445537545,0.830327517580424));
#28202=CARTESIAN_POINT('Ctrl Pts',(-31.2940295998026,34.9370233540225,0.882660893364509));
#28203=CARTESIAN_POINT('Ctrl Pts',(-31.6331814964185,36.0375699846378,0.934994269148593));
#28204=CARTESIAN_POINT('Ctrl Pts',(-31.9723333930344,37.1381166152532,0.987327644932678));
#28205=CARTESIAN_POINT('Ctrl Pts',(-32.9030917082208,38.0563310762161,1.03966102071676));
#28206=CARTESIAN_POINT('Ctrl Pts',(-34.0081263071124,38.3805512169411,1.09199439650085));
#28207=CARTESIAN_POINT('Ctrl Pts',(-35.1131609060039,38.7047713576661,1.14432777228493));
#28208=CARTESIAN_POINT('Ctrl Pts',(-36.3924717886008,38.4349971781534,1.19666114806902));
#28209=CARTESIAN_POINT('Ctrl Pts',(-37.2724838028734,37.6921714555696,1.2489945238531));
#28210=CARTESIAN_POINT('Ctrl Pts',(-38.0483632745171,37.0372449093246,1.29513524840474));
#28211=CARTESIAN_POINT('Ctrl Pts',(-38.5138515465497,36.0145962191428,1.34127597295638));
#28212=CARTESIAN_POINT('Ctrl Pts',(-38.5212301417031,34.9978480330234,1.38741669750802));
#28213=CARTESIAN_POINT('Origin',(-35.,35.,4.));
#28214=CARTESIAN_POINT('',(-38.516961906974,35.0030273033746,2.38741669750802));
#28215=CARTESIAN_POINT('',(-38.512261546942,35.0007919713519,2.11258330249198));
#28216=CARTESIAN_POINT('',(-38.5175,35.,4.));
#28217=CARTESIAN_POINT('Ctrl Pts',(-38.512261546942,35.0007919713519,2.11258330249198));
#28218=CARTESIAN_POINT('Ctrl Pts',(-38.513350743052,35.5300199732952,2.08872275352109));
#28219=CARTESIAN_POINT('Ctrl Pts',(-38.400967605409,36.0588087668393,2.06486220455019));
#28220=CARTESIAN_POINT('Ctrl Pts',(-38.1726977821637,36.5316519312173,2.0410016555793));
#28221=CARTESIAN_POINT('Ctrl Pts',(-37.6720332561867,37.568739511998,1.98866827979521));
#28222=CARTESIAN_POINT('Ctrl Pts',(-36.6138875906958,38.3366966664809,1.93633490401113));
#28223=CARTESIAN_POINT('Ctrl Pts',(-35.472685275733,38.4912080005995,1.88400152822705));
#28224=CARTESIAN_POINT('Ctrl Pts',(-34.3314829607702,38.6457193347182,1.83166815244296));
#28225=CARTESIAN_POINT('Ctrl Pts',(-33.1072239963354,38.1867848484726,1.77933477665888));
#28226=CARTESIAN_POINT('Ctrl Pts',(-32.3488111539779,37.3201662335233,1.72700140087479));
#28227=CARTESIAN_POINT('Ctrl Pts',(-31.5903983116205,36.453547618574,1.67466802509071));
#28228=CARTESIAN_POINT('Ctrl Pts',(-31.2978315913404,35.179244874921,1.62233464930662));
#28229=CARTESIAN_POINT('Ctrl Pts',(-31.6022838952552,34.0686053777681,1.57000127352254));
#28230=CARTESIAN_POINT('Ctrl Pts',(-31.90673619917,32.9579658806151,1.51766789773845));
#28231=CARTESIAN_POINT('Ctrl Pts',(-32.8082075272796,32.0109896299622,1.46533452195437));
#28232=CARTESIAN_POINT('Ctrl Pts',(-33.9025204773781,31.6522426059455,1.41300114617028));
#28233=CARTESIAN_POINT('Ctrl Pts',(-34.9968334274766,31.2934955819288,1.3606677703862));
#28234=CARTESIAN_POINT('Ctrl Pts',(-36.283987999564,31.5229777845482,1.30833439460212));
#28235=CARTESIAN_POINT('Ctrl Pts',(-37.1868790604233,32.2378307160511,1.25600101881803));
#28236=CARTESIAN_POINT('Ctrl Pts',(-38.0116591177612,32.8908402178529,1.20819511337602));
#28237=CARTESIAN_POINT('Ctrl Pts',(-38.5157865917788,33.94887224596,1.160389207934));
#28238=CARTESIAN_POINT('Ctrl Pts',(-38.5220165881118,35.0016823567161,1.11258330249198));
#28239=CARTESIAN_POINT('Ctrl Pts',(-38.5212301417031,34.9978480330234,1.38741669750802));
#28240=CARTESIAN_POINT('Ctrl Pts',(-38.5222204396842,34.8613879542309,1.39360934874046));
#28241=CARTESIAN_POINT('Ctrl Pts',(-38.5149588389545,34.7250341608202,1.39980199997291));
#28242=CARTESIAN_POINT('Ctrl Pts',(-38.499088221748,34.5896899066556,1.40599465120535));
#28243=CARTESIAN_POINT('Ctrl Pts',(-38.3649674804015,33.4459113459803,1.45832802698944));
#28244=CARTESIAN_POINT('Ctrl Pts',(-37.6160128517601,32.3742314902846,1.51066140277352));
#28245=CARTESIAN_POINT('Ctrl Pts',(-36.5880242056904,31.8551402422105,1.56299477855761));
#28246=CARTESIAN_POINT('Ctrl Pts',(-35.5600355596207,31.3360489941365,1.61532815434169));
#28247=CARTESIAN_POINT('Ctrl Pts',(-34.2530128961227,31.3695463536841,1.66766153012578));
#28248=CARTESIAN_POINT('Ctrl Pts',(-33.2529648698024,31.9406150594439,1.71999490590986));
#28249=CARTESIAN_POINT('Ctrl Pts',(-32.2529168434821,32.5116837652037,1.77232828169395));
#28250=CARTESIAN_POINT('Ctrl Pts',(-31.5598434543395,33.6203238171756,1.82466165747803));
#28251=CARTESIAN_POINT('Ctrl Pts',(-31.4844880896413,34.7694704150121,1.87699503326211));
#28252=CARTESIAN_POINT('Ctrl Pts',(-31.4091327249431,35.9186170128485,1.9293284090462));
#28253=CARTESIAN_POINT('Ctrl Pts',(-31.9514953846893,37.1082701565493,1.98166178483028));
#28254=CARTESIAN_POINT('Ctrl Pts',(-32.8684048665688,37.8050435076812,2.03399516061437));
#28255=CARTESIAN_POINT('Ctrl Pts',(-33.7853143484484,38.5018168588132,2.08632853639845));
#28256=CARTESIAN_POINT('Ctrl Pts',(-35.0767706524612,38.7057104173762,2.13866191218254));
#28257=CARTESIAN_POINT('Ctrl Pts',(-36.1637432999128,38.325307352079,2.19099528796662));
#28258=CARTESIAN_POINT('Ctrl Pts',(-37.2507159473644,37.9449042867818,2.24332866375071));
#28259=CARTESIAN_POINT('Ctrl Pts',(-38.1332049382548,36.9802045976245,2.29566203953479));
#28260=CARTESIAN_POINT('Ctrl Pts',(-38.4155420259161,35.8637361052132,2.34799541531887));
#28261=CARTESIAN_POINT('Ctrl Pts',(-38.4864342614375,35.5834011765932,2.36113584271526));
#28262=CARTESIAN_POINT('Ctrl Pts',(-38.5194889764144,35.2934977450987,2.37427627011164));
#28263=CARTESIAN_POINT('Ctrl Pts',(-38.516961906974,35.0030273033746,2.38741669750802));
#28264=CARTESIAN_POINT('Origin',(-35.,35.,4.));
#28265=CARTESIAN_POINT('',(-38.5133643814276,34.9979909506281,3.38741669750802));
#28266=CARTESIAN_POINT('',(-38.5195233495341,34.9972296620149,3.11258330249199));
#28267=CARTESIAN_POINT('',(-38.5175,35.,4.));
#28268=CARTESIAN_POINT('Ctrl Pts',(-38.5195233495341,34.9972296620149,3.11258330249199));
#28269=CARTESIAN_POINT('Ctrl Pts',(-38.5112995644464,35.9502404698791,3.06938967489226));
#28270=CARTESIAN_POINT('Ctrl Pts',(-38.1096192565637,36.9093637226591,3.02619604729254));
#28271=CARTESIAN_POINT('Ctrl Pts',(-37.4184568368782,37.5618420683218,2.98300241969282));
#28272=CARTESIAN_POINT('Ctrl Pts',(-36.581044823874,38.3523844782111,2.93066904390873));
#28273=CARTESIAN_POINT('Ctrl Pts',(-35.3186808154442,38.6927803683205,2.87833566812465));
#28274=CARTESIAN_POINT('Ctrl Pts',(-34.1973517671389,38.4304116366569,2.82600229234057));
#28275=CARTESIAN_POINT('Ctrl Pts',(-33.0760227188335,38.1680429049932,2.77366891655648));
#28276=CARTESIAN_POINT('Ctrl Pts',(-32.0957286306525,37.3029095515566,2.7213355407724));
#28277=CARTESIAN_POINT('Ctrl Pts',(-31.6959890651629,36.2228982085294,2.66900216498831));
#28278=CARTESIAN_POINT('Ctrl Pts',(-31.2962494996734,35.1428868655023,2.61666878920423));
#28279=CARTESIAN_POINT('Ctrl Pts',(-31.4770644568753,33.8479975328846,2.56433541342014));
#28280=CARTESIAN_POINT('Ctrl Pts',(-32.1573646715461,32.9188001684451,2.51200203763606));
#28281=CARTESIAN_POINT('Ctrl Pts',(-32.837664886217,31.9896028040056,2.45966866185197));
#28282=CARTESIAN_POINT('Ctrl Pts',(-34.0174503583568,31.4260974077442,2.40733528606789));
#28283=CARTESIAN_POINT('Ctrl Pts',(-35.1677586361884,31.4809340970796,2.3550019102838));
#28284=CARTESIAN_POINT('Ctrl Pts',(-36.3180669140201,31.535770786415,2.30266853449972));
#28285=CARTESIAN_POINT('Ctrl Pts',(-37.4388979975435,32.2089495613471,2.25033515871564));
#28286=CARTESIAN_POINT('Ctrl Pts',(-38.0277218460737,33.1986479523525,2.19800178293155));
#28287=CARTESIAN_POINT('Ctrl Pts',(-38.3480810663893,33.737109506995,2.16952895611836));
#28288=CARTESIAN_POINT('Ctrl Pts',(-38.5109618076844,34.3692634485841,2.14105612930517));
#28289=CARTESIAN_POINT('Ctrl Pts',(-38.512261546942,35.0007919713519,2.11258330249198));
#28290=CARTESIAN_POINT('Ctrl Pts',(-38.516961906974,35.0030273033746,2.38741669750802));
#28291=CARTESIAN_POINT('Ctrl Pts',(-38.5094246101142,34.1366633193706,2.42660964589572));
#28292=CARTESIAN_POINT('Ctrl Pts',(-38.1853502176079,33.2652551878002,2.46580259428343));
#28293=CARTESIAN_POINT('Ctrl Pts',(-37.6045914132455,32.6276444497373,2.50499554267113));
#28294=CARTESIAN_POINT('Ctrl Pts',(-36.8291185284818,31.7762585823377,2.55732891845521));
#28295=CARTESIAN_POINT('Ctrl Pts',(-35.5959875745222,31.3417241432036,2.6096622942393));
#28296=CARTESIAN_POINT('Ctrl Pts',(-34.4580787112737,31.5188667540608,2.66199567002338));
#28297=CARTESIAN_POINT('Ctrl Pts',(-33.3201698480253,31.6960093649181,2.71432904580747));
#28298=CARTESIAN_POINT('Ctrl Pts',(-32.277483075488,32.4848290257668,2.76666242159155));
#28299=CARTESIAN_POINT('Ctrl Pts',(-31.7975120187873,33.5316546471577,2.81899579737563));
#28300=CARTESIAN_POINT('Ctrl Pts',(-31.3175409620866,34.5784802685486,2.87132917315972));
#28301=CARTESIAN_POINT('Ctrl Pts',(-31.4002856212225,35.8833118504819,2.9236625489438));
#28302=CARTESIAN_POINT('Ctrl Pts',(-32.0086470268372,36.8611218995229,2.97599592472789));
#28303=CARTESIAN_POINT('Ctrl Pts',(-32.617008432452,37.8389319485639,3.02832930051197));
#28304=CARTESIAN_POINT('Ctrl Pts',(-33.7509865845457,38.4897204647128,3.08066267629606));
#28305=CARTESIAN_POINT('Ctrl Pts',(-34.902156941427,38.5217032924198,3.13299605208014));
#28306=CARTESIAN_POINT('Ctrl Pts',(-36.0533272983083,38.5536861201269,3.18532942786423));
#28307=CARTESIAN_POINT('Ctrl Pts',(-37.2216898599771,37.9668632593921,3.23766280364831));
#28308=CARTESIAN_POINT('Ctrl Pts',(-37.8834036664129,37.0243395560048,3.2899961794324));
#28309=CARTESIAN_POINT('Ctrl Pts',(-38.2940052559017,36.439491957273,3.3224696854576));
#28310=CARTESIAN_POINT('Ctrl Pts',(-38.5095290494265,35.7176868792413,3.35494319148281));
#28311=CARTESIAN_POINT('Ctrl Pts',(-38.5133643814276,34.9979909506281,3.38741669750802));
#28312=CARTESIAN_POINT('Origin',(-35.,35.,4.));
#28313=CARTESIAN_POINT('',(-38.5230459553398,34.9997936499459,4.38741669750802));
#28314=CARTESIAN_POINT('',(-38.5188569925171,35.0029051522836,4.11258330249198));
#28315=CARTESIAN_POINT('',(-38.5175,35.,4.));
#28316=CARTESIAN_POINT('Ctrl Pts',(-38.5188569925171,35.0029051522836,4.11258330249198));
#28317=CARTESIAN_POINT('Ctrl Pts',(-38.5208448945788,35.2279179383631,4.10238997204752));
#28318=CARTESIAN_POINT('Ctrl Pts',(-38.5010642738412,35.4525828200332,4.09219664160306));
#28319=CARTESIAN_POINT('Ctrl Pts',(-38.4582305083298,35.6727629510031,4.08200331115859));
#28320=CARTESIAN_POINT('Ctrl Pts',(-38.2383185218631,36.8031853970347,4.02966993537451));
#28321=CARTESIAN_POINT('Ctrl Pts',(-37.4107537806994,37.8153952892549,3.97733655959042));
#28322=CARTESIAN_POINT('Ctrl Pts',(-36.3465789061757,38.2555634668873,3.92500318380634));
#28323=CARTESIAN_POINT('Ctrl Pts',(-35.282404031652,38.6957316445196,3.87266980802226));
#28324=CARTESIAN_POINT('Ctrl Pts',(-33.9816190237685,38.5638581075641,3.82033643223817));
#28325=CARTESIAN_POINT('Ctrl Pts',(-33.0274370803658,37.9190689893243,3.76800305645409));
#28326=CARTESIAN_POINT('Ctrl Pts',(-32.0732551369631,37.2742798710845,3.71566968067));
#28327=CARTESIAN_POINT('Ctrl Pts',(-31.4656762580412,36.1165751715604,3.66333630488592));
#28328=CARTESIAN_POINT('Ctrl Pts',(-31.4771113484684,34.9650173451833,3.61100292910183));
#28329=CARTESIAN_POINT('Ctrl Pts',(-31.4885464388956,33.8134595188062,3.55866955331775));
#28330=CARTESIAN_POINT('Ctrl Pts',(-32.1189954986718,32.6680485655762,3.50633617753366));
#28331=CARTESIAN_POINT('Ctrl Pts',(-33.0857936675462,32.0423349823756,3.45400280174958));
#28332=CARTESIAN_POINT('Ctrl Pts',(-34.0525918364206,31.4166213991749,3.40166942596549));
#28333=CARTESIAN_POINT('Ctrl Pts',(-35.3557391143932,31.3106051860038,3.34933605018141));
#28334=CARTESIAN_POINT('Ctrl Pts',(-36.4109631688252,31.7718192171285,3.29700267439732));
#28335=CARTESIAN_POINT('Ctrl Pts',(-37.4661872232571,32.2330332482532,3.24466929861324));
#28336=CARTESIAN_POINT('Ctrl Pts',(-38.2734880541485,33.2614775236738,3.19233592282916));
#28337=CARTESIAN_POINT('Ctrl Pts',(-38.4709084608049,34.3960441262186,3.14000254704507));
#28338=CARTESIAN_POINT('Ctrl Pts',(-38.5053868940467,34.5941902020313,3.13086279886071));
#28339=CARTESIAN_POINT('Ctrl Pts',(-38.5212634980004,34.7955730917084,3.12172305067635));
#28340=CARTESIAN_POINT('Ctrl Pts',(-38.5195233495341,34.9972296620149,3.11258330249199));
#28341=CARTESIAN_POINT('Ctrl Pts',(-38.5133643814276,34.9979909506281,3.38741669750802));
#28342=CARTESIAN_POINT('Ctrl Pts',(-38.5157099610507,34.5578454548766,3.4072765672669));
#28343=CARTESIAN_POINT('Ctrl Pts',(-38.4388798941057,34.1184888224752,3.42713643702577));
#28344=CARTESIAN_POINT('Ctrl Pts',(-38.2790746610536,33.7117311197398,3.44699630678465));
#28345=CARTESIAN_POINT('Ctrl Pts',(-37.8579667980557,32.6398709329021,3.49932968256873));
#28346=CARTESIAN_POINT('Ctrl Pts',(-36.8606860208572,31.7943751052665,3.55166305835282));
#28347=CARTESIAN_POINT('Ctrl Pts',(-35.734367949382,31.554325747162,3.6039964341369));
#28348=CARTESIAN_POINT('Ctrl Pts',(-34.6080498779068,31.3142763890575,3.65632980992099));
#28349=CARTESIAN_POINT('Ctrl Pts',(-33.3526945121549,31.6796735004841,3.70866318570507));
#28350=CARTESIAN_POINT('Ctrl Pts',(-32.5311464521593,32.4866895335911,3.76099656148916));
#28351=CARTESIAN_POINT('Ctrl Pts',(-31.7095983921637,33.2937055666981,3.81332993727324));
#28352=CARTESIAN_POINT('Ctrl Pts',(-31.3218576379244,34.5423405214855,3.86566331305732));
#28353=CARTESIAN_POINT('Ctrl Pts',(-31.5417696164559,35.6727629267273,3.91799668884141));
#28354=CARTESIAN_POINT('Ctrl Pts',(-31.7616815949873,36.8031853319691,3.97033006462549));
#28355=CARTESIAN_POINT('Ctrl Pts',(-32.5892463062895,37.8153951876653,4.02266344040958));
#28356=CARTESIAN_POINT('Ctrl Pts',(-33.6534211424138,38.2555633494147,4.07499681619366));
#28357=CARTESIAN_POINT('Ctrl Pts',(-34.7175959785381,38.6957315111641,4.12733019197775));
#28358=CARTESIAN_POINT('Ctrl Pts',(-36.0183809394846,38.5638579789666,4.17966356776183));
#28359=CARTESIAN_POINT('Ctrl Pts',(-36.9725628484569,37.9190688839933,4.23199694354592));
#28360=CARTESIAN_POINT('Ctrl Pts',(-37.9171399008999,37.2807702775639,4.28380352819995));
#28361=CARTESIAN_POINT('Ctrl Pts',(-38.5220566388619,36.1398302190111,4.33561011285399));
#28362=CARTESIAN_POINT('Ctrl Pts',(-38.5230459553398,34.9997936499459,4.38741669750802));
#28363=CARTESIAN_POINT('Origin',(-35.,35.,4.));
#28364=CARTESIAN_POINT('',(-38.5138066110977,35.0022702462197,5.38741669750802));
#28365=CARTESIAN_POINT('',(-38.5124571785126,34.9988611669454,5.11258330249198));
#28366=CARTESIAN_POINT('',(-38.5175,35.,4.));
#28367=CARTESIAN_POINT('Ctrl Pts',(-38.5124571785126,34.9988611669454,5.11258330249198));
#28368=CARTESIAN_POINT('Ctrl Pts',(-38.5105119534794,35.6536666552656,5.08305689341869));
#28369=CARTESIAN_POINT('Ctrl Pts',(-38.3345896506072,36.3094430406945,5.0535304843454));
#28370=CARTESIAN_POINT('Ctrl Pts',(-37.9913530811025,36.8611219666803,5.02400407527211));
#28371=CARTESIAN_POINT('Ctrl Pts',(-37.3829916535365,37.8389320510055,4.97167069948803));
#28372=CARTESIAN_POINT('Ctrl Pts',(-36.2490134605232,38.4897205906347,4.91933732370395));
#28373=CARTESIAN_POINT('Ctrl Pts',(-35.0978430621031,38.5217034194952,4.86700394791986));
#28374=CARTESIAN_POINT('Ctrl Pts',(-33.946672663683,38.5536862483557,4.81467057213578));
#28375=CARTESIAN_POINT('Ctrl Pts',(-32.7783100598561,37.9668633664475,4.76233719635169));
#28376=CARTESIAN_POINT('Ctrl Pts',(-32.1165962295435,37.0243396290507,4.71000382056761));
#28377=CARTESIAN_POINT('Ctrl Pts',(-31.4548823992308,36.081815891654,4.65767044478352));
#28378=CARTESIAN_POINT('Ctrl Pts',(-31.2998173424323,34.7835912987687,4.60533706899944));
#28379=CARTESIAN_POINT('Ctrl Pts',(-31.7209252206252,33.7117310732541,4.55300369321535));
#28380=CARTESIAN_POINT('Ctrl Pts',(-32.1420330988181,32.6398708477396,4.50067031743127));
#28381=CARTESIAN_POINT('Ctrl Pts',(-33.1393139120024,31.7943749895958,4.44833694164718));
#28382=CARTESIAN_POINT('Ctrl Pts',(-34.2656320241194,31.5543256228295,4.3960035658631));
#28383=CARTESIAN_POINT('Ctrl Pts',(-35.3919501362363,31.3142762560632,4.34367019007901));
#28384=CARTESIAN_POINT('Ctrl Pts',(-36.647305547286,31.6796733806745,4.29133681429493));
#28385=CARTESIAN_POINT('Ctrl Pts',(-37.4688536369261,32.4866894429016,4.23900343851085));
#28386=CARTESIAN_POINT('Ctrl Pts',(-38.1303831719009,33.1365174530869,4.19686339317123));
#28387=CARTESIAN_POINT('Ctrl Pts',(-38.5106388460078,34.0726842535258,4.15472334783161));
#28388=CARTESIAN_POINT('Ctrl Pts',(-38.5188569925171,35.0029051522836,4.11258330249198));
#28389=CARTESIAN_POINT('Ctrl Pts',(-38.5230459553398,34.9997936499459,4.38741669750802));
#28390=CARTESIAN_POINT('Ctrl Pts',(-38.5230560151256,34.9882012788887,4.38794348863807));
#28391=CARTESIAN_POINT('Ctrl Pts',(-38.5230036307651,34.9766090012494,4.38847027976812));
#28392=CARTESIAN_POINT('Ctrl Pts',(-38.5228885244128,34.9650173464461,4.38899707089817));
#28393=CARTESIAN_POINT('Ctrl Pts',(-38.5114534343983,33.813459561621,4.44133044668225));
#28394=CARTESIAN_POINT('Ctrl Pts',(-37.881004397371,32.66804864972,4.49366382246634));
#28395=CARTESIAN_POINT('Ctrl Pts',(-36.9142062633822,32.0423350890982,4.54599719825042));
#28396=CARTESIAN_POINT('Ctrl Pts',(-35.9474081293934,31.4166215284763,4.59833057403451));
#28397=CARTESIAN_POINT('Ctrl Pts',(-34.6442608984431,31.3106053191336,4.65066394981859));
#28398=CARTESIAN_POINT('Ctrl Pts',(-33.5890368820876,31.7718193336147,4.70299732560267));
#28399=CARTESIAN_POINT('Ctrl Pts',(-32.533812865732,32.2330333480957,4.75533070138676));
#28400=CARTESIAN_POINT('Ctrl Pts',(-31.7265120639713,33.2614775864005,4.80766407717084));
#28401=CARTESIAN_POINT('Ctrl Pts',(-31.5290916644384,34.3960441480086,4.85999745295493));
#28402=CARTESIAN_POINT('Ctrl Pts',(-31.3316712649055,35.5306107096167,4.91233082873901));
#28403=CARTESIAN_POINT('Ctrl Pts',(-31.7441312676005,36.771299594528,4.9646642045231));
#28404=CARTESIAN_POINT('Ctrl Pts',(-32.5815432503882,37.5618419758867,5.01699758030718));
#28405=CARTESIAN_POINT('Ctrl Pts',(-33.418955233176,38.3523843572453,5.06933095609127));
#28406=CARTESIAN_POINT('Ctrl Pts',(-34.6813191960565,38.6927802350512,5.12166433187535));
#28407=CARTESIAN_POINT('Ctrl Pts',(-35.8026482038993,38.4304115128643,5.17399770765944));
#28408=CARTESIAN_POINT('Ctrl Pts',(-36.9239772117421,38.1680427906774,5.22633108344352));
#28409=CARTESIAN_POINT('Ctrl Pts',(-37.9042712645471,37.3029094684976,5.2786644592276));
#28410=CARTESIAN_POINT('Ctrl Pts',(-38.3040108156146,36.2228981644233,5.33099783501169));
#28411=CARTESIAN_POINT('Ctrl Pts',(-38.4476594300862,35.8347901400117,5.34980412251047));
#28412=CARTESIAN_POINT('Ctrl Pts',(-38.5163373319043,35.4189335486904,5.36861041000924));
#28413=CARTESIAN_POINT('Ctrl Pts',(-38.5138066110977,35.0022702462197,5.38741669750802));
#28414=CARTESIAN_POINT('Origin',(-35.,35.,4.));
#28415=CARTESIAN_POINT('',(-38.5163029138352,34.997016742257,6.38741669750802));
#28416=CARTESIAN_POINT('',(-38.5224238694764,34.9986908177615,6.11258330249199));
#28417=CARTESIAN_POINT('',(-38.5175,35.,4.));
#28418=CARTESIAN_POINT('Ctrl Pts',(-38.5224238694764,34.9986908177615,6.11258330249199));
#28419=CARTESIAN_POINT('Ctrl Pts',(-38.5172129982537,36.0743835623573,6.06372381478987));
#28420=CARTESIAN_POINT('Ctrl Pts',(-37.9876402962914,37.154522030678,6.01486432708775));
#28421=CARTESIAN_POINT('Ctrl Pts',(-37.1315952103829,37.8050436089632,5.96600483938563));
#28422=CARTESIAN_POINT('Ctrl Pts',(-36.2146856954469,38.5018169852953,5.91367146360155));
#28423=CARTESIAN_POINT('Ctrl Pts',(-34.9232293447652,38.705710551088,5.86133808781746));
#28424=CARTESIAN_POINT('Ctrl Pts',(-33.8362566580758,38.325307472034,5.80900471203338));
#28425=CARTESIAN_POINT('Ctrl Pts',(-32.7492839713864,37.9449043929801,5.75667133624929));
#28426=CARTESIAN_POINT('Ctrl Pts',(-31.8667949486893,36.9802046690794,5.70433796046521));
#28427=CARTESIAN_POINT('Ctrl Pts',(-31.5844578508488,35.8637361363978,5.65200458468113));
#28428=CARTESIAN_POINT('Ctrl Pts',(-31.3021207530084,34.7472676037162,5.59967120889704));
#28429=CARTESIAN_POINT('Ctrl Pts',(-31.6199355800247,33.4790302622538,5.54733783311296));
#28430=CARTESIAN_POINT('Ctrl Pts',(-32.3954084927658,32.6276443641247,5.49500445732887));
#28431=CARTESIAN_POINT('Ctrl Pts',(-33.1708814055069,31.7762584659956,5.44267108154479));
#28432=CARTESIAN_POINT('Ctrl Pts',(-34.4040124039728,31.3417240112,5.39033770576071));
#28433=CARTESIAN_POINT('Ctrl Pts',(-35.5419213082836,31.5188666284535,5.33800432997662));
#28434=CARTESIAN_POINT('Ctrl Pts',(-36.6798302125945,31.6960092457071,5.28567095419254));
#28435=CARTESIAN_POINT('Ctrl Pts',(-37.7225170227502,32.4848289350099,5.23333757840845));
#28436=CARTESIAN_POINT('Ctrl Pts',(-38.2024880967687,33.5316545941719,5.18100420262437));
#28437=CARTESIAN_POINT('Ctrl Pts',(-38.4116602387006,33.987862847563,5.15819723591357));
#28438=CARTESIAN_POINT('Ctrl Pts',(-38.5139597209473,34.4930723682773,5.13539026920278));
#28439=CARTESIAN_POINT('Ctrl Pts',(-38.5124571785126,34.9988611669454,5.11258330249198));
#28440=CARTESIAN_POINT('Ctrl Pts',(-38.5138066110977,35.0022702462197,5.38741669750802));
#28441=CARTESIAN_POINT('Ctrl Pts',(-38.5092949444589,34.2594597724306,5.42094378579333));
#28442=CARTESIAN_POINT('Ctrl Pts',(-38.2784657870358,33.5140853838181,5.45447087407863));
#28443=CARTESIAN_POINT('Ctrl Pts',(-37.8426352258847,32.9188002435034,5.48799796236394));
#28444=CARTESIAN_POINT('Ctrl Pts',(-37.1623350357574,31.9896029126267,5.54033133814803));
#28445=CARTESIAN_POINT('Ctrl Pts',(-35.9825496061728,31.4260975368425,5.59266471393211));
#28446=CARTESIAN_POINT('Ctrl Pts',(-34.8322413698574,31.4809342241349,5.6449980897162));
#28447=CARTESIAN_POINT('Ctrl Pts',(-33.681933133542,31.5357709114273,5.69733146550028));
#28448=CARTESIAN_POINT('Ctrl Pts',(-32.5611020904959,32.2089496617965,5.74966484128436));
#28449=CARTESIAN_POINT('Ctrl Pts',(-31.9722782631938,33.1986480172104,5.80199821706845));
#28450=CARTESIAN_POINT('Ctrl Pts',(-31.3834544358917,34.1883463726244,5.85433159285253));
#28451=CARTESIAN_POINT('Ctrl Pts',(-31.3266378243335,35.4945643330831,5.90666496863662));
#28452=CARTESIAN_POINT('Ctrl Pts',(-31.8273023322845,36.531651876217,5.95899834442071));
#28453=CARTESIAN_POINT('Ctrl Pts',(-32.3279668402356,37.5687394193509,6.01133172020479));
#28454=CARTESIAN_POINT('Ctrl Pts',(-33.3861124676959,38.3366965451598,6.06366509598887));
#28455=CARTESIAN_POINT('Ctrl Pts',(-34.5273147413959,38.4912078741205,6.11599847177296));
#28456=CARTESIAN_POINT('Ctrl Pts',(-35.668517015096,38.6457192030811,6.16833184755704));
#28457=CARTESIAN_POINT('Ctrl Pts',(-36.8927759350357,38.1867847351935,6.22066522334113));
#28458=CARTESIAN_POINT('Ctrl Pts',(-37.6511887502036,37.3201661507465,6.27299859912521));
#28459=CARTESIAN_POINT('Ctrl Pts',(-38.2039026464539,36.688594367157,6.31113796525282));
#28460=CARTESIAN_POINT('Ctrl Pts',(-38.5091981905113,35.8404949979527,6.34927733138042));
#28461=CARTESIAN_POINT('Ctrl Pts',(-38.5163029138352,34.997016742257,6.38741669750802));
#28462=CARTESIAN_POINT('Origin',(-35.,35.,4.));
#28463=CARTESIAN_POINT('',(-38.521739013009,35.0017650567249,7.38741669750802));
#28464=CARTESIAN_POINT('',(-38.5153120432796,35.002811202661,7.11258330249199));
#28465=CARTESIAN_POINT('',(-38.5175,35.,4.));
#28466=CARTESIAN_POINT('',(-32.3264680662287,37.2858331630075,8.));
#28467=CARTESIAN_POINT('Ctrl Pts',(-38.521739013009,35.0017650567249,7.38741669750802));
#28468=CARTESIAN_POINT('Ctrl Pts',(-38.515045138314,33.9623979425516,7.43461100431976));
#28469=CARTESIAN_POINT('Ctrl Pts',(-38.025374647688,32.917767542155,7.4818053111315));
#28470=CARTESIAN_POINT('Ctrl Pts',(-37.2186053621485,32.2635140899837,7.52899961794324));
#28471=CARTESIAN_POINT('Ctrl Pts',(-36.3239855860891,31.5380178578407,7.58133299372732));
#28472=CARTESIAN_POINT('Ctrl Pts',(-35.039448183402,31.2925450618756,7.63366636951141));
#28473=CARTESIAN_POINT('Ctrl Pts',(-33.9411232613757,31.6392615106971,7.68599974529549));
#28474=CARTESIAN_POINT('Ctrl Pts',(-32.8427983393495,31.9859779595187,7.73833312107958));
#28475=CARTESIAN_POINT('Ctrl Pts',(-31.9306858979841,32.9248836531268,7.79066649686366));
#28476=CARTESIAN_POINT('Ctrl Pts',(-31.6136962443577,34.0300695623378,7.84299987264775));
#28477=CARTESIAN_POINT('Ctrl Pts',(-31.2967065907312,35.1352554715487,7.89533324843183));
#28478=CARTESIAN_POINT('Ctrl Pts',(-31.5748397248436,36.4067215963625,7.94766662421592));
#28479=CARTESIAN_POINT('Ctrl Pts',(-32.3264680662287,37.2858331630075,8.));
#28480=CARTESIAN_POINT('',(-37.6785007864356,37.2890249916441,8.));
#28481=CARTESIAN_POINT('Origin',(-35.,35.,8.));
#28482=CARTESIAN_POINT('Ctrl Pts',(-37.6785239274887,37.2890398567007,8.));
#28483=CARTESIAN_POINT('Ctrl Pts',(-36.9607510630042,38.1233253004298,7.95000212253756));
#28484=CARTESIAN_POINT('Ctrl Pts',(-35.8186698457281,38.5989197552422,7.90000424507511));
#28485=CARTESIAN_POINT('Ctrl Pts',(-34.7217022012346,38.5118537728532,7.85000636761267));
#28486=CARTESIAN_POINT('Ctrl Pts',(-33.5734930596489,38.4207207687012,7.79767299182859));
#28487=CARTESIAN_POINT('Ctrl Pts',(-32.4747106147993,37.7131336670436,7.7453396160445));
#28488=CARTESIAN_POINT('Ctrl Pts',(-31.9173295125726,36.7055536114064,7.69300624026042));
#28489=CARTESIAN_POINT('Ctrl Pts',(-31.3599484103458,35.6979735557692,7.64067286447633));
#28490=CARTESIAN_POINT('Ctrl Pts',(-31.3439686507417,34.3904005461523,7.58833948869225));
#28491=CARTESIAN_POINT('Ctrl Pts',(-31.8768870047646,33.3694814192899,7.53600611290817));
#28492=CARTESIAN_POINT('Ctrl Pts',(-32.4098053587874,32.3485622924274,7.48367273712408));
#28493=CARTESIAN_POINT('Ctrl Pts',(-33.4916218264372,31.6142970483194,7.43133936134));
#28494=CARTESIAN_POINT('Ctrl Pts',(-34.6371339251584,31.4957034085517,7.37900598555591));
#28495=CARTESIAN_POINT('Ctrl Pts',(-35.7826460238797,31.3771097687841,7.32667260977183));
#28496=CARTESIAN_POINT('Ctrl Pts',(-36.9918537536724,31.8741877333568,7.27433923398774));
#28497=CARTESIAN_POINT('Ctrl Pts',(-37.7226848809369,32.7641661288242,7.22200585820366));
#28498=CARTESIAN_POINT('Ctrl Pts',(-38.232043765465,33.3844440368906,7.18553167296644));
#28499=CARTESIAN_POINT('Ctrl Pts',(-38.5090307393652,34.1955737201714,7.14905748772921));
#28500=CARTESIAN_POINT('Ctrl Pts',(-38.5153120432796,35.002811202661,7.11258330249199));
#28501=CARTESIAN_POINT('Origin',(-35.,-35.,4.));
#28502=CARTESIAN_POINT('',(-38.5120271382808,-35.0001374244476,0.387416697508025));
#28503=CARTESIAN_POINT('',(-38.5151976130935,-35.0046525930694,0.112583302491978));
#28504=CARTESIAN_POINT('',(-38.5175,-35.,4.));
#28505=CARTESIAN_POINT('',(-37.6735319337713,-32.7141668369925,0.));
#28506=CARTESIAN_POINT('Ctrl Pts',(-38.5151976130935,-35.0046525930694,
0.112583302491978));
#28507=CARTESIAN_POINT('Ctrl Pts',(-38.5080219923978,-34.1767290340604,
0.075055534994651));
#28508=CARTESIAN_POINT('Ctrl Pts',(-38.2125174896864,-33.3445694048179,
0.0375277674973242));
#28509=CARTESIAN_POINT('Ctrl Pts',(-37.6735319337713,-32.7141668369925,
-2.28983498828939E-15));
#28510=CARTESIAN_POINT('',(-32.3214990837181,-32.7109751024398,8.09549783939668E-17));
#28511=CARTESIAN_POINT('Origin',(-35.,-35.,0.));
#28512=CARTESIAN_POINT('Ctrl Pts',(-32.3214759334524,-32.7109602322923,
3.12480707463443E-17));
#28513=CARTESIAN_POINT('Ctrl Pts',(-33.0392487617403,-31.8766749582113,
0.0499978774624439));
#28514=CARTESIAN_POINT('Ctrl Pts',(-34.1813300785248,-31.4010800346315,
0.099995754924887));
#28515=CARTESIAN_POINT('Ctrl Pts',(-35.2782977997678,-31.4881459202074,
0.149993632387331));
#28516=CARTESIAN_POINT('Ctrl Pts',(-36.4265070216881,-31.5792788230239,
0.202327008171415));
#28517=CARTESIAN_POINT('Ctrl Pts',(-37.5252895219377,-32.2868662308611,
0.254660383955499));
#28518=CARTESIAN_POINT('Ctrl Pts',(-38.0826706431354,-33.2944463926721,
0.306993759739583));
#28519=CARTESIAN_POINT('Ctrl Pts',(-38.3681877823846,-33.8105769080839,
0.333801405662397));
#28520=CARTESIAN_POINT('Ctrl Pts',(-38.5116424994856,-34.4054248019609,
0.360609051585211));
#28521=CARTESIAN_POINT('Ctrl Pts',(-38.5120271382808,-35.0001374244476,
0.387416697508025));
#28522=CARTESIAN_POINT('Origin',(-35.,-35.,4.));
#28523=CARTESIAN_POINT('',(-38.5212304296149,-35.0021519659852,1.38741669750803));
#28524=CARTESIAN_POINT('',(-38.5220168341852,-34.9983176676613,1.11258330249198));
#28525=CARTESIAN_POINT('',(-38.5175,-35.,4.));
#28526=CARTESIAN_POINT('Ctrl Pts',(-38.5220168341852,-34.9983176676613,
1.11258330249198));
#28527=CARTESIAN_POINT('Ctrl Pts',(-38.52260684792,-34.8986110126186,1.10805583214991));
#28528=CARTESIAN_POINT('Ctrl Pts',(-38.5187311767415,-34.7989511930367,
1.10352836180784));
#28529=CARTESIAN_POINT('Ctrl Pts',(-38.5102392653976,-34.699686678491,1.09900089146577));
#28530=CARTESIAN_POINT('Ctrl Pts',(-38.4120806130139,-33.5522805666331,
1.04666751568169));
#28531=CARTESIAN_POINT('Ctrl Pts',(-37.6971357336766,-32.4576920494149,
0.994334139897603));
#28532=CARTESIAN_POINT('Ctrl Pts',(-36.6859405355102,-31.906559687218,0.942000764113519));
#28533=CARTESIAN_POINT('Ctrl Pts',(-35.6747453373438,-31.355427325021,0.889667388329434));
#28534=CARTESIAN_POINT('Ctrl Pts',(-34.3672998203483,-31.3477511178455,
0.83733401254535));
#28535=CARTESIAN_POINT('Ctrl Pts',(-33.3498297550083,-31.8872254772169,
0.785000636761265));
#28536=CARTESIAN_POINT('Ctrl Pts',(-32.3323596896683,-32.4266998365882,
0.732667260977181));
#28537=CARTESIAN_POINT('Ctrl Pts',(-31.6048650759839,-33.5133247625066,
0.680333885193095));
#28538=CARTESIAN_POINT('Ctrl Pts',(-31.4934686932928,-34.6593973938948,
0.628000509409011));
#28539=CARTESIAN_POINT('Ctrl Pts',(-31.3820723106017,-35.8054700252831,
0.575667133624927));
#28540=CARTESIAN_POINT('Ctrl Pts',(-31.8867741589039,-37.0109903621411,
0.523333757840844));
#28541=CARTESIAN_POINT('Ctrl Pts',(-32.7813942262272,-37.7364865047087,
0.47100038205676));
#28542=CARTESIAN_POINT('Ctrl Pts',(-33.6760142935505,-38.4619826472763,
0.418667006272675));
#28543=CARTESIAN_POINT('Ctrl Pts',(-34.9605525798949,-38.7074545955534,
0.366333630488589));
#28544=CARTESIAN_POINT('Ctrl Pts',(-36.0588770784695,-38.3607385484851,
0.314000254704505));
#28545=CARTESIAN_POINT('Ctrl Pts',(-37.157201577044,-38.0140225014167,0.26166687892042));
#28546=CARTESIAN_POINT('Ctrl Pts',(-38.0693122878488,-37.0751184590028,
0.209333503136336));
#28547=CARTESIAN_POINT('Ctrl Pts',(-38.3863019623769,-35.9699324345579,
0.157000127352251));
#28548=CARTESIAN_POINT('Ctrl Pts',(-38.4759813473142,-35.6572648277626,
0.142194519065493));
#28549=CARTESIAN_POINT('Ctrl Pts',(-38.518028568312,-35.3312883810079,0.127388910778735));
#28550=CARTESIAN_POINT('Ctrl Pts',(-38.5151976130935,-35.0046525930694,
0.112583302491978));
#28551=CARTESIAN_POINT('Ctrl Pts',(-38.5120271382808,-35.0001374244476,
0.387416697508025));
#28552=CARTESIAN_POINT('Ctrl Pts',(-38.5123933840156,-35.5664114565052,
0.412942427369296));
#28553=CARTESIAN_POINT('Ctrl Pts',(-38.3830453480461,-36.1325628449505,
0.438468157230567));
#28554=CARTESIAN_POINT('Ctrl Pts',(-38.1231131273625,-36.6305186098067,
0.463993887091838));
#28555=CARTESIAN_POINT('Ctrl Pts',(-37.5901947482463,-37.6514377493457,
0.516327262875923));
#28556=CARTESIAN_POINT('Ctrl Pts',(-36.5083782478681,-38.3857031126391,
0.568660638660007));
#28557=CARTESIAN_POINT('Ctrl Pts',(-35.362866098922,-38.5042967770896,0.620994014444091));
#28558=CARTESIAN_POINT('Ctrl Pts',(-34.2173539499758,-38.6228904415402,
0.673327390228176));
#28559=CARTESIAN_POINT('Ctrl Pts',(-33.0081461524618,-38.1258124071479,
0.72566076601226));
#28560=CARTESIAN_POINT('Ctrl Pts',(-32.2773149895643,-37.2358339601687,
0.777994141796345));
#28561=CARTESIAN_POINT('Ctrl Pts',(-31.5464838266669,-36.3458555131895,
0.83032751758043));
#28562=CARTESIAN_POINT('Ctrl Pts',(-31.294029298386,-35.0629766536234,0.882660893364515));
#28563=CARTESIAN_POINT('Ctrl Pts',(-31.6331812255463,-33.9624299433603,
0.934994269148599));
#28564=CARTESIAN_POINT('Ctrl Pts',(-31.9723331527066,-32.8618832330971,
0.987327644932684));
#28565=CARTESIAN_POINT('Ctrl Pts',(-32.9030915353081,-31.9436686721369,
1.03966102071677));
#28566=CARTESIAN_POINT('Ctrl Pts',(-34.0081262229406,-31.6194484991129,
1.09199439650085));
#28567=CARTESIAN_POINT('Ctrl Pts',(-35.1131609105731,-31.2952283260889,
1.14432777228494));
#28568=CARTESIAN_POINT('Ctrl Pts',(-36.3924719032364,-31.5650025410011,
1.19666114806902));
#28569=CARTESIAN_POINT('Ctrl Pts',(-37.2724839907223,-32.3078283275476,
1.24899452385311));
#28570=CARTESIAN_POINT('Ctrl Pts',(-38.0483635269158,-32.9627549301865,
1.29513524840475));
#28571=CARTESIAN_POINT('Ctrl Pts',(-38.5138518348506,-33.9854036989656,
1.34127597295639));
#28572=CARTESIAN_POINT('Ctrl Pts',(-38.5212304296149,-35.0021519659852,
1.38741669750803));
#28573=CARTESIAN_POINT('Origin',(-35.,-35.,4.));
#28574=CARTESIAN_POINT('',(-38.5169621951111,-34.9969726963287,2.38741669750803));
#28575=CARTESIAN_POINT('',(-38.5122617995812,-34.9992080290324,2.11258330249198));
#28576=CARTESIAN_POINT('',(-38.5175,-35.,4.));
#28577=CARTESIAN_POINT('Ctrl Pts',(-38.5122617995812,-34.9992080290324,
2.11258330249198));
#28578=CARTESIAN_POINT('Ctrl Pts',(-38.5133509957446,-34.4699799892041,
2.08872275352108));
#28579=CARTESIAN_POINT('Ctrl Pts',(-38.4009678500058,-33.9411911577145,
2.06486220455019));
#28580=CARTESIAN_POINT('Ctrl Pts',(-38.1726980103725,-33.4683479591114,
2.04100165557929));
#28581=CARTESIAN_POINT('Ctrl Pts',(-37.6720334484517,-32.4312603032644,
1.98866827979521));
#28582=CARTESIAN_POINT('Ctrl Pts',(-36.613887707127,-31.6633030916115,1.93633490401112));
#28583=CARTESIAN_POINT('Ctrl Pts',(-35.4726853098873,-31.5087917472057,
1.88400152822704));
#28584=CARTESIAN_POINT('Ctrl Pts',(-34.3314829126475,-31.3542804028,1.83166815244296));
#28585=CARTESIAN_POINT('Ctrl Pts',(-33.1072238594927,-31.8132149256414,
1.77933477665887));
#28586=CARTESIAN_POINT('Ctrl Pts',(-32.3488109629184,-32.6798336014156,
1.72700140087479));
#28587=CARTESIAN_POINT('Ctrl Pts',(-31.5903980663441,-33.5464522771898,
1.6746680250907));
#28588=CARTESIAN_POINT('Ctrl Pts',(-31.2978313263503,-34.8207551058968,
1.62233464930662));
#28589=CARTESIAN_POINT('Ctrl Pts',(-31.602283651433,-35.931394685751,1.57000127352253));
#28590=CARTESIAN_POINT('Ctrl Pts',(-31.9067359765157,-37.0420342656052,
1.51766789773845));
#28591=CARTESIAN_POINT('Ctrl Pts',(-32.808207366675,-37.9890105966065,1.46533452195436));
#28592=CARTESIAN_POINT('Ctrl Pts',(-33.9025203970559,-38.3477576413965,
1.41300114617028));
#28593=CARTESIAN_POINT('Ctrl Pts',(-34.9968334274368,-38.7065046861866,
1.36066777038619));
#28594=CARTESIAN_POINT('Ctrl Pts',(-36.2839880980393,-38.4770224447653,
1.30833439460211));
#28595=CARTESIAN_POINT('Ctrl Pts',(-37.1868792206255,-37.7621694708059,
1.25600101881803));
#28596=CARTESIAN_POINT('Ctrl Pts',(-38.0116593343501,-37.1091599302205,
1.20819511337601));
#28597=CARTESIAN_POINT('Ctrl Pts',(-38.515786834056,-36.0511278602802,1.16038920793399));
#28598=CARTESIAN_POINT('Ctrl Pts',(-38.5220168341852,-34.9983176676613,
1.11258330249198));
#28599=CARTESIAN_POINT('Ctrl Pts',(-38.5212304296149,-35.0021519659852,
1.38741669750803));
#28600=CARTESIAN_POINT('Ctrl Pts',(-38.5222207275437,-35.1386120556355,
1.39360934874047));
#28601=CARTESIAN_POINT('Ctrl Pts',(-38.5149591261082,-35.2749658599455,
1.39980199997291));
#28602=CARTESIAN_POINT('Ctrl Pts',(-38.4990885075235,-35.4103101250027,
1.40599465120536));
#28603=CARTESIAN_POINT('Ctrl Pts',(-38.3649677545306,-36.5540887777307,
1.45832802698944));
#28604=CARTESIAN_POINT('Ctrl Pts',(-37.6160130662365,-37.6257687250057,
1.51066140277353));
#28605=CARTESIAN_POINT('Ctrl Pts',(-36.5880243363171,-38.1448600164999,
1.56299477855761));
#28606=CARTESIAN_POINT('Ctrl Pts',(-35.5600356063977,-38.6639513079941,
1.6153281543417));
#28607=CARTESIAN_POINT('Ctrl Pts',(-34.2530128348529,-38.6304539437074,
1.66766153012578));
#28608=CARTESIAN_POINT('Ctrl Pts',(-33.2529647263785,-38.059385190685,1.71999490590987));
#28609=CARTESIAN_POINT('Ctrl Pts',(-32.2529166179041,-37.4883164376626,
1.77232828169395));
#28610=CARTESIAN_POINT('Ctrl Pts',(-31.5598431725,-36.3796762959045,1.82466165747803));
#28611=CARTESIAN_POINT('Ctrl Pts',(-31.4844878017471,-35.2305296041615,
1.87699503326212));
#28612=CARTESIAN_POINT('Ctrl Pts',(-31.4091324309942,-34.0813829124186,
1.9293284090462));
#28613=CARTESIAN_POINT('Ctrl Pts',(-31.9514951348924,-32.8917296706907,
1.98166178483029));
#28614=CARTESIAN_POINT('Ctrl Pts',(-32.8684046918336,-32.1949562623368,
2.03399516061437));
#28615=CARTESIAN_POINT('Ctrl Pts',(-33.7853142487749,-31.4981828539828,
2.08632853639846));
#28616=CARTESIAN_POINT('Ctrl Pts',(-35.0767706587592,-31.2942892790027,
2.13866191218254));
#28617=CARTESIAN_POINT('Ctrl Pts',(-36.1637433953085,-31.6746923755375,
2.19099528796663));
#28618=CARTESIAN_POINT('Ctrl Pts',(-37.2507161318578,-32.0550954720723,
2.24332866375071));
#28619=CARTESIAN_POINT('Ctrl Pts',(-38.1332051949721,-33.019795240122,2.29566203953479));
#28620=CARTESIAN_POINT('Ctrl Pts',(-38.4155423057474,-34.1362638239756,
2.34799541531888));
#28621=CARTESIAN_POINT('Ctrl Pts',(-38.4864345470726,-34.416598775556,2.36113584271526));
#28622=CARTESIAN_POINT('Ctrl Pts',(-38.519489264757,-34.7065022308021,2.37427627011164));
#28623=CARTESIAN_POINT('Ctrl Pts',(-38.5169621951111,-34.9969726963287,
2.38741669750803));
#28624=CARTESIAN_POINT('Origin',(-35.,-35.,4.));
#28625=CARTESIAN_POINT('',(-38.5133646692972,-35.0020090495363,3.38741669750803));
#28626=CARTESIAN_POINT('',(-38.5195236027652,-35.0027703381826,3.11258330249198));
#28627=CARTESIAN_POINT('',(-38.5175,-35.,4.));
#28628=CARTESIAN_POINT('Ctrl Pts',(-38.5195236027652,-35.0027703381826,
3.11258330249198));
#28629=CARTESIAN_POINT('Ctrl Pts',(-38.5112998170852,-34.0497594617567,
3.06938967489226));
#28630=CARTESIAN_POINT('Ctrl Pts',(-38.1096194803006,-33.0906361399806,
3.02619604729253));
#28631=CARTESIAN_POINT('Ctrl Pts',(-37.4184570108864,-32.4381577473637,
2.98300241969281));
#28632=CARTESIAN_POINT('Ctrl Pts',(-36.5810449376309,-31.6476152805848,
2.93066904390873));
#28633=CARTESIAN_POINT('Ctrl Pts',(-35.3186808383768,-31.3072193659425,
2.87833566812464));
#28634=CARTESIAN_POINT('Ctrl Pts',(-34.1973517093896,-31.5695881165025,
2.82600229234056));
#28635=CARTESIAN_POINT('Ctrl Pts',(-33.0760225804023,-31.8319568670625,
2.77366891655648));
#28636=CARTESIAN_POINT('Ctrl Pts',(-32.0957284216819,-32.6970902828246,
2.72133554077239));
#28637=CARTESIAN_POINT('Ctrl Pts',(-31.6959888274348,-33.7771017035233,
2.66900216498831));
#28638=CARTESIAN_POINT('Ctrl Pts',(-31.2962492331877,-34.8571131242219,
2.61666878920422));
#28639=CARTESIAN_POINT('Ctrl Pts',(-31.477064203414,-36.1520025498569,2.56433541342014));
#28640=CARTESIAN_POINT('Ctrl Pts',(-32.1573644670244,-37.0811999812203,
2.51200203763605));
#28641=CARTESIAN_POINT('Ctrl Pts',(-32.8376647306348,-38.0103974125836,
2.45966866185197));
#28642=CARTESIAN_POINT('Ctrl Pts',(-34.0174502876292,-38.5739028496752,
2.40733528606788));
#28643=CARTESIAN_POINT('Ctrl Pts',(-35.1677586482437,-38.5190661562666,
2.3550019102838));
#28644=CARTESIAN_POINT('Ctrl Pts',(-36.3180670088582,-38.4642294628581,
2.30266853449971));
#28645=CARTESIAN_POINT('Ctrl Pts',(-37.4388981730927,-37.7910506389493,
2.25033515871563));
#28646=CARTESIAN_POINT('Ctrl Pts',(-38.0277220639514,-36.8013521769744,
2.19800178293155));
#28647=CARTESIAN_POINT('Ctrl Pts',(-38.3480813072967,-36.2628905837198,
2.16952895611836));
#28648=CARTESIAN_POINT('Ctrl Pts',(-38.5109620602598,-35.6307365970085,
2.14105612930517));
#28649=CARTESIAN_POINT('Ctrl Pts',(-38.5122617995812,-34.9992080290324,
2.11258330249198));
#28650=CARTESIAN_POINT('Ctrl Pts',(-38.5169621951111,-34.9969726963287,
2.38741669750803));
#28651=CARTESIAN_POINT('Ctrl Pts',(-38.5094248976387,-35.8633367513267,
2.42660964589573));
#28652=CARTESIAN_POINT('Ctrl Pts',(-38.1853504786061,-36.7347449543441,
2.46580259428343));
#28653=CARTESIAN_POINT('Ctrl Pts',(-37.6045916266667,-37.3723557446642,
2.50499554267113));
#28654=CARTESIAN_POINT('Ctrl Pts',(-36.8291186783745,-38.2237416818415,
2.55732891845522));
#28655=CARTESIAN_POINT('Ctrl Pts',(-35.5959876233539,-38.6582761565386,
2.6096622942393));
#28656=CARTESIAN_POINT('Ctrl Pts',(-34.4580786668646,-38.4811335311572,
2.66199567002338));
#28657=CARTESIAN_POINT('Ctrl Pts',(-33.3201697103753,-38.3039909057758,
2.71432904580747));
#28658=CARTESIAN_POINT('Ctrl Pts',(-32.2774828524173,-37.5151711803159,
2.76666242159156));
#28659=CARTESIAN_POINT('Ctrl Pts',(-31.7975117563928,-36.4683454731577,
2.81899579737564));
#28660=CARTESIAN_POINT('Ctrl Pts',(-31.3175406603683,-35.4215197659996,
2.87132917315973));
#28661=CARTESIAN_POINT('Ctrl Pts',(-31.4002853262773,-34.1166880771431,
2.92366254894381));
#28662=CARTESIAN_POINT('Ctrl Pts',(-32.008646781737,-33.138877947982,2.97599592472789));
#28663=CARTESIAN_POINT('Ctrl Pts',(-32.6170082371967,-32.1610678188208,
3.02832930051198));
#28664=CARTESIAN_POINT('Ctrl Pts',(-33.7509864822071,-31.5102792493549,
3.08066267629606));
#28665=CARTESIAN_POINT('Ctrl Pts',(-34.9021569334111,-31.4782964190287,
3.13299605208015));
#28666=CARTESIAN_POINT('Ctrl Pts',(-36.0533273846151,-31.4463135887025,
3.18532942786423));
#28667=CARTESIAN_POINT('Ctrl Pts',(-37.2216900420126,-32.033136497516,3.23766280364832));
#28668=CARTESIAN_POINT('Ctrl Pts',(-37.883403902666,-32.9756602781289,3.2899961794324));
#28669=CARTESIAN_POINT('Ctrl Pts',(-38.2940055257973,-33.5605079247801,
3.32246968545761));
#28670=CARTESIAN_POINT('Ctrl Pts',(-38.5095293369816,-34.2823130619538,
3.35494319148282));
#28671=CARTESIAN_POINT('Ctrl Pts',(-38.5133646692972,-35.0020090495363,
3.38741669750803));
#28672=CARTESIAN_POINT('Origin',(-35.,-35.,4.));
#28673=CARTESIAN_POINT('',(-38.5230462440028,-35.0002063500719,4.38741669750802));
#28674=CARTESIAN_POINT('',(-38.5188572457002,-34.9970948475072,4.11258330249198));
#28675=CARTESIAN_POINT('',(-38.5175,-35.,4.));
#28676=CARTESIAN_POINT('Ctrl Pts',(-38.5188572457002,-34.9970948475072,
4.11258330249198));
#28677=CARTESIAN_POINT('Ctrl Pts',(-38.5208451479049,-34.772082045238,4.10238997204752));
#28678=CARTESIAN_POINT('Ctrl Pts',(-38.5010645257441,-34.5474171474031,
4.09219664160305));
#28679=CARTESIAN_POINT('Ctrl Pts',(-38.4582307571508,-34.3272370005912,
4.08200331115859));
#28680=CARTESIAN_POINT('Ctrl Pts',(-38.2383187548614,-33.1968144732253,
4.0296699353745));
#28681=CARTESIAN_POINT('Ctrl Pts',(-37.410753954154,-32.1846045081767,3.97733655959042));
#28682=CARTESIAN_POINT('Ctrl Pts',(-36.3465790030625,-31.7444362988739,
3.92500318380633));
#28683=CARTESIAN_POINT('Ctrl Pts',(-35.2824040519711,-31.3042680895711,
3.87266980802225));
#28684=CARTESIAN_POINT('Ctrl Pts',(-33.9816189504956,-31.4361416360142,
3.82033643223816));
#28685=CARTESIAN_POINT('Ctrl Pts',(-33.0274369384391,-32.0809308006472,
3.76800305645408));
#28686=CARTESIAN_POINT('Ctrl Pts',(-32.0732549263827,-32.7257199652802,
3.71566968067));
#28687=CARTESIAN_POINT('Ctrl Pts',(-31.4656760037452,-33.8834247481031,
3.66333630488591));
#28688=CARTESIAN_POINT('Ctrl Pts',(-31.4771110949952,-35.0349826573345,
3.61100292910183));
#28689=CARTESIAN_POINT('Ctrl Pts',(-31.4885461862452,-36.1865405665659,
3.55866955331774));
#28690=CARTESIAN_POINT('Ctrl Pts',(-32.1189952913826,-37.3319516022057,
3.50633617753366));
#28691=CARTESIAN_POINT('Ctrl Pts',(-33.0857935298184,-37.957665230428,3.45400280174958));
#28692=CARTESIAN_POINT('Ctrl Pts',(-34.0525917682542,-38.5833788586504,
3.40166942596549));
#28693=CARTESIAN_POINT('Ctrl Pts',(-35.3557391399884,-38.6893950794552,
3.3493360501814));
#28694=CARTESIAN_POINT('Ctrl Pts',(-36.4109632703443,-38.2281810151433,
3.29700267439732));
#28695=CARTESIAN_POINT('Ctrl Pts',(-37.4661874007003,-37.7669669508313,
3.24466929861323));
#28696=CARTESIAN_POINT('Ctrl Pts',(-38.273488289678,-36.7385226014027,3.19233592282915));
#28697=CARTESIAN_POINT('Ctrl Pts',(-38.4709087105384,-35.6039559172305,
3.14000254704507));
#28698=CARTESIAN_POINT('Ctrl Pts',(-38.5053871462609,-35.4058098271621,
3.1308627988607));
#28699=CARTESIAN_POINT('Ctrl Pts',(-38.5212637513569,-35.2044269229967,
3.12172305067634));
#28700=CARTESIAN_POINT('Ctrl Pts',(-38.5195236027652,-35.0027703381826,
3.11258330249198));
#28701=CARTESIAN_POINT('Ctrl Pts',(-38.5133646692972,-35.0020090495363,
3.38741669750803));
#28702=CARTESIAN_POINT('Ctrl Pts',(-38.5157102491126,-35.4421545813516,
3.4072765672669));
#28703=CARTESIAN_POINT('Ctrl Pts',(-38.4388801758726,-35.8815112497523,
3.42713643702578));
#28704=CARTESIAN_POINT('Ctrl Pts',(-38.2790749297269,-36.2882689858157,
3.44699630678465));
#28705=CARTESIAN_POINT('Ctrl Pts',(-37.8579670322255,-37.3601292604774,
3.49932968256874));
#28706=CARTESIAN_POINT('Ctrl Pts',(-36.8606861733137,-38.2056251573884,
3.55166305835282));
#28707=CARTESIAN_POINT('Ctrl Pts',(-35.7343680095528,-38.4456745351613,
3.60399643413691));
#28708=CARTESIAN_POINT('Ctrl Pts',(-34.6080498457918,-38.6857239129342,
3.65632980992099));
#28709=CARTESIAN_POINT('Ctrl Pts',(-33.3526943771818,-38.3203267715691,
3.70866318570508));
#28710=CARTESIAN_POINT('Ctrl Pts',(-32.5311462498722,-37.5133106723387,
3.76099656148916));
#28711=CARTESIAN_POINT('Ctrl Pts',(-31.7095981225626,-36.7062945731084,
3.81332993727325));
#28712=CARTESIAN_POINT('Ctrl Pts',(-31.3218573365535,-35.4576595160129,
3.86566331305733));
#28713=CARTESIAN_POINT('Ctrl Pts',(-31.5417693331035,-34.3272370181493,
3.91799668884141));
#28714=CARTESIAN_POINT('Ctrl Pts',(-31.7616813296536,-33.1968145202857,
3.9703300646255));
#28715=CARTESIAN_POINT('Ctrl Pts',(-32.5892461087628,-32.184604581654,4.02266344040958));
#28716=CARTESIAN_POINT('Ctrl Pts',(-33.653421032081,-31.7444363838389,4.07499681619367));
#28717=CARTESIAN_POINT('Ctrl Pts',(-34.7175959553992,-31.3042681860239,
4.12733019197775));
#28718=CARTESIAN_POINT('Ctrl Pts',(-36.0183810229263,-31.4361417290255,
4.17966356776184));
#28719=CARTESIAN_POINT('Ctrl Pts',(-36.9725630100801,-32.0809308768304,
4.23199694354592));
#28720=CARTESIAN_POINT('Ctrl Pts',(-37.9171401399176,-32.7192295355597,
4.28380352819995));
#28721=CARTESIAN_POINT('Ctrl Pts',(-38.5220569274439,-33.8601696875978,
4.33561011285399));
#28722=CARTESIAN_POINT('Ctrl Pts',(-38.5230462440028,-35.0002063500719,
4.38741669750802));
#28723=CARTESIAN_POINT('Origin',(-35.,-35.,4.));
#28724=CARTESIAN_POINT('',(-38.5138068989996,-34.9977297535637,5.38741669750802));
#28725=CARTESIAN_POINT('',(-38.5124574312326,-35.001138833141,5.11258330249198));
#28726=CARTESIAN_POINT('',(-38.5175,-35.,4.));
#28727=CARTESIAN_POINT('Ctrl Pts',(-38.5124574312326,-35.001138833141,5.11258330249198));
#28728=CARTESIAN_POINT('Ctrl Pts',(-38.5105122060607,-34.3463332977053,
5.08305689341869));
#28729=CARTESIAN_POINT('Ctrl Pts',(-38.3345898905329,-33.6905568650893,
5.0535304843454));
#28730=CARTESIAN_POINT('Ctrl Pts',(-37.9913532963331,-33.1388778994087,
5.02400407527211));
#28731=CARTESIAN_POINT('Ctrl Pts',(-37.3829918249966,-32.1610677447274,
4.97167069948802));
#28732=CARTESIAN_POINT('Ctrl Pts',(-36.2490135503901,-31.5102791582787,
4.91933732370394));
#28733=CARTESIAN_POINT('Ctrl Pts',(-35.0978430691422,-31.4782963271182,
4.86700394791986));
#28734=CARTESIAN_POINT('Ctrl Pts',(-33.9466725878942,-31.4463134959578,
4.81467057213577));
#28735=CARTESIAN_POINT('Ctrl Pts',(-32.7783099000047,-32.0331364200855,
4.76233719635169));
#28736=CARTESIAN_POINT('Ctrl Pts',(-32.1165960220819,-32.9756602252966,
4.7100038205676));
#28737=CARTESIAN_POINT('Ctrl Pts',(-31.454882144159,-33.9181840305077,4.65767044478352));
#28738=CARTESIAN_POINT('Ctrl Pts',(-31.2998170762027,-35.216408716802,4.60533706899943));
#28739=CARTESIAN_POINT('Ctrl Pts',(-31.7209249846943,-36.2882690194377,
4.55300369321535));
#28740=CARTESIAN_POINT('Ctrl Pts',(-32.1420328931859,-37.3601293220733,
4.50067031743126));
#28741=CARTESIAN_POINT('Ctrl Pts',(-33.1393137781253,-38.2056252410501,
4.44833694164718));
#28742=CARTESIAN_POINT('Ctrl Pts',(-34.2656319712814,-38.4456746250879,
4.39600356586309));
#28743=CARTESIAN_POINT('Ctrl Pts',(-35.3919501644375,-38.6857240091257,
4.34367019007901));
#28744=CARTESIAN_POINT('Ctrl Pts',(-36.6473056658103,-38.3203268582244,
4.29133681429492));
#28745=CARTESIAN_POINT('Ctrl Pts',(-37.468853814561,-37.5133107379322,4.23900343851084));
#28746=CARTESIAN_POINT('Ctrl Pts',(-38.1303833971331,-36.8634826809916,
4.19686339317122));
#28747=CARTESIAN_POINT('Ctrl Pts',(-38.5106390985996,-35.9273158131948,
4.1547233478316));
#28748=CARTESIAN_POINT('Ctrl Pts',(-38.5188572457002,-34.9970948475072,
4.11258330249198));
#28749=CARTESIAN_POINT('Ctrl Pts',(-38.5230462440028,-35.0002063500719,
4.38741669750802));
#28750=CARTESIAN_POINT('Ctrl Pts',(-38.5230563037894,-35.0117987220789,
4.38794348863807));
#28751=CARTESIAN_POINT('Ctrl Pts',(-38.5230039194247,-35.023391000668,4.38847027976812));
#28752=CARTESIAN_POINT('Ctrl Pts',(-38.5228888130629,-35.0349826564212,
4.38899707089817));
#28753=CARTESIAN_POINT('Ctrl Pts',(-38.5114537221114,-36.186540535599,4.44133044668226));
#28754=CARTESIAN_POINT('Ctrl Pts',(-37.8810046334278,-37.3319515413465,
4.49366382246634));
#28755=CARTESIAN_POINT('Ctrl Pts',(-36.9142064202239,-37.9576651532382,
4.54599719825043));
#28756=CARTESIAN_POINT('Ctrl Pts',(-35.94740820702,-38.5833787651299,4.59833057403451));
#28757=CARTESIAN_POINT('Ctrl Pts',(-34.6442608692957,-38.6893949831658,
4.6506639498186));
#28758=CARTESIAN_POINT('Ctrl Pts',(-33.5890367664795,-38.2281809308918,
4.70299732560268));
#28759=CARTESIAN_POINT('Ctrl Pts',(-32.5338126636633,-37.7669668786178,
4.75533070138677));
#28760=CARTESIAN_POINT('Ctrl Pts',(-31.7265117957552,-36.7385225560339,
4.80766407717085));
#28761=CARTESIAN_POINT('Ctrl Pts',(-31.529091380047,-35.6039559014703,4.85999745295494));
#28762=CARTESIAN_POINT('Ctrl Pts',(-31.3316709643388,-34.4693892469067,
4.91233082873902));
#28763=CARTESIAN_POINT('Ctrl Pts',(-31.7441310008306,-33.2287002603633,
4.9646642045231));
#28764=CARTESIAN_POINT('Ctrl Pts',(-32.5815430522312,-32.4381578142198,
5.01699758030719));
#28765=CARTESIAN_POINT('Ctrl Pts',(-33.4189551036319,-31.6476153680763,
5.06933095609127));
#28766=CARTESIAN_POINT('Ctrl Pts',(-34.6813191699414,-31.3072194623328,
5.12166433187536));
#28767=CARTESIAN_POINT('Ctrl Pts',(-35.8026482696631,-31.5695882060385,
5.17399770765944));
#28768=CARTESIAN_POINT('Ctrl Pts',(-36.9239773693848,-31.8319569497442,
5.22633108344353));
#28769=CARTESIAN_POINT('Ctrl Pts',(-37.9042715025186,-32.6970903428993,
5.27866445922761));
#28770=CARTESIAN_POINT('Ctrl Pts',(-38.3040110863345,-33.7771017354242,
5.33099783501169));
#28771=CARTESIAN_POINT('Ctrl Pts',(-38.4476597125745,-34.1652097916211,
5.34980412251047));
#28772=CARTESIAN_POINT('Ctrl Pts',(-38.5163376200166,-34.5810664169843,
5.36861041000925));
#28773=CARTESIAN_POINT('Ctrl Pts',(-38.5138068989996,-34.9977297535637,
5.38741669750802));
#28774=CARTESIAN_POINT('Origin',(-35.,-35.,4.));
#28775=CARTESIAN_POINT('',(-38.5163032009778,-35.0029832534533,6.38741669750803));
#28776=CARTESIAN_POINT('',(-38.522424122767,-35.0013091826171,6.11258330249198));
#28777=CARTESIAN_POINT('',(-38.5175,-35.,4.));
#28778=CARTESIAN_POINT('Ctrl Pts',(-38.522424122767,-35.0013091826171,6.11258330249198));
#28779=CARTESIAN_POINT('Ctrl Pts',(-38.5172132511134,-33.9256163607463,
6.06372381478986));
#28780=CARTESIAN_POINT('Ctrl Pts',(-37.9876405112709,-32.8454778142804,
6.01486432708775));
#28781=CARTESIAN_POINT('Ctrl Pts',(-37.1315953638235,-32.1949561890823,
5.96600483938563));
#28782=CARTESIAN_POINT('Ctrl Pts',(-36.2146857829733,-31.4981827625019,
5.91367146360154));
#28783=CARTESIAN_POINT('Ctrl Pts',(-34.9232293392347,-31.2942891822923,
5.86133808781746));
#28784=CARTESIAN_POINT('Ctrl Pts',(-33.8362565743057,-31.6746922887769,
5.80900471203338));
#28785=CARTESIAN_POINT('Ctrl Pts',(-32.7492838093767,-32.0550953952615,
5.75667133624929));
#28786=CARTESIAN_POINT('Ctrl Pts',(-31.8667947232573,-33.0197951884404,
5.7043379604652));
#28787=CARTESIAN_POINT('Ctrl Pts',(-31.5844576051196,-34.1362638014206,
5.65200458468112));
#28788=CARTESIAN_POINT('Ctrl Pts',(-31.302120486982,-35.2527324144008,5.59967120889704));
#28789=CARTESIAN_POINT('Ctrl Pts',(-31.6199353368261,-36.5209698471824,
5.54733783311296));
#28790=CARTESIAN_POINT('Ctrl Pts',(-32.3954083053537,-37.3723558065856,
5.49500445732887));
#28791=CARTESIAN_POINT('Ctrl Pts',(-33.1708812738812,-38.2237417659887,
5.44267108154479));
#28792=CARTESIAN_POINT('Ctrl Pts',(-34.4040123610921,-38.6582762520135,
5.3903377057607));
#28793=CARTESIAN_POINT('Ctrl Pts',(-35.5419213472807,-38.4811336220058,
5.33800432997661));
#28794=CARTESIAN_POINT('Ctrl Pts',(-36.6798303334694,-38.3039909919981,
5.28567095419253));
#28795=CARTESIAN_POINT('Ctrl Pts',(-37.722517218636,-37.515171245958,5.23333757840845));
#28796=CARTESIAN_POINT('Ctrl Pts',(-38.202488327186,-36.468345511481,5.18100420262436));
#28797=CARTESIAN_POINT('Ctrl Pts',(-38.4116604841668,-36.0121372252676,
5.15819723591357));
#28798=CARTESIAN_POINT('Ctrl Pts',(-38.5139599737744,-35.5069276682025,
5.13539026920277));
#28799=CARTESIAN_POINT('Ctrl Pts',(-38.5124574312326,-35.001138833141,5.11258330249198));
#28800=CARTESIAN_POINT('Ctrl Pts',(-38.5138068989996,-34.9977297535637,
5.38741669750802));
#28801=CARTESIAN_POINT('Ctrl Pts',(-38.5092952319858,-35.7405402881605,
5.42094378579333));
#28802=CARTESIAN_POINT('Ctrl Pts',(-38.2784660556449,-36.4859147377931,
5.45447087407864));
#28803=CARTESIAN_POINT('Ctrl Pts',(-37.8426354587898,-37.0811999269324,
5.48799796236395));
#28804=CARTESIAN_POINT('Ctrl Pts',(-37.1623352129312,-38.0103973340206,
5.54033133814803));
#28805=CARTESIAN_POINT('Ctrl Pts',(-35.982549686716,-38.5739027563021,5.59266471393212));
#28806=CARTESIAN_POINT('Ctrl Pts',(-34.8322413561292,-38.5190660643709,
5.6449980897162));
#28807=CARTESIAN_POINT('Ctrl Pts',(-33.6819330255423,-38.4642293724398,
5.69733146550029));
#28808=CARTESIAN_POINT('Ctrl Pts',(-32.5611018905839,-37.791050566296,5.74966484128437));
#28809=CARTESIAN_POINT('Ctrl Pts',(-31.9722780150789,-36.8013521300638,
5.80199821706845));
#28810=CARTESIAN_POINT('Ctrl Pts',(-31.3834541395739,-35.8116536938316,
5.85433159285254));
#28811=CARTESIAN_POINT('Ctrl Pts',(-31.3266375235224,-34.5054356275111,
5.90666496863662));
#28812=CARTESIAN_POINT('Ctrl Pts',(-31.8273020724053,-33.4683479988925,
5.95899834442071));
#28813=CARTESIAN_POINT('Ctrl Pts',(-32.3279666212882,-32.431260370274,6.01133172020479));
#28814=CARTESIAN_POINT('Ctrl Pts',(-33.3861123351056,-31.6633031793574,
6.06366509598888));
#28815=CARTESIAN_POINT('Ctrl Pts',(-34.5273147025013,-31.5087918386834,
6.11599847177296));
#28816=CARTESIAN_POINT('Ctrl Pts',(-35.668517069897,-31.3542804980094,6.16833184755705));
#28817=CARTESIAN_POINT('Ctrl Pts',(-36.892776090871,-31.8132150075779,6.22066522334113));
#28818=CARTESIAN_POINT('Ctrl Pts',(-37.6511889677791,-32.6798336612887,
6.27299859912521));
#28819=CARTESIAN_POINT('Ctrl Pts',(-38.2039029090244,-33.3114054953559,
6.31113796525282));
#28820=CARTESIAN_POINT('Ctrl Pts',(-38.509198477207,-34.1595049296877,6.34927733138042));
#28821=CARTESIAN_POINT('Ctrl Pts',(-38.5163032009778,-35.0029832534533,
6.38741669750803));
#28822=CARTESIAN_POINT('Origin',(-35.,-35.,4.));
#28823=CARTESIAN_POINT('',(-38.5217392653161,-34.9982348400382,7.38741669750802));
#28824=CARTESIAN_POINT('',(-38.5153122961063,-34.9971887940747,7.11258330249198));
#28825=CARTESIAN_POINT('',(-38.5175,-35.,4.));
#28826=CARTESIAN_POINT('',(-32.3264680662287,-32.7141668369925,8.));
#28827=CARTESIAN_POINT('Ctrl Pts',(-38.5217392653161,-34.9982348400382,
7.38741669750802));
#28828=CARTESIAN_POINT('Ctrl Pts',(-38.5150454835571,-36.0376021634142,
7.43461100431976));
#28829=CARTESIAN_POINT('Ctrl Pts',(-38.0253751592018,-37.0822329702746,
7.48180531113151));
#28830=CARTESIAN_POINT('Ctrl Pts',(-37.2186056743939,-37.7364863611315,
7.52899961794325));
#28831=CARTESIAN_POINT('Ctrl Pts',(-36.3239856773675,-38.4619825252834,
7.58133299372733));
#28832=CARTESIAN_POINT('Ctrl Pts',(-35.0394476042314,-38.7074546780583,
7.63366636951141));
#28833=CARTESIAN_POINT('Ctrl Pts',(-33.9411230034093,-38.3607385339716,
7.68599974529549));
#28834=CARTESIAN_POINT('Ctrl Pts',(-32.8427984025871,-38.0140223898848,
7.73833312107958));
#28835=CARTESIAN_POINT('Ctrl Pts',(-31.9306872740789,-37.0751179489365,
7.79066649686366));
#28836=CARTESIAN_POINT('Ctrl Pts',(-31.613697604643,-35.9699319523746,7.84299987264775));
#28837=CARTESIAN_POINT('Ctrl Pts',(-31.2967079352071,-34.8647459558128,
7.89533324843184));
#28838=CARTESIAN_POINT('Ctrl Pts',(-31.5748397248436,-33.5932784036375,
7.94766662421592));
#28839=CARTESIAN_POINT('Ctrl Pts',(-32.3264680662287,-32.7141668369925,
8.));
#28840=CARTESIAN_POINT('',(-37.6785009901498,-32.7109751557132,8.));
#28841=CARTESIAN_POINT('Origin',(-35.,-35.,8.));
#28842=CARTESIAN_POINT('Ctrl Pts',(-37.6785241456451,-32.7109602826759,
8.));
#28843=CARTESIAN_POINT('Ctrl Pts',(-36.9607513379489,-31.8766751051408,
7.95000212253756));
#28844=CARTESIAN_POINT('Ctrl Pts',(-35.8186699645707,-31.4010799150529,
7.90000424507511));
#28845=CARTESIAN_POINT('Ctrl Pts',(-34.7217021996619,-31.4881457455928,
7.85000636761267));
#28846=CARTESIAN_POINT('Ctrl Pts',(-33.573492932036,-31.5792785908026,7.79767299182859));
#28847=CARTESIAN_POINT('Ctrl Pts',(-32.4747104002448,-32.2868661727234,
7.7453396160445));
#28848=CARTESIAN_POINT('Ctrl Pts',(-31.9173292682424,-33.2944463949298,
7.69300624026042));
#28849=CARTESIAN_POINT('Ctrl Pts',(-31.3599481362399,-34.3020266171361,
7.64067286447633));
#28850=CARTESIAN_POINT('Ctrl Pts',(-31.3439684040262,-35.609599479628,7.58833948869224));
#28851=CARTESIAN_POINT('Ctrl Pts',(-31.8768867974267,-36.6305186264058,
7.53600611290816));
#28852=CARTESIAN_POINT('Ctrl Pts',(-32.4098051908272,-37.6514377731836,
7.48367273712407));
#28853=CARTESIAN_POINT('Ctrl Pts',(-33.491621709842,-38.3857032042473,7.43133936134));
#28854=CARTESIAN_POINT('Ctrl Pts',(-34.6371338873761,-38.5042968827328,
7.37900598555591));
#28855=CARTESIAN_POINT('Ctrl Pts',(-35.7826460649101,-38.6228905612183,
7.32667260977183));
#28856=CARTESIAN_POINT('Ctrl Pts',(-36.9918539009634,-38.1258124871256,
7.27433923398775));
#28857=CARTESIAN_POINT('Ctrl Pts',(-37.7226850841419,-37.2358340108349,
7.22200585820366));
#28858=CARTESIAN_POINT('Ctrl Pts',(-38.2320440076398,-36.615556046438,7.18553167296643));
#28859=CARTESIAN_POINT('Ctrl Pts',(-38.5090309960538,-35.8044263207662,
7.14905748772921));
#28860=CARTESIAN_POINT('Ctrl Pts',(-38.5153122961063,-34.9971887940747,
7.11258330249198));
#28861=CARTESIAN_POINT('Origin',(35.,-35.,4.));
#28862=CARTESIAN_POINT('',(31.4879726191333,-35.0001375015905,0.387416697508024));
#28863=CARTESIAN_POINT('',(31.4847993146864,-35.0046492582639,0.112583302491975));
#28864=CARTESIAN_POINT('',(31.4825,-35.,4.));
#28865=CARTESIAN_POINT('',(32.3264680662287,-32.7141668369925,0.));
#28866=CARTESIAN_POINT('Ctrl Pts',(31.4847993146864,-35.0046492582639,0.112583302491975));
#28867=CARTESIAN_POINT('Ctrl Pts',(31.4919760559448,-34.1767269622227,0.0750555349946493));
#28868=CARTESIAN_POINT('Ctrl Pts',(31.7874825103136,-33.3445694048179,0.037527767497323));
#28869=CARTESIAN_POINT('Ctrl Pts',(32.3264680662287,-32.7141668369925,-2.98372437868011E-15));
#28870=CARTESIAN_POINT('',(37.6785011129036,-32.7109752438421,-5.55678203018928E-16));
#28871=CARTESIAN_POINT('Origin',(35.,-35.,0.));
#28872=CARTESIAN_POINT('Ctrl Pts',(37.6785242770714,-32.7109603660127,-2.86292032689789E-16));
#28873=CARTESIAN_POINT('Ctrl Pts',(36.9607515035944,-31.8766753489742,0.0499978774624439));
#28874=CARTESIAN_POINT('Ctrl Pts',(35.8186700361932,-31.4010797162719,0.099995754924888));
#28875=CARTESIAN_POINT('Ctrl Pts',(34.7217021987141,-31.4881454554173,0.149993632387332));
#28876=CARTESIAN_POINT('Ctrl Pts',(33.5734928551282,-31.5792782049632,0.202327008171416));
#28877=CARTESIAN_POINT('Ctrl Pts',(32.4747102708807,-32.2868660760186,0.2546603839555));
#28878=CARTESIAN_POINT('Ctrl Pts',(31.9173291209027,-33.2944463985812,0.306993759739584));
#28879=CARTESIAN_POINT('Ctrl Pts',(31.6318119669108,-33.8105769963377,0.333801405662397));
#28880=CARTESIAN_POINT('Ctrl Pts',(31.488357249556,-34.4054248931928,0.360609051585211));
#28881=CARTESIAN_POINT('Ctrl Pts',(31.4879726191333,-35.0001375015905,0.387416697508024));
#28882=CARTESIAN_POINT('Origin',(35.,-35.,4.));
#28883=CARTESIAN_POINT('',(31.4787693262007,-35.0021519651487,1.38741669750802));
#28884=CARTESIAN_POINT('',(31.4779839561681,-34.998317589092,1.11258330249197));
#28885=CARTESIAN_POINT('',(31.4825,-35.,4.));
#28886=CARTESIAN_POINT('Ctrl Pts',(31.4779839561681,-34.998317589092,1.11258330249197));
#28887=CARTESIAN_POINT('Ctrl Pts',(31.4773939435915,-34.8986109589584,1.10805583214991));
#28888=CARTESIAN_POINT('Ctrl Pts',(31.4812696152992,-34.7989511654426,1.10352836180784));
#28889=CARTESIAN_POINT('Ctrl Pts',(31.4897615265674,-34.6996866782215,1.09900089146577));
#28890=CARTESIAN_POINT('Ctrl Pts',(31.5879201780762,-33.5522808822113,1.04666751568169));
#28891=CARTESIAN_POINT('Ctrl Pts',(32.3028649757287,-32.457692848996,0.994334139897601));
#28892=CARTESIAN_POINT('Ctrl Pts',(33.314059894657,-31.906560527472,0.942000764113516));
#28893=CARTESIAN_POINT('Ctrl Pts',(34.3252548135852,-31.3554282059481,0.889667388329432));
#28894=CARTESIAN_POINT('Ctrl Pts',(35.6326998537893,-31.3477515961155,0.837334012545348));
#28895=CARTESIAN_POINT('Ctrl Pts',(36.650169778933,-31.8872259747803,0.785000636761264));
#28896=CARTESIAN_POINT('Ctrl Pts',(37.6676397040767,-32.4267003534451,0.732667260977179));
#28897=CARTESIAN_POINT('Ctrl Pts',(38.39513451416,-33.5133257206073,0.680333885193094));
#28898=CARTESIAN_POINT('Ctrl Pts',(38.5065306720619,-34.6593978563341,0.628000509409009));
#28899=CARTESIAN_POINT('Ctrl Pts',(38.6179268299637,-35.8054699920609,0.575667133624925));
#28900=CARTESIAN_POINT('Ctrl Pts',(38.1132243356843,-37.0109888963523,0.523333757840841));
#28901=CARTESIAN_POINT('Ctrl Pts',(37.2186048923566,-37.7364852312874,0.471000382056757));
#28902=CARTESIAN_POINT('Ctrl Pts',(36.3239854490289,-38.4619815662224,0.418667006272672));
#28903=CARTESIAN_POINT('Ctrl Pts',(35.0394490566529,-38.7074553318012,0.366333630488587));
#28904=CARTESIAN_POINT('Ctrl Pts',(33.9411236515154,-38.3607384247595,0.314000254704503));
#28905=CARTESIAN_POINT('Ctrl Pts',(32.842798246378,-38.0140215177178,0.261666878920419));
#28906=CARTESIAN_POINT('Ctrl Pts',(31.930683828479,-37.0751139380558,0.209333503136335));
#28907=CARTESIAN_POINT('Ctrl Pts',(31.6136941980954,-35.9699281595357,0.157000127352251));
#28908=CARTESIAN_POINT('Ctrl Pts',(31.524014825647,-35.6572606223148,0.142194519065492));
#28909=CARTESIAN_POINT('Ctrl Pts',(31.4819679173789,-35.3312845479312,0.127388910778734));
#28910=CARTESIAN_POINT('Ctrl Pts',(31.4847993146864,-35.0046492582639,0.112583302491975));
#28911=CARTESIAN_POINT('Ctrl Pts',(31.4879726191333,-35.0001375015905,0.387416697508024));
#28912=CARTESIAN_POINT('Ctrl Pts',(31.4876063813705,-35.5664115202329,0.412942427369295));
#28913=CARTESIAN_POINT('Ctrl Pts',(31.6169544331328,-36.1325628797889,0.438468157230566));
#28914=CARTESIAN_POINT('Ctrl Pts',(31.8768866723687,-36.6305186540646,0.463993887091838));
#28915=CARTESIAN_POINT('Ctrl Pts',(32.4098050895213,-37.6514378129155,0.516327262875923));
#28916=CARTESIAN_POINT('Ctrl Pts',(33.491621639535,-38.3857033565476,0.568660638660007));
#28917=CARTESIAN_POINT('Ctrl Pts',(34.6371338646016,-38.5042970583454,0.620994014444092));
#28918=CARTESIAN_POINT('Ctrl Pts',(35.7826460896681,-38.6228907601432,0.673327390228177));
#28919=CARTESIAN_POINT('Ctrl Pts',(36.9918539897876,-38.1258126201067,0.725660766012261));
#28920=CARTESIAN_POINT('Ctrl Pts',(37.7226852066847,-37.235834095095,0.777994141796346));
#28921=CARTESIAN_POINT('Ctrl Pts',(38.4535164235819,-36.3458555700833,0.83032751758043));
#28922=CARTESIAN_POINT('Ctrl Pts',(38.7059709572567,-35.0629766600964,0.882660893364514));
#28923=CARTESIAN_POINT('Ctrl Pts',(38.3668190041959,-33.9624298822548,0.934994269148598));
#28924=CARTESIAN_POINT('Ctrl Pts',(38.027667051135,-32.8618831044132,0.987327644932683));
#28925=CARTESIAN_POINT('Ctrl Pts',(37.0969086113384,-31.9436684587171,1.03966102071677));
#28926=CARTESIAN_POINT('Ctrl Pts',(35.9918738484399,-31.6194482583158,1.09199439650085));
#28927=CARTESIAN_POINT('Ctrl Pts',(34.8868390855414,-31.2952280579146,1.14432777228494));
#28928=CARTESIAN_POINT('Ctrl Pts',(33.607527999541,-31.5650023028083,1.19666114806902));
#28929=CARTESIAN_POINT('Ctrl Pts',(32.7275158499642,-32.3078281435934,1.24899452385311));
#28930=CARTESIAN_POINT('Ctrl Pts',(31.9516362590269,-32.9627547940529,1.29513524840474));
#28931=CARTESIAN_POINT('Ctrl Pts',(31.4861479206373,-33.9854036295086,1.34127597295638));
#28932=CARTESIAN_POINT('Ctrl Pts',(31.4787693262007,-35.0021519651487,1.38741669750802));
#28933=CARTESIAN_POINT('Origin',(35.,-35.,4.));
#28934=CARTESIAN_POINT('',(31.4830375605149,-34.9969726960772,2.38741669750802));
#28935=CARTESIAN_POINT('',(31.4877390119671,-34.9992080277921,2.11258330249198));
#28936=CARTESIAN_POINT('',(31.4825,-35.,4.));
#28937=CARTESIAN_POINT('Ctrl Pts',(31.4877390119671,-34.9992080277921,2.11258330249198));
#28938=CARTESIAN_POINT('Ctrl Pts',(31.4866498159747,-34.4699801096587,2.08872275352108));
#28939=CARTESIAN_POINT('Ctrl Pts',(31.5990329357071,-33.9411914000592,2.06486220455019));
#28940=CARTESIAN_POINT('Ctrl Pts',(31.8273027226982,-33.4683483113999,2.04100165557929));
#28941=CARTESIAN_POINT('Ctrl Pts',(32.3279671691587,-32.431260896693,1.98866827979521));
#28942=CARTESIAN_POINT('Ctrl Pts',(33.3861126668897,-31.6633038687123,1.93633490401112));
#28943=CARTESIAN_POINT('Ctrl Pts',(34.5273147998293,-31.5087925573416,1.88400152822704));
#28944=CARTESIAN_POINT('Ctrl Pts',(35.6685169327689,-31.3542812459709,1.83166815244295));
#28945=CARTESIAN_POINT('Ctrl Pts',(36.892775700917,-31.8132156512101,1.77933477665887));
#28946=CARTESIAN_POINT('Ctrl Pts',(37.651188423337,-32.679834131615,1.72700140087478));
#28947=CARTESIAN_POINT('Ctrl Pts',(38.409601145757,-33.5464526120198,1.6746680250907));
#28948=CARTESIAN_POINT('Ctrl Pts',(38.7021678224488,-34.8207551675903,1.62233464930661));
#28949=CARTESIAN_POINT('Ctrl Pts',(38.3977155653522,-35.9313944817532,1.57000127352253));
#28950=CARTESIAN_POINT('Ctrl Pts',(38.0932633082556,-37.0420337959161,1.51766789773845));
#28951=CARTESIAN_POINT('Ctrl Pts',(37.1917921173706,-37.9890098686715,1.46533452195436));
#28952=CARTESIAN_POINT('Ctrl Pts',(36.0974793449018,-38.347756846785,1.41300114617028));
#28953=CARTESIAN_POINT('Ctrl Pts',(35.0031665724331,-38.7065038248986,1.36066777038619));
#28954=CARTESIAN_POINT('Ctrl Pts',(33.7160122183805,-38.4770217083703,1.30833439460211));
#28955=CARTESIAN_POINT('Ctrl Pts',(32.8131212940369,-37.7621688707036,1.25600101881802));
#28956=CARTESIAN_POINT('Ctrl Pts',(31.9883413614044,-37.10915945462,1.20819511337601));
#28957=CARTESIAN_POINT('Ctrl Pts',(31.4842139440677,-36.051127518694,1.16038920793399));
#28958=CARTESIAN_POINT('Ctrl Pts',(31.4779839561681,-34.998317589092,1.11258330249197));
#28959=CARTESIAN_POINT('Ctrl Pts',(31.4787693262007,-35.0021519651487,1.38741669750802));
#28960=CARTESIAN_POINT('Ctrl Pts',(31.4777790283158,-35.1386120640087,1.39360934874047));
#28961=CARTESIAN_POINT('Ctrl Pts',(31.4850406303498,-35.2749658775635,1.39980199997291));
#28962=CARTESIAN_POINT('Ctrl Pts',(31.5009112501032,-35.4103101518596,1.40599465120536));
#28963=CARTESIAN_POINT('Ctrl Pts',(31.6350320129721,-36.554088882664,1.45832802698944));
#28964=CARTESIAN_POINT('Ctrl Pts',(32.3839867518631,-37.6257689075961,1.51066140277353));
#28965=CARTESIAN_POINT('Ctrl Pts',(33.4119755528977,-38.1448602359127,1.56299477855761));
#28966=CARTESIAN_POINT('Ctrl Pts',(34.4399643539324,-38.6639515642293,1.6153281543417));
#28967=CARTESIAN_POINT('Ctrl Pts',(35.7469872171107,-38.6304541959304,1.66766153012578));
#28968=CARTESIAN_POINT('Ctrl Pts',(36.7470353952608,-38.0593854028254,1.71999490590987));
#28969=CARTESIAN_POINT('Ctrl Pts',(37.7470835734109,-37.4883166097203,1.77232828169395));
#28970=CARTESIAN_POINT('Ctrl Pts',(38.4401570665328,-36.3796763918093,1.82466165747804));
#28971=CARTESIAN_POINT('Ctrl Pts',(38.5155124424211,-35.2305296204218,1.87699503326212));
#28972=CARTESIAN_POINT('Ctrl Pts',(38.5908678183095,-34.0813828490343,1.9293284090462));
#28973=CARTESIAN_POINT('Ctrl Pts',(38.0485050769643,-32.8917295241703,1.98166178483029));
#28974=CARTESIAN_POINT('Ctrl Pts',(37.1315954563618,-32.1949560672859,2.03399516061437));
#28975=CARTESIAN_POINT('Ctrl Pts',(36.2146858357593,-31.4981826104015,2.08632853639846));
#28976=CARTESIAN_POINT('Ctrl Pts',(34.9232293358993,-31.2942890214966,2.13866191218254));
#28977=CARTESIAN_POINT('Ctrl Pts',(33.8362565237849,-31.6746921445243,2.19099528796663));
#28978=CARTESIAN_POINT('Ctrl Pts',(32.7492837116705,-32.055095267552,2.24332866375071));
#28979=CARTESIAN_POINT('Ctrl Pts',(31.8667945873017,-33.0197951025121,2.2956620395348));
#28980=CARTESIAN_POINT('Ctrl Pts',(31.5844574569229,-34.1362637639197,2.34799541531888));
#28981=CARTESIAN_POINT('Ctrl Pts',(31.5135652106755,-34.4165987349732,2.36113584271526));
#28982=CARTESIAN_POINT('Ctrl Pts',(31.4805104906949,-34.7065022103634,2.37427627011164));
#28983=CARTESIAN_POINT('Ctrl Pts',(31.4830375605149,-34.9969726960772,2.38741669750802));
#28984=CARTESIAN_POINT('Origin',(35.,-35.,4.));
#28985=CARTESIAN_POINT('',(31.486635086556,-35.0020090496756,3.38741669750802));
#28986=CARTESIAN_POINT('',(31.4804772106861,-35.0027703375482,3.11258330249198));
#28987=CARTESIAN_POINT('',(31.4825,-35.,4.));
#28988=CARTESIAN_POINT('Ctrl Pts',(31.4804772106861,-35.0027703375482,3.11258330249198));
#28989=CARTESIAN_POINT('Ctrl Pts',(31.4887009944635,-34.0497596813621,3.06938967489225));
#28990=CARTESIAN_POINT('Ctrl Pts',(31.8903812384068,-33.090636581221,3.02619604729253));
#28991=CARTESIAN_POINT('Ctrl Pts',(32.5815435480781,-32.4381583394347,2.98300241969281));
#28992=CARTESIAN_POINT('Ctrl Pts',(33.4189554277892,-31.647616055402,2.93066904390873));
#28993=CARTESIAN_POINT('Ctrl Pts',(34.6813192352892,-31.3072202195671,2.87833566812464));
#28994=CARTESIAN_POINT('Ctrl Pts',(35.8026481051029,-31.5695889094262,2.82600229234056));
#28995=CARTESIAN_POINT('Ctrl Pts',(36.9239769749167,-31.8319575992854,2.77366891655647));
#28996=CARTESIAN_POINT('Ctrl Pts',(37.904270907044,-32.6970908148387,2.72133554077239));
#28997=CARTESIAN_POINT('Ctrl Pts',(38.3040104089138,-33.7771019860347,2.66900216498831));
#28998=CARTESIAN_POINT('Ctrl Pts',(38.7037499107836,-34.8571131572306,2.61666878920422));
#28999=CARTESIAN_POINT('Ctrl Pts',(38.5229349823959,-36.1520022840693,2.56433541342014));
#29000=CARTESIAN_POINT('Ctrl Pts',(37.8426348759932,-37.0811995004531,2.51200203763605));
#29001=CARTESIAN_POINT('Ctrl Pts',(37.1623347695905,-38.0103967168369,2.45966866185197));
#29002=CARTESIAN_POINT('Ctrl Pts',(35.9825494851727,-38.5739020227658,2.40733528606788));
#29003=CARTESIAN_POINT('Ctrl Pts',(34.832241390481,-38.5190653424433,2.3550019102838));
#29004=CARTESIAN_POINT('Ctrl Pts',(33.6819332957892,-38.4642286621207,2.30266853449971));
#29005=CARTESIAN_POINT('Ctrl Pts',(32.5611023908235,-37.7910499955468,2.25033515871563));
#29006=CARTESIAN_POINT('Ctrl Pts',(31.9722786359356,-36.8013517615434,2.19800178293155));
#29007=CARTESIAN_POINT('Ctrl Pts',(31.6519194665675,-36.2628902923203,2.16952895611836));
#29008=CARTESIAN_POINT('Ctrl Pts',(31.4890387510844,-35.6307364505496,2.14105612930517));
#29009=CARTESIAN_POINT('Ctrl Pts',(31.4877390119671,-34.9992080277921,2.11258330249198));
#29010=CARTESIAN_POINT('Ctrl Pts',(31.4830375605149,-34.9969726960772,2.38741669750802));
#29011=CARTESIAN_POINT('Ctrl Pts',(31.490574858507,-35.8633368112863,2.42660964589573));
#29012=CARTESIAN_POINT('Ctrl Pts',(31.8146493000371,-36.734745074899,2.46580259428343));
#29013=CARTESIAN_POINT('Ctrl Pts',(32.3954081923274,-37.3723559095391,2.50499554267113));
#29014=CARTESIAN_POINT('Ctrl Pts',(33.1708811944992,-38.223741905896,2.55732891845522));
#29015=CARTESIAN_POINT('Ctrl Pts',(34.4040123352312,-38.6582764107548,2.60966229423931));
#29016=CARTESIAN_POINT('Ctrl Pts',(35.5419213707996,-38.4811337730552,2.66199567002339));
#29017=CARTESIAN_POINT('Ctrl Pts',(36.679830406368,-38.3039911353557,2.71432904580747));
#29018=CARTESIAN_POINT('Ctrl Pts',(37.7225173367726,-37.5151713550979,2.76666242159156));
#29019=CARTESIAN_POINT('Ctrl Pts',(38.2024884661482,-36.4683455751991,2.81899579737564));
#29020=CARTESIAN_POINT('Ctrl Pts',(38.6824595955238,-35.4215197953004,2.87132917315972));
#29021=CARTESIAN_POINT('Ctrl Pts',(38.5997149238704,-34.1166880157607,2.92366254894381));
#29022=CARTESIAN_POINT('Ctrl Pts',(37.9913534261364,-33.1388778186484,2.97599592472789));
#29023=CARTESIAN_POINT('Ctrl Pts',(37.3829919284024,-32.161067621536,3.02832930051198));
#29024=CARTESIAN_POINT('Ctrl Pts',(36.2490136045879,-31.510279006851,3.08066267629606));
#29025=CARTESIAN_POINT('Ctrl Pts',(35.0978430733873,-31.4782961743034,3.13299605208015));
#29026=CARTESIAN_POINT('Ctrl Pts',(33.9466725421867,-31.4463133417559,3.18532942786423));
#29027=CARTESIAN_POINT('Ctrl Pts',(32.7783098036,-32.0331362913458,3.23766280364832));
#29028=CARTESIAN_POINT('Ctrl Pts',(32.116595896964,-32.975660137455,3.2899961794324));
#29029=CARTESIAN_POINT('Ctrl Pts',(31.7059942452997,-33.5605078247475,3.32246968545761));
#29030=CARTESIAN_POINT('Ctrl Pts',(31.4904704191383,-34.2823130120804,3.35494319148282));
#29031=CARTESIAN_POINT('Ctrl Pts',(31.486635086556,-35.0020090496756,3.38741669750802));
#29032=CARTESIAN_POINT('Origin',(35.,-35.,4.));
#29033=CARTESIAN_POINT('',(31.4769535111774,-35.000206350087,4.38741669750802));
#29034=CARTESIAN_POINT('',(31.481143567597,-34.9970948481792,4.11258330249198));
#29035=CARTESIAN_POINT('',(31.4825,-35.,4.));
#29036=CARTESIAN_POINT('Ctrl Pts',(31.481143567597,-34.9970948481792,4.11258330249198));
#29037=CARTESIAN_POINT('Ctrl Pts',(31.4791556658517,-34.7720820979161,4.10238997204751));
#29038=CARTESIAN_POINT('Ctrl Pts',(31.4989362834408,-34.5474172520071,4.09219664160305));
#29039=CARTESIAN_POINT('Ctrl Pts',(31.5417700421341,-34.3272371560843,4.08200331115859));
#29040=CARTESIAN_POINT('Ctrl Pts',(31.7616819935963,-33.1968148899876,4.0296699353745));
#29041=CARTESIAN_POINT('Ctrl Pts',(32.5892466030323,-32.1846051588847,3.97733655959042));
#29042=CARTESIAN_POINT('Ctrl Pts',(33.6534213081659,-31.7444370513165,3.92500318380633));
#29043=CARTESIAN_POINT('Ctrl Pts',(34.7175960132996,-31.3042689437483,3.87266980802225));
#29044=CARTESIAN_POINT('Ctrl Pts',(36.0183808141308,-31.4361424597148,3.82033643223816));
#29045=CARTESIAN_POINT('Ctrl Pts',(36.9725626056516,-32.0809314753194,3.76800305645408));
#29046=CARTESIAN_POINT('Ctrl Pts',(37.9267443971724,-32.7257204909241,3.71566968066999));
#29047=CARTESIAN_POINT('Ctrl Pts',(38.5343231793827,-33.883425006167,3.66333630488591));
#29048=CARTESIAN_POINT('Ctrl Pts',(38.5228880907758,-35.0349826492465,3.61100292910183));
#29049=CARTESIAN_POINT('Ctrl Pts',(38.5114530021688,-36.186540292326,3.55866955331774));
#29050=CARTESIAN_POINT('Ctrl Pts',(37.8810040427447,-37.3319510632421,3.50633617753366));
#29051=CARTESIAN_POINT('Ctrl Pts',(36.9142060277602,-37.9576645468416,3.45400280174957));
#29052=CARTESIAN_POINT('Ctrl Pts',(35.9474080127757,-38.5833780304411,3.40166942596549));
#29053=CARTESIAN_POINT('Ctrl Pts',(34.6442609422309,-38.6893942267241,3.3493360501814));
#29054=CARTESIAN_POINT('Ctrl Pts',(33.5890370557646,-38.2281802690192,3.29700267439732));
#29055=CARTESIAN_POINT('Ctrl Pts',(32.5338131692983,-37.7669663113142,3.24466929861323));
#29056=CARTESIAN_POINT('Ctrl Pts',(31.7265124669105,-36.7385221996213,3.19233592282915));
#29057=CARTESIAN_POINT('Ctrl Pts',(31.5290920916777,-35.6039557776596,3.14000254704507));
#29058=CARTESIAN_POINT('Ctrl Pts',(31.4946136639238,-35.4058097333848,3.1308627988607));
#29059=CARTESIAN_POINT('Ctrl Pts',(31.478737062497,-35.2044268757596,3.12172305067634));
#29060=CARTESIAN_POINT('Ctrl Pts',(31.4804772106861,-35.0027703375482,3.11258330249198));
#29061=CARTESIAN_POINT('Ctrl Pts',(31.486635086556,-35.0020090496756,3.38741669750802));
#29062=CARTESIAN_POINT('Ctrl Pts',(31.4842895065774,-35.4421546120773,3.4072765672669));
#29063=CARTESIAN_POINT('Ctrl Pts',(31.5611195851562,-35.8815113110096,3.42713643702578));
#29064=CARTESIAN_POINT('Ctrl Pts',(31.7209248424069,-36.2882690753391,3.44699630678465));
#29065=CARTESIAN_POINT('Ctrl Pts',(32.1420327691713,-37.3601294244856,3.49932968256874));
#29066=CARTESIAN_POINT('Ctrl Pts',(33.1393136973855,-38.2056253801502,3.55166305835282));
#29067=CARTESIAN_POINT('Ctrl Pts',(34.2656319394155,-38.4456747746043,3.60399643413691));
#29068=CARTESIAN_POINT('Ctrl Pts',(35.3919501814454,-38.6857241690583,3.65632980992099));
#29069=CARTESIAN_POINT('Ctrl Pts',(36.647305737291,-38.3203270023018,3.70866318570508));
#29070=CARTESIAN_POINT('Ctrl Pts',(37.4688539216907,-37.5133108469912,3.76099656148916));
#29071=CARTESIAN_POINT('Ctrl Pts',(38.2904021060904,-36.7062946916805,3.81332993727324));
#29072=CARTESIAN_POINT('Ctrl Pts',(38.6781429190441,-35.4576595478158,3.86566331305733));
#29073=CARTESIAN_POINT('Ctrl Pts',(38.4582309072122,-34.3272369713982,3.91799668884141));
#29074=CARTESIAN_POINT('Ctrl Pts',(38.2383188953802,-33.1968143949805,3.9703300646255));
#29075=CARTESIAN_POINT('Ctrl Pts',(37.4107540587627,-32.1846043860099,4.02266344040958));
#29076=CARTESIAN_POINT('Ctrl Pts',(36.346579061494,-31.744436157607,4.07499681619367));
#29077=CARTESIAN_POINT('Ctrl Pts',(35.2824040642253,-31.3042679292041,4.12733019197775));
#29078=CARTESIAN_POINT('Ctrl Pts',(33.9816189063054,-31.4361414813689,4.17966356776183));
#29079=CARTESIAN_POINT('Ctrl Pts',(33.0274368528446,-32.0809306739812,4.23199694354592));
#29080=CARTESIAN_POINT('Ctrl Pts',(32.0828596573675,-32.7192293770668,4.28380352819995));
#29081=CARTESIAN_POINT('Ctrl Pts',(31.477942827805,-33.8601696083914,4.33561011285399));
#29082=CARTESIAN_POINT('Ctrl Pts',(31.4769535111774,-35.000206350087,4.38741669750802));
#29083=CARTESIAN_POINT('Origin',(35.,-35.,4.));
#29084=CARTESIAN_POINT('',(31.4861928568261,-34.9977297533801,5.38741669750802));
#29085=CARTESIAN_POINT('',(31.4875433805768,-35.0011388328632,5.11258330249198));
#29086=CARTESIAN_POINT('',(31.4825,-35.,4.));
#29087=CARTESIAN_POINT('Ctrl Pts',(31.4875433805768,-35.0011388328632,5.11258330249198));
#29088=CARTESIAN_POINT('Ctrl Pts',(31.4894886053032,-34.3463334487764,5.08305689341869));
#29089=CARTESIAN_POINT('Ctrl Pts',(31.6654108801779,-33.6905571677388,5.0535304843454));
#29090=CARTESIAN_POINT('Ctrl Pts',(32.0086473950495,-33.1388783295694,5.02400407527211));
#29091=CARTESIAN_POINT('Ctrl Pts',(32.6170087257827,-32.1610684008923,4.97167069948802));
#29092=CARTESIAN_POINT('Ctrl Pts',(33.7509867382882,-31.5102799648413,4.91933732370394));
#29093=CARTESIAN_POINT('Ctrl Pts',(34.9021569534692,-31.478297141069,4.86700394791986));
#29094=CARTESIAN_POINT('Ctrl Pts',(36.0533271686501,-31.4463143172967,4.81467057213577));
#29095=CARTESIAN_POINT('Ctrl Pts',(37.2216895865065,-32.0331371058031,4.76233719635168));
#29096=CARTESIAN_POINT('Ctrl Pts',(37.8834033114917,-32.975660693175,4.7100038205676));
#29097=CARTESIAN_POINT('Ctrl Pts',(38.5451170364769,-33.9181842805469,4.65767044478351));
#29098=CARTESIAN_POINT('Ctrl Pts',(38.7001820685911,-35.2164086667843,4.60533706899943));
#29099=CARTESIAN_POINT('Ctrl Pts',(38.2790742574276,-36.2882687216848,4.55300369321535));
#29100=CARTESIAN_POINT('Ctrl Pts',(37.8579664462641,-37.3601287765853,4.50067031743126));
#29101=CARTESIAN_POINT('Ctrl Pts',(36.8606857918229,-38.205624500149,4.44833694164718));
#29102=CARTESIAN_POINT('Ctrl Pts',(35.7343678589879,-38.4456738287057,4.39600356586309));
#29103=CARTESIAN_POINT('Ctrl Pts',(34.6080499261528,-38.6857231572625,4.34367019007901));
#29104=CARTESIAN_POINT('Ctrl Pts',(33.3526947149239,-38.3203260908123,4.29133681429492));
#29105=CARTESIAN_POINT('Ctrl Pts',(32.5311467560536,-37.5133101570419,4.23900343851084));
#29106=CARTESIAN_POINT('Ctrl Pts',(31.8696173263776,-36.863482250293,4.19686339317122));
#29107=CARTESIAN_POINT('Ctrl Pts',(31.489361712798,-35.9273155988689,4.1547233478316));
#29108=CARTESIAN_POINT('Ctrl Pts',(31.481143567597,-34.9970948481792,4.11258330249198));
#29109=CARTESIAN_POINT('Ctrl Pts',(31.4769535111774,-35.000206350087,4.38741669750802));
#29110=CARTESIAN_POINT('Ctrl Pts',(31.47694345139,-35.0117987228996,4.38794348863807));
#29111=CARTESIAN_POINT('Ctrl Pts',(31.4769958357584,-35.0233910022943,4.38847027976812));
#29112=CARTESIAN_POINT('Ctrl Pts',(31.4771109421281,-35.034982658853,4.38899707089817));
#29113=CARTESIAN_POINT('Ctrl Pts',(31.4885460338743,-36.1865406180529,4.44133044668226));
#29114=CARTESIAN_POINT('Ctrl Pts',(32.1189951663686,-37.3319517033932,4.49366382246634));
#29115=CARTESIAN_POINT('Ctrl Pts',(33.0857934467562,-37.9576653587677,4.54599719825043));
#29116=CARTESIAN_POINT('Ctrl Pts',(34.0525917271438,-38.5833790141421,4.59833057403451));
#29117=CARTESIAN_POINT('Ctrl Pts',(35.3557391554246,-38.6893952395508,4.6506639498186));
#29118=CARTESIAN_POINT('Ctrl Pts',(36.4109633315695,-38.228181155224,4.70299732560268));
#29119=CARTESIAN_POINT('Ctrl Pts',(37.4661875077144,-37.7669670708972,4.75533070138676));
#29120=CARTESIAN_POINT('Ctrl Pts',(38.2734884317233,-36.738522676835,4.80766407717085));
#29121=CARTESIAN_POINT('Ctrl Pts',(38.47090886115,-35.6039559434342,4.85999745295493));
#29122=CARTESIAN_POINT('Ctrl Pts',(38.6683292905767,-34.4693892100334,4.91233082873902));
#29123=CARTESIAN_POINT('Ctrl Pts',(38.2558692254213,-33.2287001372941,4.9646642045231));
#29124=CARTESIAN_POINT('Ctrl Pts',(37.4184571158289,-32.4381576362056,5.01699758030719));
#29125=CARTESIAN_POINT('Ctrl Pts',(36.5810450062365,-31.6476151351171,5.06933095609127));
#29126=CARTESIAN_POINT('Ctrl Pts',(35.3186808522071,-31.3072192056794,5.12166433187536));
#29127=CARTESIAN_POINT('Ctrl Pts',(34.1973516745615,-31.5695879676355,5.17399770765944));
#29128=CARTESIAN_POINT('Ctrl Pts',(33.0760224969158,-31.8319567295916,5.22633108344352));
#29129=CARTESIAN_POINT('Ctrl Pts',(32.0957282956539,-32.6970901829416,5.27866445922761));
#29130=CARTESIAN_POINT('Ctrl Pts',(31.6959886840635,-33.7771016504831,5.33099783501169));
#29131=CARTESIAN_POINT('Ctrl Pts',(31.5523400478426,-34.1652097336376,5.34980412251047));
#29132=CARTESIAN_POINT('Ctrl Pts',(31.4836621356307,-34.5810663878724,5.36861041000924));
#29133=CARTESIAN_POINT('Ctrl Pts',(31.4861928568261,-34.9977297533801,5.38741669750802));
#29134=CARTESIAN_POINT('Origin',(35.,-35.,4.));
#29135=CARTESIAN_POINT('',(31.4836965554877,-35.0029832498286,6.38741669750802));
#29136=CARTESIAN_POINT('',(31.4775766908735,-35.0013091813966,6.11258330249198));
#29137=CARTESIAN_POINT('',(31.4825,-35.,4.));
#29138=CARTESIAN_POINT('Ctrl Pts',(31.4775766908735,-35.0013091813966,6.11258330249198));
#29139=CARTESIAN_POINT('Ctrl Pts',(31.4827875611424,-33.9256166077537,6.06372381478986));
#29140=CARTESIAN_POINT('Ctrl Pts',(32.0123601793055,-32.8454783123193,6.01486432708774));
#29141=CARTESIAN_POINT('Ctrl Pts',(32.8684051290729,-32.1949568378204,5.96600483938563));
#29142=CARTESIAN_POINT('Ctrl Pts',(33.7853144981881,-31.4981835726539,5.91367146360154));
#29143=CARTESIAN_POINT('Ctrl Pts',(35.0767706429996,-31.2942900387516,5.86133808781746));
#29144=CARTESIAN_POINT('Ctrl Pts',(36.1637431566001,-31.6746930571201,5.80900471203337));
#29145=CARTESIAN_POINT('Ctrl Pts',(37.2507156702007,-32.0550960754886,5.75667133624929));
#29146=CARTESIAN_POINT('Ctrl Pts',(38.1332045525903,-33.0197956461279,5.70433796046521));
#29147=CARTESIAN_POINT('Ctrl Pts',(38.4155416055276,-34.1362640011663,5.65200458468112));
#29148=CARTESIAN_POINT('Ctrl Pts',(38.6978786584649,-35.2527323562045,5.59967120889703));
#29149=CARTESIAN_POINT('Ctrl Pts',(38.3800638819499,-36.5209694956418,5.54733783311295));
#29150=CARTESIAN_POINT('Ctrl Pts',(37.6045910926243,-37.3723552582146,5.49500445732887));
#29151=CARTESIAN_POINT('Ctrl Pts',(36.8291183032988,-38.2237410207875,5.44267108154478));
#29152=CARTESIAN_POINT('Ctrl Pts',(35.5959875011627,-38.658275406496,5.3903377057607));
#29153=CARTESIAN_POINT('Ctrl Pts',(34.4580787779894,-38.4811328174583,5.33800432997662));
#29154=CARTESIAN_POINT('Ctrl Pts',(33.3201700548161,-38.3039902284206,5.28567095419253));
#29155=CARTESIAN_POINT('Ctrl Pts',(32.2774834106055,-37.5151706646368,5.23333757840844));
#29156=CARTESIAN_POINT('Ctrl Pts',(31.7975124129806,-36.4683451720932,5.18100420262436));
#29157=CARTESIAN_POINT('Ctrl Pts',(31.5883403043411,-36.0121369913148,5.15819723591357));
#29158=CARTESIAN_POINT('Ctrl Pts',(31.486040838379,-35.5069275510188,5.13539026920277));
#29159=CARTESIAN_POINT('Ctrl Pts',(31.4875433805768,-35.0011388328632,5.11258330249198));
#29160=CARTESIAN_POINT('Ctrl Pts',(31.4861928568261,-34.9977297533801,5.38741669750802));
#29161=CARTESIAN_POINT('Ctrl Pts',(31.4907045241579,-35.7405403395491,5.42094378579333));
#29162=CARTESIAN_POINT('Ctrl Pts',(31.7215337165433,-36.4859148409341,5.45447087407864));
#29163=CARTESIAN_POINT('Ctrl Pts',(32.1573643436795,-37.081200071482,5.48799796236395));
#29164=CARTESIAN_POINT('Ctrl Pts',(32.8376646368048,-38.0103975432063,5.54033133814803));
#29165=CARTESIAN_POINT('Ctrl Pts',(34.0174502449743,-38.5739030049216,5.59266471393212));
#29166=CARTESIAN_POINT('Ctrl Pts',(35.1677586555142,-38.5190663090568,5.6449980897162));
#29167=CARTESIAN_POINT('Ctrl Pts',(36.318067066054,-38.464229613192,5.69733146550028));
#29168=CARTESIAN_POINT('Ctrl Pts',(37.4388982789643,-37.7910507597469,5.74966484128437));
#29169=CARTESIAN_POINT('Ctrl Pts',(38.0277221953511,-36.8013522549706,5.80199821706845));
#29170=CARTESIAN_POINT('Ctrl Pts',(38.6165461117379,-35.8116537501943,5.85433159285254));
#29171=CARTESIAN_POINT('Ctrl Pts',(38.6733627316013,-34.5054355940866,5.90666496863662));
#29172=CARTESIAN_POINT('Ctrl Pts',(38.172698148003,-33.4683478929687,5.9589983444207));
#29173=CARTESIAN_POINT('Ctrl Pts',(37.6720335644046,-32.4312601918508,6.01133172020479));
#29174=CARTESIAN_POINT('Ctrl Pts',(36.6138877773445,-31.6633029457227,6.06366509598888));
#29175=CARTESIAN_POINT('Ctrl Pts',(35.4726853304849,-31.5087915951115,6.11599847177296));
#29176=CARTESIAN_POINT('Ctrl Pts',(34.3314828836252,-31.3542802445004,6.16833184755705));
#29177=CARTESIAN_POINT('Ctrl Pts',(33.107223776966,-31.8132147894062,6.22066522334113));
#29178=CARTESIAN_POINT('Ctrl Pts',(32.3488108476933,-32.6798335018657,6.27299859912521));
#29179=CARTESIAN_POINT('Ctrl Pts',(31.7960968682859,-33.3114053787477,6.31113796525282));
#29180=CARTESIAN_POINT('Ctrl Pts',(31.4908012796383,-34.1595048683285,6.34927733138042));
#29181=CARTESIAN_POINT('Ctrl Pts',(31.4836965554877,-35.0029832498286,6.38741669750802));
#29182=CARTESIAN_POINT('Origin',(35.,-35.,4.));
#29183=CARTESIAN_POINT('',(31.478260520576,-34.9982347527286,7.38741669750802));
#29184=CARTESIAN_POINT('',(31.4846885160394,-34.9971888045819,7.11258330249198));
#29185=CARTESIAN_POINT('',(31.4825,-35.,4.));
#29186=CARTESIAN_POINT('',(37.6735319337713,-32.7141668369925,8.));
#29187=CARTESIAN_POINT('Ctrl Pts',(31.478260520576,-34.9982347527286,7.38741669750802));
#29188=CARTESIAN_POINT('Ctrl Pts',(31.4849542237249,-36.0376022532878,7.43461100431976));
#29189=CARTESIAN_POINT('Ctrl Pts',(31.9746244075585,-37.0822334042073,7.4818053111315));
#29190=CARTESIAN_POINT('Ctrl Pts',(32.7813940610787,-37.7364867433061,7.52899961794324));
#29191=CARTESIAN_POINT('Ctrl Pts',(33.6760142451889,-38.4619828500639,7.58133299372733));
#29192=CARTESIAN_POINT('Ctrl Pts',(34.9605528856554,-38.7074544587316,7.63366636951141));
#29193=CARTESIAN_POINT('Ctrl Pts',(36.0588772142959,-38.3607385729207,7.6859997452955));
#29194=CARTESIAN_POINT('Ctrl Pts',(37.1572015429365,-38.0140226871098,7.73833312107958));
#29195=CARTESIAN_POINT('Ctrl Pts',(38.069311559751,-37.0751193068202,7.79066649686367));
#29196=CARTESIAN_POINT('Ctrl Pts',(38.386301242806,-35.9699332359521,7.84299987264775));
#29197=CARTESIAN_POINT('Ctrl Pts',(38.703290925861,-34.864747165084,7.89533324843183));
#29198=CARTESIAN_POINT('Ctrl Pts',(38.4251602751564,-33.5932784036374,7.94766662421592));
#29199=CARTESIAN_POINT('Ctrl Pts',(37.6735319337713,-32.7141668369925,8.));
#29200=CARTESIAN_POINT('',(32.3214996650065,-32.7109746768979,8.));
#29201=CARTESIAN_POINT('Origin',(35.,-35.,8.));
#29202=CARTESIAN_POINT('Ctrl Pts',(32.3214765561793,-32.7109598296518,8.));
#29203=CARTESIAN_POINT('Ctrl Pts',(33.0392495465109,-31.8766737967152,7.95000212253756));
#29204=CARTESIAN_POINT('Ctrl Pts',(34.181330417556,-31.4010809746138,7.90000424507511));
#29205=CARTESIAN_POINT('Ctrl Pts',(35.2782977952799,-31.4881472942925,7.85000636761267));
#29206=CARTESIAN_POINT('Ctrl Pts',(36.4265066576347,-31.5792806514897,7.79767299182859));
#29207=CARTESIAN_POINT('Ctrl Pts',(37.5252889103119,-32.2868666869212,7.74533961604451));
#29208=CARTESIAN_POINT('Ctrl Pts',(38.0826699468004,-33.2944463733222,7.69300624026042));
#29209=CARTESIAN_POINT('Ctrl Pts',(38.6400509832889,-34.302026059723,7.64067286447634));
#29210=CARTESIAN_POINT('Ctrl Pts',(38.6560308035887,-35.6095993970933,7.58833948869224));
#29211=CARTESIAN_POINT('Ctrl Pts',(38.1231125366528,-36.6305184803578,7.53600611290816));
#29212=CARTESIAN_POINT('Ctrl Pts',(37.5901942697169,-37.6514375636223,7.48367273712407));
#29213=CARTESIAN_POINT('Ctrl Pts',(36.5083779155453,-38.3857023927811,7.43133936133999));
#29214=CARTESIAN_POINT('Ctrl Pts',(35.3628659911708,-38.5042959466132,7.37900598555591));
#29215=CARTESIAN_POINT('Ctrl Pts',(34.2173540667963,-38.6228895004453,7.32667260977183));
#29216=CARTESIAN_POINT('Ctrl Pts',(33.0081465722189,-38.1258117789507,7.27433923398774));
#29217=CARTESIAN_POINT('Ctrl Pts',(32.2773155686706,-37.2358335624551,7.22200585820366));
#29218=CARTESIAN_POINT('Ctrl Pts',(31.7679567703675,-36.6155557791246,7.18553167296643));
#29219=CARTESIAN_POINT('Ctrl Pts',(31.4909698285316,-35.80442618944,7.1490574877292));
#29220=CARTESIAN_POINT('Ctrl Pts',(31.4846885160394,-34.9971888045819,7.11258330249198));
#29221=CARTESIAN_POINT('Origin',(-35.,35.,10.2084234471775));
#29222=CARTESIAN_POINT('',(-39.0787305107814,35.0019482814736,0.791576552822544));
#29223=CARTESIAN_POINT('',(-39.0671617292797,34.9998409589035,0.708423447177453));
#29224=CARTESIAN_POINT('',(-39.0735,35.0000000000001,10.2084234471775));
#29225=CARTESIAN_POINT('',(-33.9479286229388,31.0647048309474,0.));
#29226=CARTESIAN_POINT('Ctrl Pts',(-39.0671617292797,34.9998409589035,0.708423447177453));
#29227=CARTESIAN_POINT('Ctrl Pts',(-39.0667162804106,35.6885579272407,0.68161580125464));
#29228=CARTESIAN_POINT('Ctrl Pts',(-38.5762700272017,37.7222374436051,0.602474779547742));
#29229=CARTESIAN_POINT('Ctrl Pts',(-35.379526836985,39.7808556694562,0.471000382056761));
#29230=CARTESIAN_POINT('Ctrl Pts',(-31.2187001848465,37.9557862959725,0.314000254704507));
#29231=CARTESIAN_POINT('Ctrl Pts',(-30.4549372314006,33.4726351387477,0.157000127352253));
#29232=CARTESIAN_POINT('Ctrl Pts',(-32.6539236935135,31.4106472544613,0.0523333757840845));
#29233=CARTESIAN_POINT('Ctrl Pts',(-33.9479286229388,31.0647048309474,0.));
#29234=CARTESIAN_POINT('',(-36.0547197101746,31.058399207452,2.73005324693302E-15));
#29235=CARTESIAN_POINT('Origin',(-35.,35.,0.));
#29236=CARTESIAN_POINT('Ctrl Pts',(-39.0787305107814,35.0019482814736,0.791576552822544));
#29237=CARTESIAN_POINT('Ctrl Pts',(-39.0794137856881,35.117415240318,0.787049082480477));
#29238=CARTESIAN_POINT('Ctrl Pts',(-39.0230450544057,36.5668924114048,0.730188236354325));
#29239=CARTESIAN_POINT('Ctrl Pts',(-37.2955092110801,39.2117686241983,0.620994014444089));
#29240=CARTESIAN_POINT('Ctrl Pts',(-32.7531819533668,39.2384377406302,0.463993887091835));
#29241=CARTESIAN_POINT('Ctrl Pts',(-30.2257196451616,35.46328448449,0.306993759739582));
#29242=CARTESIAN_POINT('Ctrl Pts',(-31.9530720002325,31.3373697401077,0.152329130708971));
#29243=CARTESIAN_POINT('Ctrl Pts',(-34.822442511108,30.7329994872565,0.0499978774624443));
#29244=CARTESIAN_POINT('Ctrl Pts',(-36.0547320440515,31.0583698407595,2.40774197454718E-15));
#29245=CARTESIAN_POINT('Origin',(-35.,35.,10.2084234471775));
#29246=CARTESIAN_POINT('',(-39.0674335213841,35.0009171557363,1.79157655282254));
#29247=CARTESIAN_POINT('',(-39.0778197532985,34.9975078784707,1.70842344717745));
#29248=CARTESIAN_POINT('',(-39.0735,35.0000000000001,10.2084234471775));
#29249=CARTESIAN_POINT('Ctrl Pts',(-39.0778197532985,34.9975078784707,1.70842344717745));
#29250=CARTESIAN_POINT('Ctrl Pts',(-39.0692748471557,36.1749702057365,1.66228272262582));
#29251=CARTESIAN_POINT('Ctrl Pts',(-37.9187924724061,38.702508200362,1.56380862229009));
#29252=CARTESIAN_POINT('Ctrl Pts',(-33.6495204180096,39.602789266723,1.41300114617028));
#29253=CARTESIAN_POINT('Ctrl Pts',(-30.4158794824773,36.4127281948833,1.25600101881803));
#29254=CARTESIAN_POINT('Ctrl Pts',(-31.2929570903083,31.9557501199225,1.09900089146578));
#29255=CARTESIAN_POINT('Ctrl Pts',(-35.4939869156159,30.2288018345407,0.942000764113521));
#29256=CARTESIAN_POINT('Ctrl Pts',(-38.6106822216958,32.3442076080298,0.811808282684081));
#29257=CARTESIAN_POINT('Ctrl Pts',(-39.0675858772087,34.3440577791618,0.733949177038725));
#29258=CARTESIAN_POINT('Ctrl Pts',(-39.0671617292797,34.9998409589035,0.708423447177453));
#29259=CARTESIAN_POINT('Ctrl Pts',(-39.0674335213841,35.0009171557363,1.79157655282255));
#29260=CARTESIAN_POINT('Ctrl Pts',(-39.0686948832473,35.6137985390812,1.76771600385165));
#29261=CARTESIAN_POINT('Ctrl Pts',(-38.6530957043657,37.569289309386,1.69152207909667));
#29262=CARTESIAN_POINT('Ctrl Pts',(-35.6435862778458,39.7534633517259,1.56299477855761));
#29263=CARTESIAN_POINT('Ctrl Pts',(-31.3902652615342,38.1590329639038,1.40599465120536));
#29264=CARTESIAN_POINT('Ctrl Pts',(-30.3738298371754,33.7318498284919,1.2489945238531));
#29265=CARTESIAN_POINT('Ctrl Pts',(-33.5057219097166,30.4418645346457,1.09199439650085));
#29266=CARTESIAN_POINT('Ctrl Pts',(-37.8485989831919,31.216140614721,0.939521739490665));
#29267=CARTESIAN_POINT('Ctrl Pts',(-39.0715157588091,33.7827238362241,0.839382458264561));
#29268=CARTESIAN_POINT('Ctrl Pts',(-39.0787305107814,35.0019482814736,0.791576552822544));
#29269=CARTESIAN_POINT('Origin',(-35.,35.,10.2084234471775));
#29270=CARTESIAN_POINT('',(-39.0758431739381,34.9967917635303,2.79157655282255));
#29271=CARTESIAN_POINT('',(-39.0728768523265,35.0035058195583,2.70842344717746));
#29272=CARTESIAN_POINT('',(-39.0735,35.0000000000001,10.2084234471775));
#29273=CARTESIAN_POINT('Ctrl Pts',(-39.0728768523265,35.0035058195583,2.70842344717746));
#29274=CARTESIAN_POINT('Ctrl Pts',(-39.075803367569,35.3398899970603,2.69528301978107));
#29275=CARTESIAN_POINT('Ctrl Pts',(-38.8850706886071,37.0126939576436,2.62980921660061));
#29276=CARTESIAN_POINT('Ctrl Pts',(-36.5844982252159,39.5275826001387,2.51200203763606));
#29277=CARTESIAN_POINT('Ctrl Pts',(-32.0977201830868,38.819215512031,2.3550019102838));
#29278=CARTESIAN_POINT('Ctrl Pts',(-30.2134435993119,34.6861220528707,2.19800178293155));
#29279=CARTESIAN_POINT('Ctrl Pts',(-32.6213194634248,30.8344843115421,2.04100165557929));
#29280=CARTESIAN_POINT('Ctrl Pts',(-37.1621781583154,30.7181077707172,1.88400152822704));
#29281=CARTESIAN_POINT('Ctrl Pts',(-38.9994901450348,33.3471191547144,1.77314212542643));
#29282=CARTESIAN_POINT('Ctrl Pts',(-39.0789665845212,34.8394779904932,1.7146160984099));
#29283=CARTESIAN_POINT('Ctrl Pts',(-39.0778197532985,34.9975078784707,1.70842344717745));
#29284=CARTESIAN_POINT('Ctrl Pts',(-39.0758431739381,34.9967917635303,2.79157655282255));
#29285=CARTESIAN_POINT('Ctrl Pts',(-39.0663194813852,36.100441948558,2.74838292522283));
#29286=CARTESIAN_POINT('Ctrl Pts',(-38.0375439399374,38.5569291706849,2.65285592183902));
#29287=CARTESIAN_POINT('Ctrl Pts',(-33.9071518161688,39.6706875589806,2.50499554267113));
#29288=CARTESIAN_POINT('Ctrl Pts',(-30.5014136769744,36.6650408935442,2.34799541531887));
#29289=CARTESIAN_POINT('Ctrl Pts',(-31.1296010783918,32.1663358219723,2.19099528796663));
#29290=CARTESIAN_POINT('Ctrl Pts',(-35.2284122688067,30.2086051339802,2.03399516061437));
#29291=CARTESIAN_POINT('Ctrl Pts',(-38.5306034134223,32.1919236036427,1.90085558223301));
#29292=CARTESIAN_POINT('Ctrl Pts',(-39.0659283364897,34.2695649347001,1.82004937963574));
#29293=CARTESIAN_POINT('Ctrl Pts',(-39.0674335213841,35.0009171557363,1.79157655282255));
#29294=CARTESIAN_POINT('Origin',(-35.,35.,10.2084234471775));
#29295=CARTESIAN_POINT('',(-39.0750714879939,35.0033643604342,3.79157655282255));
#29296=CARTESIAN_POINT('',(-39.0687106773974,34.997673386605,3.70842344717746));
#29297=CARTESIAN_POINT('',(-39.0735,35.0000000000001,10.2084234471775));
#29298=CARTESIAN_POINT('Ctrl Pts',(-39.0687106773974,34.997673386605,3.70842344717746));
#29299=CARTESIAN_POINT('Ctrl Pts',(-39.0642691067062,35.8311293539699,3.67594994115225));
#29300=CARTESIAN_POINT('Ctrl Pts',(-38.4124444982778,38.0141380355395,3.59114305934295));
#29301=CARTESIAN_POINT('Ctrl Pts',(-34.866781479659,39.7949860223284,3.45400280174958));
#29302=CARTESIAN_POINT('Ctrl Pts',(-30.9271141000824,37.5340162820022,3.29700267439732));
#29303=CARTESIAN_POINT('Ctrl Pts',(-30.6396425700269,33.0007698436185,3.14000254704507));
#29304=CARTESIAN_POINT('Ctrl Pts',(-34.2621453998186,30.2602522415144,2.98300241969281));
#29305=CARTESIAN_POINT('Ctrl Pts',(-38.1877198129624,31.6435581024348,2.83914271973695));
#29306=CARTESIAN_POINT('Ctrl Pts',(-39.064148159005,34.0001984453322,2.74761639556516));
#29307=CARTESIAN_POINT('Ctrl Pts',(-39.0728768523265,35.0035058195583,2.70842344717746));
#29308=CARTESIAN_POINT('Ctrl Pts',(-39.0750714879939,35.0033643604342,3.79157655282255));
#29309=CARTESIAN_POINT('Ctrl Pts',(-39.0773736113907,35.2639441995514,3.78138322237809));
#29310=CARTESIAN_POINT('Ctrl Pts',(-38.9368585171591,36.8598904257655,3.71885651614954));
#29311=CARTESIAN_POINT('Ctrl Pts',(-36.8334386787628,39.4326225179073,3.6039964341369));
#29312=CARTESIAN_POINT('Ctrl Pts',(-32.314250849668,38.9744674195804,3.44699630678465));
#29313=CARTESIAN_POINT('Ctrl Pts',(-30.2034000494222,34.9523692588031,3.2899961794324));
#29314=CARTESIAN_POINT('Ctrl Pts',(-32.3937064417451,30.9729820366429,3.13299605208014));
#29315=CARTESIAN_POINT('Ctrl Pts',(-36.9211012705904,30.6046604636344,2.97599592472789));
#29316=CARTESIAN_POINT('Ctrl Pts',(-38.9541946698804,33.1946779489209,2.86218942497536));
#29317=CARTESIAN_POINT('Ctrl Pts',(-39.0778583821194,34.7632599826793,2.80071630100691));
#29318=CARTESIAN_POINT('Ctrl Pts',(-39.0758431739381,34.9967917635303,2.79157655282255));
#29319=CARTESIAN_POINT('Origin',(-35.,35.,10.2084234471775));
#29320=CARTESIAN_POINT('',(-39.0676600758127,34.9986811552388,4.79157655282255));
#29321=CARTESIAN_POINT('',(-39.0799225868021,34.9997610328513,4.70842344717746));
#29322=CARTESIAN_POINT('',(-39.0735,35.0000000000001,10.2084234471775));
#29323=CARTESIAN_POINT('Ctrl Pts',(-39.0799225868021,34.9997610328513,4.70842344717746));
#29324=CARTESIAN_POINT('Ctrl Pts',(-39.0787768922257,36.3199995443189,4.65661686252342));
#29325=CARTESIAN_POINT('Ctrl Pts',(-37.6705855754179,38.9760045490164,4.5524769020853));
#29326=CARTESIAN_POINT('Ctrl Pts',(-33.1665613873943,39.4326223579625,4.3960035658631));
#29327=CARTESIAN_POINT('Ctrl Pts',(-30.2914357144823,35.9160024456566,4.23900343851084));
#29328=CARTESIAN_POINT('Ctrl Pts',(-31.6385248082081,31.5779943532675,4.08200331115859));
#29329=CARTESIAN_POINT('Ctrl Pts',(-35.9998809552364,30.3085315529294,3.92500318380634));
#29330=CARTESIAN_POINT('Ctrl Pts',(-38.7479935181635,32.6383846484188,3.80047656247929));
#29331=CARTESIAN_POINT('Ctrl Pts',(-39.0714270153063,34.4879554969268,3.72828331693633));
#29332=CARTESIAN_POINT('Ctrl Pts',(-39.0687106773974,34.997673386605,3.70842344717746));
#29333=CARTESIAN_POINT('Ctrl Pts',(-39.0676600758127,34.9986811552388,4.79157655282255));
#29334=CARTESIAN_POINT('Ctrl Pts',(-39.065407375266,35.756989657491,4.76205014374926));
#29335=CARTESIAN_POINT('Ctrl Pts',(-38.500581632009,37.8624610972284,4.68019035889188));
#29336=CARTESIAN_POINT('Ctrl Pts',(-35.1332185251462,39.7949861953461,4.54599719825043));
#29337=CARTESIAN_POINT('Ctrl Pts',(-31.0740926686951,37.7562458887763,4.38899707089817));
#29338=CARTESIAN_POINT('Ctrl Pts',(-30.5353655822401,33.2459534545604,4.23199694354592));
#29339=CARTESIAN_POINT('Ctrl Pts',(-34.0001190086845,30.3085313836444,4.07499681619366));
#29340=CARTESIAN_POINT('Ctrl Pts',(-38.0783115555367,31.4955735687615,3.92819001928588));
#29341=CARTESIAN_POINT('Ctrl Pts',(-39.0655543252915,33.9261064127185,3.83371659816217));
#29342=CARTESIAN_POINT('Ctrl Pts',(-39.0750714879939,35.0033643604342,3.79157655282255));
#29343=CARTESIAN_POINT('Origin',(-35.,35.,10.2084234471775));
#29344=CARTESIAN_POINT('',(-39.0792021698116,34.998483879503,5.79157655282255));
#29345=CARTESIAN_POINT('',(-39.0692228089002,35.0026290967949,5.70842344717746));
#29346=CARTESIAN_POINT('',(-39.0735,35.0000000000001,10.2084234471775));
#29347=CARTESIAN_POINT('Ctrl Pts',(-39.0692228089002,35.0026290967949,5.70842344717746));
#29348=CARTESIAN_POINT('Ctrl Pts',(-39.0721535526687,35.4851530378365,5.68961715967868));
#29349=CARTESIAN_POINT('Ctrl Pts',(-38.7712970745332,37.3068911247937,5.61847749639582));
#29350=CARTESIAN_POINT('Ctrl Pts',(-36.092848144401,39.6706873903976,5.49500445732886));
#29351=CARTESIAN_POINT('Ctrl Pts',(-31.7071427262397,38.4880838865661,5.33800432997662));
#29352=CARTESIAN_POINT('Ctrl Pts',(-30.2741740089879,34.1776820335287,5.18100420262436));
#29353=CARTESIAN_POINT('Ctrl Pts',(-33.0788987987297,30.6046606222411,5.02400407527212));
#29354=CARTESIAN_POINT('Ctrl Pts',(-37.6062934642105,30.9729821819491,4.86700394791985));
#29355=CARTESIAN_POINT('Ctrl Pts',(-39.073846927859,33.6392591565121,4.76181040522164));
#29356=CARTESIAN_POINT('Ctrl Pts',(-39.0799342367062,34.9863362926946,4.70895023830751));
#29357=CARTESIAN_POINT('Ctrl Pts',(-39.0799225868021,34.9997610328513,4.70842344717746));
#29358=CARTESIAN_POINT('Ctrl Pts',(-39.0792021698116,34.998483879503,5.79157655282255));
#29359=CARTESIAN_POINT('Ctrl Pts',(-39.0731676328035,36.2442079435004,5.74271706512043));
#29360=CARTESIAN_POINT('Ctrl Pts',(-37.8030025161425,38.8348894467969,5.64152420163423));
#29361=CARTESIAN_POINT('Ctrl Pts',(-33.4155017175264,39.5275827633586,5.48799796236395));
#29362=CARTESIAN_POINT('Ctrl Pts',(-30.3495579785441,36.176022571197,5.33099783501169));
#29363=CARTESIAN_POINT('Ctrl Pts',(-31.4537103860929,31.7699118586619,5.17399770765944));
#29364=CARTESIAN_POINT('Ctrl Pts',(-35.7378546268185,30.2602520705083,5.01699758030719));
#29365=CARTESIAN_POINT('Ctrl Pts',(-38.6790874120226,32.4853711659013,4.88952386202822));
#29366=CARTESIAN_POINT('Ctrl Pts',(-39.0694001203352,34.4129439352318,4.81438351953334));
#29367=CARTESIAN_POINT('Ctrl Pts',(-39.0676600758127,34.9986811552388,4.79157655282255));
#29368=CARTESIAN_POINT('Origin',(-35.,35.,10.2084234471775));
#29369=CARTESIAN_POINT('',(-39.070966199943,35.0032555604945,6.79157655282255));
#29370=CARTESIAN_POINT('',(-39.0721136942453,34.9965451882256,6.70842344717746));
#29371=CARTESIAN_POINT('',(-39.0735,35.0000000000001,10.2084234471775));
#29372=CARTESIAN_POINT('Ctrl Pts',(-39.0721136942453,34.9965451882256,6.70842344717746));
#29373=CARTESIAN_POINT('Ctrl Pts',(-39.0638859499781,35.9733493601025,6.67028408104985));
#29374=CARTESIAN_POINT('Ctrl Pts',(-38.2252019424137,38.3031815231405,6.57981133913817));
#29375=CARTESIAN_POINT('Ctrl Pts',(-34.3564137457339,39.7534631780217,6.4370052214424));
#29376=CARTESIAN_POINT('Ctrl Pts',(-30.6802037555765,37.0854262040492,6.28000509409013));
#29377=CARTESIAN_POINT('Ctrl Pts',(-30.8775960516807,32.5473632088007,6.12300496673789));
#29378=CARTESIAN_POINT('Ctrl Pts',(-34.7715877393978,30.2086053071985,5.96600483938563));
#29379=CARTESIAN_POINT('Ctrl Pts',(-38.3794219899756,31.9318288223888,5.82781099953215));
#29380=CARTESIAN_POINT('Ctrl Pts',(-39.0639979975134,34.142404941861,5.74195053546276));
#29381=CARTESIAN_POINT('Ctrl Pts',(-39.0692228089002,35.0026290967949,5.70842344717746));
#29382=CARTESIAN_POINT('Ctrl Pts',(-39.070966199943,35.0032555604945,6.79157655282255));
#29383=CARTESIAN_POINT('Ctrl Pts',(-39.0741290517156,35.409727295843,6.77571736227569));
#29384=CARTESIAN_POINT('Ctrl Pts',(-38.8328829256554,37.1538415310843,6.70752479594475));
#29385=CARTESIAN_POINT('Ctrl Pts',(-36.3504796357983,39.6027894460767,6.58699885382972));
#29386=CARTESIAN_POINT('Ctrl Pts',(-31.905897053523,38.6655398223873,6.42999872647746));
#29387=CARTESIAN_POINT('Ctrl Pts',(-30.2358031812474,34.4413383659989,6.27299859912522));
#29388=CARTESIAN_POINT('Ctrl Pts',(-32.8378217627235,30.7181076142107,6.11599847177296));
#29389=CARTESIAN_POINT('Ctrl Pts',(-37.3786806229274,30.8344841622903,5.95899834442071));
#29390=CARTESIAN_POINT('Ctrl Pts',(-39.0372095034026,33.4874666211437,5.85085770477057));
#29391=CARTESIAN_POINT('Ctrl Pts',(-39.0796312227382,34.9099134465561,5.79505044090451));
#29392=CARTESIAN_POINT('Ctrl Pts',(-39.0792021698116,34.998483879503,5.79157655282255));
#29393=CARTESIAN_POINT('Origin',(-35.,35.,10.2084234471775));
#29394=CARTESIAN_POINT('',(-39.0691248821302,34.9959228837483,7.79157655282255));
#29395=CARTESIAN_POINT('',(-39.0784090602678,35.0020440536087,7.70842344717746));
#29396=CARTESIAN_POINT('',(-39.0735,35.0000000000001,10.2084234471775));
#29397=CARTESIAN_POINT('',(-36.0520713770612,31.0647048309474,8.));
#29398=CARTESIAN_POINT('Ctrl Pts',(-36.0520713770612,31.0647048309474,8.));
#29399=CARTESIAN_POINT('Ctrl Pts',(-37.3460763064866,31.4106472544613,7.94766662421592));
#29400=CARTESIAN_POINT('Ctrl Pts',(-38.8056938328118,32.7793309690615,7.87819214182344));
#29401=CARTESIAN_POINT('Ctrl Pts',(-39.0721267560147,34.5563414191054,7.80871765943095));
#29402=CARTESIAN_POINT('Ctrl Pts',(-39.0691248821302,34.9959228837483,7.79157655282255));
#29403=CARTESIAN_POINT('',(-33.9452804362612,31.0583992034428,8.));
#29404=CARTESIAN_POINT('Origin',(-35.,35.,8.));
#29405=CARTESIAN_POINT('Ctrl Pts',(-33.9452681066883,31.058369845356,8.));
#29406=CARTESIAN_POINT('Ctrl Pts',(-35.1775577544271,30.7329993831125,7.95000212253756));
#29407=CARTESIAN_POINT('Ctrl Pts',(-37.9028280459028,31.3070187859893,7.85280993826337));
#29408=CARTESIAN_POINT('Ctrl Pts',(-39.0706571061612,33.7983874965128,7.7556177539892));
#29409=CARTESIAN_POINT('Ctrl Pts',(-39.0784090602678,35.0020440536087,7.70842344717747));
#29410=CARTESIAN_POINT('Origin',(35.,-35.,10.2084234471775));
#29411=CARTESIAN_POINT('',(30.9212701195312,-34.9980516557686,0.791576552822542));
#29412=CARTESIAN_POINT('',(30.9328376585755,-35.000159236028,0.708423447177449));
#29413=CARTESIAN_POINT('',(30.9265,-34.9999999999999,10.2084234471775));
#29414=CARTESIAN_POINT('',(36.0520713770612,-38.9352951690526,0.));
#29415=CARTESIAN_POINT('Ctrl Pts',(30.9328376585755,-35.000159236028,0.708423447177449));
#29416=CARTESIAN_POINT('Ctrl Pts',(30.9332830863018,-34.31144230346,0.681615801254637));
#29417=CARTESIAN_POINT('Ctrl Pts',(31.423729341332,-32.2777627653814,0.602474779547741));
#29418=CARTESIAN_POINT('Ctrl Pts',(34.6204730639081,-30.2191415991965,0.471000382056761));
#29419=CARTESIAN_POINT('Ctrl Pts',(38.7813009234074,-32.0442168078902,0.314000254704507));
#29420=CARTESIAN_POINT('Ctrl Pts',(39.5450614875854,-36.5273565705141,0.157000127352254));
#29421=CARTESIAN_POINT('Ctrl Pts',(37.3460763064866,-38.5893527455387,0.0523333757840845));
#29422=CARTESIAN_POINT('Ctrl Pts',(36.0520713770612,-38.9352951690526,0.));
#29423=CARTESIAN_POINT('',(33.9452809380949,-38.9416008127442,2.82508323912273E-15));
#29424=CARTESIAN_POINT('Origin',(35.,-35.,0.));
#29425=CARTESIAN_POINT('Ctrl Pts',(30.9212701195312,-34.9980516557686,0.791576552822542));
#29426=CARTESIAN_POINT('Ctrl Pts',(30.9205868455494,-34.8825847167923,0.787049082480475));
#29427=CARTESIAN_POINT('Ctrl Pts',(30.9769555821544,-33.4331078068366,0.730188236354323));
#29428=CARTESIAN_POINT('Ctrl Pts',(32.704491289799,-30.7882324000235,0.620994014444087));
#29429=CARTESIAN_POINT('Ctrl Pts',(37.2468174060219,-30.7615623188695,0.463993887091833));
#29430=CARTESIAN_POINT('Ctrl Pts',(39.7742801854456,-34.536716632844,0.306993759739581));
#29431=CARTESIAN_POINT('Ctrl Pts',(38.0469263053514,-38.6626279973746,0.152329130708969));
#29432=CARTESIAN_POINT('Ctrl Pts',(35.1775586628442,-39.2670009745688,0.0499978774624438));
#29433=CARTESIAN_POINT('Ctrl Pts',(33.94526862329,-38.9416301412996,2.47469145869816E-15));
#29434=CARTESIAN_POINT('Origin',(35.,-35.,10.2084234471775));
#29435=CARTESIAN_POINT('',(30.9325671258701,-34.9990828432724,1.79157655282254));
#29436=CARTESIAN_POINT('',(30.9221796304986,-35.0024921194124,1.70842344717745));
#29437=CARTESIAN_POINT('',(30.9265,-34.9999999999999,10.2084234471775));
#29438=CARTESIAN_POINT('Ctrl Pts',(30.9221796304986,-35.0024921194124,1.70842344717745));
#29439=CARTESIAN_POINT('Ctrl Pts',(30.9307245358113,-33.8250296189916,1.66228272262581));
#29440=CARTESIAN_POINT('Ctrl Pts',(32.0812070745664,-31.2974912653129,1.56380862229009));
#29441=CARTESIAN_POINT('Ctrl Pts',(36.3504798077544,-30.397209980765,1.41300114617028));
#29442=CARTESIAN_POINT('Ctrl Pts',(39.5841211762074,-33.5872716944053,1.25600101881803));
#29443=CARTESIAN_POINT('Ctrl Pts',(38.7070435276578,-38.0442501505519,1.09900089146578));
#29444=CARTESIAN_POINT('Ctrl Pts',(34.5060129254091,-39.7711992366401,0.942000764113522));
#29445=CARTESIAN_POINT('Ctrl Pts',(31.3893173078737,-37.6557923296961,0.811808282684079));
#29446=CARTESIAN_POINT('Ctrl Pts',(30.9324135307783,-35.6559423817109,0.733949177038721));
#29447=CARTESIAN_POINT('Ctrl Pts',(30.9328376585755,-35.000159236028,0.708423447177449));
#29448=CARTESIAN_POINT('Ctrl Pts',(30.9325671258701,-34.9990828432724,1.79157655282254));
#29449=CARTESIAN_POINT('Ctrl Pts',(30.931305764143,-34.3862015569849,1.76771600385165));
#29450=CARTESIAN_POINT('Ctrl Pts',(31.3469048767902,-32.4307110971121,1.69152207909667));
#29451=CARTESIAN_POINT('Ctrl Pts',(34.3564138261785,-30.2465374145616,1.56299477855761));
#29452=CARTESIAN_POINT('Ctrl Pts',(38.6097341605507,-31.8409675209513,1.40599465120535));
#29453=CARTESIAN_POINT('Ctrl Pts',(39.6261694334752,-36.2681500029269,1.2489945238531));
#29454=CARTESIAN_POINT('Ctrl Pts',(36.4942778376799,-39.5581346787212,1.09199439650085));
#29455=CARTESIAN_POINT('Ctrl Pts',(32.1514014998571,-38.7838588891191,0.939521739490662));
#29456=CARTESIAN_POINT('Ctrl Pts',(30.928484861737,-36.2172758912295,0.839382458264559));
#29457=CARTESIAN_POINT('Ctrl Pts',(30.9212701195312,-34.9980516557686,0.791576552822542));
#29458=CARTESIAN_POINT('Origin',(35.,-35.,10.2084234471775));
#29459=CARTESIAN_POINT('',(30.9241574748343,-35.0032082359637,2.79157655282255));
#29460=CARTESIAN_POINT('',(30.9271225309901,-34.9964941798068,2.70842344717745));
#29461=CARTESIAN_POINT('',(30.9265,-34.9999999999999,10.2084234471775));
#29462=CARTESIAN_POINT('Ctrl Pts',(30.9271225309901,-34.9964941798068,2.70842344717745));
#29463=CARTESIAN_POINT('Ctrl Pts',(30.9241960153079,-34.6601099513618,2.69528301978107));
#29464=CARTESIAN_POINT('Ctrl Pts',(31.1149287231428,-32.9873057374911,2.62980921660061));
#29465=CARTESIAN_POINT('Ctrl Pts',(33.4155015345008,-30.4724167149005,2.51200203763606));
#29466=CARTESIAN_POINT('Ctrl Pts',(37.9022802570419,-31.180783908422,2.3550019102838));
#29467=CARTESIAN_POINT('Ctrl Pts',(39.7865571243079,-35.3138779969793,2.19800178293155));
#29468=CARTESIAN_POINT('Ctrl Pts',(37.3786808989502,-39.1655163148135,2.04100165557929));
#29469=CARTESIAN_POINT('Ctrl Pts',(32.8378215103303,-39.2818928860424,1.88400152822704));
#29470=CARTESIAN_POINT('Ctrl Pts',(31.0005092531499,-36.6528810868796,1.77314212542643));
#29471=CARTESIAN_POINT('Ctrl Pts',(30.9210327993872,-35.1605220306295,1.7146160984099));
#29472=CARTESIAN_POINT('Ctrl Pts',(30.9221796304986,-35.0024921194124,1.70842344717745));
#29473=CARTESIAN_POINT('Ctrl Pts',(30.9241574748343,-35.0032082359637,2.79157655282255));
#29474=CARTESIAN_POINT('Ctrl Pts',(30.9336811658698,-33.8995582265895,2.74838292522282));
#29475=CARTESIAN_POINT('Ctrl Pts',(31.9624565435572,-31.4430713953983,2.65285592183902));
#29476=CARTESIAN_POINT('Ctrl Pts',(36.092848009894,-30.329313184686,2.50499554267113));
#29477=CARTESIAN_POINT('Ctrl Pts',(39.4985856069267,-33.3349593710879,2.34799541531888));
#29478=CARTESIAN_POINT('Ctrl Pts',(38.8703983056154,-37.8336637277424,2.19099528796662));
#29479=CARTESIAN_POINT('Ctrl Pts',(34.7715877673847,-39.7913941019012,2.03399516061437));
#29480=CARTESIAN_POINT('Ctrl Pts',(31.4693971488356,-37.8080759514836,1.90085558223301));
#29481=CARTESIAN_POINT('Ctrl Pts',(30.9340723106019,-35.73043494849,1.82004937963573));
#29482=CARTESIAN_POINT('Ctrl Pts',(30.9325671258701,-34.9990828432724,1.79157655282254));
#29483=CARTESIAN_POINT('Origin',(35.,-35.,10.2084234471775));
#29484=CARTESIAN_POINT('',(30.9249291606556,-34.9966356401017,3.79157655282255));
#29485=CARTESIAN_POINT('',(30.9312887064921,-35.0023266137465,3.70842344717745));
#29486=CARTESIAN_POINT('',(30.9265,-34.9999999999999,10.2084234471775));
#29487=CARTESIAN_POINT('Ctrl Pts',(30.9312887064921,-35.0023266137465,3.70842344717745));
#29488=CARTESIAN_POINT('Ctrl Pts',(30.9357302778565,-34.1688705201733,3.67594994115225));
#29489=CARTESIAN_POINT('Ctrl Pts',(31.5875549849899,-31.9858615080358,3.59114305934295));
#29490=CARTESIAN_POINT('Ctrl Pts',(35.1332185405061,-30.2050132515957,3.45400280174957));
#29491=CARTESIAN_POINT('Ctrl Pts',(39.0728865166754,-32.4659833342563,3.29700267439732));
#29492=CARTESIAN_POINT('Ctrl Pts',(39.3603580902194,-36.9992304591644,3.14000254704507));
#29493=CARTESIAN_POINT('Ctrl Pts',(35.7378547119649,-39.73974847612,2.98300241969282));
#29494=CARTESIAN_POINT('Ctrl Pts',(31.8122797042457,-38.3564424059702,2.83914271973694));
#29495=CARTESIAN_POINT('Ctrl Pts',(30.9358512256228,-35.9998017059771,2.74761639556516));
#29496=CARTESIAN_POINT('Ctrl Pts',(30.9271225309901,-34.9964941798068,2.70842344717745));
#29497=CARTESIAN_POINT('Ctrl Pts',(30.9249291606557,-34.9966356401017,3.79157655282255));
#29498=CARTESIAN_POINT('Ctrl Pts',(30.9226270376253,-34.7360558424623,3.78138322237808));
#29499=CARTESIAN_POINT('Ctrl Pts',(31.0631421094905,-33.1401098702831,3.71885651614953));
#29500=CARTESIAN_POINT('Ctrl Pts',(33.1665616130745,-30.567378187653,3.6039964341369));
#29501=CARTESIAN_POINT('Ctrl Pts',(37.6857487228281,-31.0255332130596,3.44699630678465));
#29502=CARTESIAN_POINT('Ctrl Pts',(39.7965991870786,-35.0476307336073,3.28999617943239));
#29503=CARTESIAN_POINT('Ctrl Pts',(37.606293143399,-39.0270173223719,3.13299605208014));
#29504=CARTESIAN_POINT('Ctrl Pts',(33.0788990351993,-39.3953388367078,2.97599592472789));
#29505=CARTESIAN_POINT('Ctrl Pts',(31.0458059595307,-36.8053217637502,2.86218942497536));
#29506=CARTESIAN_POINT('Ctrl Pts',(30.9221422669741,-35.2367399796465,2.80071630100691));
#29507=CARTESIAN_POINT('Ctrl Pts',(30.9241574748343,-35.0032082359637,2.79157655282255));
#29508=CARTESIAN_POINT('Origin',(35.,-35.,10.2084234471775));
#29509=CARTESIAN_POINT('',(30.9323405716502,-35.0013188445396,4.79157655282255));
#29510=CARTESIAN_POINT('',(30.9200767953891,-35.0002389671868,4.70842344717745));
#29511=CARTESIAN_POINT('',(30.9265,-34.9999999999999,10.2084234471775));
#29512=CARTESIAN_POINT('Ctrl Pts',(30.9200767953891,-35.0002389671868,4.70842344717745));
#29513=CARTESIAN_POINT('Ctrl Pts',(30.9212224901389,-33.6800002558017,4.65661686252342));
#29514=CARTESIAN_POINT('Ctrl Pts',(32.3294140201846,-31.0239948489069,4.5524769020853));
#29515=CARTESIAN_POINT('Ctrl Pts',(36.8334388902368,-30.5673769708228,4.39600356586309));
#29516=CARTESIAN_POINT('Ctrl Pts',(39.7085649985197,-34.0839974156347,4.23900343851085));
#29517=CARTESIAN_POINT('Ctrl Pts',(38.3614757008081,-38.4220061649164,4.08200331115859));
#29518=CARTESIAN_POINT('Ctrl Pts',(34.0001188933562,-39.6914691574817,3.92500318380634));
#29519=CARTESIAN_POINT('Ctrl Pts',(31.2520059142893,-37.3616157091949,3.80047656247929));
#29520=CARTESIAN_POINT('Ctrl Pts',(30.9285723681714,-35.5120445806103,3.72828331693633));
#29521=CARTESIAN_POINT('Ctrl Pts',(30.9312887064921,-35.0023266137465,3.70842344717745));
#29522=CARTESIAN_POINT('Ctrl Pts',(30.9323405716502,-35.0013188445396,4.79157655282255));
#29523=CARTESIAN_POINT('Ctrl Pts',(30.9345932718416,-34.2430104629966,4.76205014374926));
#29524=CARTESIAN_POINT('Ctrl Pts',(31.4994189252081,-32.1375393584237,4.68019035889188));
#29525=CARTESIAN_POINT('Ctrl Pts',(34.8667814960507,-30.2050145678827,4.54599719825042));
#29526=CARTESIAN_POINT('Ctrl Pts',(38.9259067064028,-32.2437545499559,4.38899707089817));
#29527=CARTESIAN_POINT('Ctrl Pts',(39.4646337070995,-36.7540462662356,4.23199694354592));
#29528=CARTESIAN_POINT('Ctrl Pts',(35.9998808321606,-39.6914678695931,4.07499681619366));
#29529=CARTESIAN_POINT('Ctrl Pts',(31.921688934453,-38.5044258734202,3.92819001928587));
#29530=CARTESIAN_POINT('Ctrl Pts',(30.934446321843,-36.0738934163447,3.83371659816217));
#29531=CARTESIAN_POINT('Ctrl Pts',(30.9249291606557,-34.9966356401017,3.79157655282255));
#29532=CARTESIAN_POINT('Origin',(35.,-35.,10.2084234471775));
#29533=CARTESIAN_POINT('',(30.9207984791111,-35.0015161195221,5.79157655282255));
#29534=CARTESIAN_POINT('',(30.93077657492,-34.9973709027416,5.70842344717745));
#29535=CARTESIAN_POINT('',(30.9265,-34.9999999999999,10.2084234471775));
#29536=CARTESIAN_POINT('Ctrl Pts',(30.93077657492,-34.9973709027416,5.70842344717745));
#29537=CARTESIAN_POINT('Ctrl Pts',(30.9278458307013,-34.5148468886989,5.68961715967867));
#29538=CARTESIAN_POINT('Ctrl Pts',(31.2287023543687,-32.6931085261371,5.61847749639581));
#29539=CARTESIAN_POINT('Ctrl Pts',(33.9071516901285,-30.3293119021379,5.49500445732887));
#29540=CARTESIAN_POINT('Ctrl Pts',(38.292857772379,-31.5119155853487,5.33800432997662));
#29541=CARTESIAN_POINT('Ctrl Pts',(39.7258267066312,-35.8223180909381,5.18100420262436));
#29542=CARTESIAN_POINT('Ctrl Pts',(36.9211014921746,-39.3953400433581,5.02400407527211));
#29543=CARTESIAN_POINT('Ctrl Pts',(32.3937061411281,-39.0270184278339,4.86700394791986));
#29544=CARTESIAN_POINT('Ctrl Pts',(30.9261524552523,-36.3607410495406,4.76181040522164));
#29545=CARTESIAN_POINT('Ctrl Pts',(30.9200651454832,-35.0136637093765,4.7089502383075));
#29546=CARTESIAN_POINT('Ctrl Pts',(30.9200767953891,-35.0002389671868,4.70842344717745));
#29547=CARTESIAN_POINT('Ctrl Pts',(30.9207984791111,-35.0015161195221,5.79157655282254));
#29548=CARTESIAN_POINT('Ctrl Pts',(30.9268330150145,-33.7557922534996,5.74271706512043));
#29549=CARTESIAN_POINT('Ctrl Pts',(32.1969979306855,-31.1651111648659,5.64152420163423));
#29550=CARTESIAN_POINT('Ctrl Pts',(36.584498029893,-30.4724179566463,5.48799796236395));
#29551=CARTESIAN_POINT('Ctrl Pts',(39.6504412814188,-33.8239776163473,5.33099783501169));
#29552=CARTESIAN_POINT('Ctrl Pts',(38.5462890493217,-38.2300876270061,5.17399770765944));
#29553=CARTESIAN_POINT('Ctrl Pts',(34.2621454906851,-39.7397471751372,5.01699758030718));
#29554=CARTESIAN_POINT('Ctrl Pts',(31.3209131735827,-37.5146284338107,4.88952386202822));
#29555=CARTESIAN_POINT('Ctrl Pts',(30.9306005274021,-35.5870559713077,4.81438351953334));
#29556=CARTESIAN_POINT('Ctrl Pts',(30.9323405716502,-35.0013188445396,4.79157655282255));
#29557=CARTESIAN_POINT('Origin',(35.,-35.,10.2084234471775));
#29558=CARTESIAN_POINT('',(30.9290344477858,-34.9967444478932,6.79157655282255));
#29559=CARTESIAN_POINT('',(30.9278856911952,-35.003454802609,6.70842344717745));
#29560=CARTESIAN_POINT('',(30.9265,-34.9999999999999,10.2084234471775));
#29561=CARTESIAN_POINT('Ctrl Pts',(30.9278856911952,-35.003454802609,6.70842344717745));
#29562=CARTESIAN_POINT('Ctrl Pts',(30.9361134364198,-34.0266504850423,6.67028408104985));
#29563=CARTESIAN_POINT('Ctrl Pts',(31.7747975664789,-31.6968179913154,6.57981133913816));
#29564=CARTESIAN_POINT('Ctrl Pts',(35.6435863532121,-30.2465360930486,6.43700522144239));
#29565=CARTESIAN_POINT('Ctrl Pts',(39.3197968978512,-32.9145734850341,6.28000509409014));
#29566=CARTESIAN_POINT('Ctrl Pts',(39.1224045728929,-37.4526371600059,6.12300496673789));
#29567=CARTESIAN_POINT('Ctrl Pts',(35.2284122950338,-39.7913954197145,5.96600483938562));
#29568=CARTESIAN_POINT('Ctrl Pts',(31.6205774983358,-38.0681716417432,5.82781099953216));
#29569=CARTESIAN_POINT('Ctrl Pts',(30.9360013871094,-35.857595187819,5.74195053546276));
#29570=CARTESIAN_POINT('Ctrl Pts',(30.93077657492,-34.9973709027416,5.70842344717745));
#29571=CARTESIAN_POINT('Ctrl Pts',(30.9290344477858,-34.9967444478932,6.79157655282255));
#29572=CARTESIAN_POINT('Ctrl Pts',(30.9258715916941,-34.5902727617055,6.77571736227569));
#29573=CARTESIAN_POINT('Ctrl Pts',(31.1671176609215,-32.8461587416485,6.70752479594475));
#29574=CARTESIAN_POINT('Ctrl Pts',(33.6495206016122,-30.3972113452741,6.58699885382972));
#29575=CARTESIAN_POINT('Ctrl Pts',(38.09410244091,-31.3344607296745,6.42999872647747));
#29576=CARTESIAN_POINT('Ctrl Pts',(39.7641960678496,-35.558661561786,6.27299859912521));
#29577=CARTESIAN_POINT('Ctrl Pts',(37.1621778889461,-39.2818916953666,6.11599847177296));
#29578=CARTESIAN_POINT('Ctrl Pts',(32.6213197580022,-39.1655151793351,5.95899834442071));
#29579=CARTESIAN_POINT('Ctrl Pts',(30.962791139069,-36.5125331378606,5.85085770477057));
#29580=CARTESIAN_POINT('Ctrl Pts',(30.920369426263,-35.0900865383931,5.79505044090451));
#29581=CARTESIAN_POINT('Ctrl Pts',(30.9207984791111,-35.0015161195221,5.79157655282254));
#29582=CARTESIAN_POINT('Origin',(35.,-35.,10.2084234471775));
#29583=CARTESIAN_POINT('',(30.9308748007386,-35.0040807474719,7.79157655282254));
#29584=CARTESIAN_POINT('',(30.9215903995924,-34.9979557257256,7.70842344717745));
#29585=CARTESIAN_POINT('',(30.9265,-34.9999999999999,10.2084234471775));
#29586=CARTESIAN_POINT('',(33.9479286229388,-38.9352951690526,8.));
#29587=CARTESIAN_POINT('Ctrl Pts',(33.9479286229388,-38.9352951690526,8.));
#29588=CARTESIAN_POINT('Ctrl Pts',(32.6539236935135,-38.5893527455387,7.94766662421592));
#29589=CARTESIAN_POINT('Ctrl Pts',(31.1943052713303,-37.2206748258175,7.87819214182343));
#29590=CARTESIAN_POINT('Ctrl Pts',(30.9278727863252,-35.4436627970733,7.80871765943094));
#29591=CARTESIAN_POINT('Ctrl Pts',(30.9308748007386,-35.0040807474719,7.79157655282254));
#29592=CARTESIAN_POINT('',(36.0547201762178,-38.9416007819636,8.));
#29593=CARTESIAN_POINT('Origin',(35.,-35.,8.));
#29594=CARTESIAN_POINT('Ctrl Pts',(36.0547325237759,-38.9416301760088,8.));
#29595=CARTESIAN_POINT('Ctrl Pts',(34.822443357586,-39.2670001819919,7.95000212253756));
#29596=CARTESIAN_POINT('Ctrl Pts',(32.0971704836176,-38.6929832307492,7.85280993826338));
#29597=CARTESIAN_POINT('Ctrl Pts',(30.9293421550372,-36.2016127302822,7.75561775398919));
#29598=CARTESIAN_POINT('Ctrl Pts',(30.9215903995924,-34.9979557257256,7.70842344717745));
#29599=CARTESIAN_POINT('Origin',(-35.,-35.,10.2084234471775));
#29600=CARTESIAN_POINT('',(-39.0787307957508,-34.998051746757,0.791576552822544));
#29601=CARTESIAN_POINT('',(-39.0671620604938,-35.0001591466914,0.708423447177451));
#29602=CARTESIAN_POINT('',(-39.0735,-34.9999999999999,10.2084234471775));
#29603=CARTESIAN_POINT('',(-33.9479286229388,-38.9352951690526,0.));
#29604=CARTESIAN_POINT('Ctrl Pts',(-39.0671620604938,-35.0001591466914,
0.708423447177451));
#29605=CARTESIAN_POINT('Ctrl Pts',(-39.0667166230717,-34.3114421978074,
0.681615801254639));
#29606=CARTESIAN_POINT('Ctrl Pts',(-38.5762703689089,-32.2777626699106,
0.602474779547742));
#29607=CARTESIAN_POINT('Ctrl Pts',(-35.3795268907121,-30.2191428513895,
0.471000382056761));
#29608=CARTESIAN_POINT('Ctrl Pts',(-31.2186995847689,-32.0442153857854,
0.314000254704507));
#29609=CARTESIAN_POINT('Ctrl Pts',(-30.4549379250093,-36.5273603729133,
0.157000127352253));
#29610=CARTESIAN_POINT('Ctrl Pts',(-32.6539236935135,-38.5893527455387,
0.0523333757840845));
#29611=CARTESIAN_POINT('Ctrl Pts',(-33.9479286229388,-38.9352951690526,
0.));
#29612=CARTESIAN_POINT('',(-36.0547200012553,-38.9416007855471,4.26113251110999E-15));
#29613=CARTESIAN_POINT('Origin',(-35.,-35.,0.));
#29614=CARTESIAN_POINT('Ctrl Pts',(-39.0787307957508,-34.9980517467571,
0.791576552822544));
#29615=CARTESIAN_POINT('Ctrl Pts',(-39.0794140710738,-34.8825847789344,
0.787049082480477));
#29616=CARTESIAN_POINT('Ctrl Pts',(-39.0230453421645,-33.4331074898667,
0.730188236354326));
#29617=CARTESIAN_POINT('Ctrl Pts',(-37.2955094371433,-30.7882309135474,
0.620994014444089));
#29618=CARTESIAN_POINT('Ctrl Pts',(-32.7531816644513,-30.7615622313046,
0.463993887091836));
#29619=CARTESIAN_POINT('Ctrl Pts',(-30.2257195673566,-34.5367150123096,
0.306993759739581));
#29620=CARTESIAN_POINT('Ctrl Pts',(-31.9530712365814,-38.6626312798268,
0.152329130708972));
#29621=CARTESIAN_POINT('Ctrl Pts',(-34.8224430395506,-39.2670003060384,
0.0499978774624443));
#29622=CARTESIAN_POINT('Ctrl Pts',(-36.0547323436802,-38.9416301693299,
2.36437388764776E-15));
#29623=CARTESIAN_POINT('Origin',(-35.,-35.,10.2084234471775));
#29624=CARTESIAN_POINT('',(-39.0674338139571,-34.9990828447087,1.79157655282254));
#29625=CARTESIAN_POINT('',(-39.0778200867196,-35.0024921203811,1.70842344717745));
#29626=CARTESIAN_POINT('',(-39.0735,-34.9999999999999,10.2084234471775));
#29627=CARTESIAN_POINT('Ctrl Pts',(-39.0778200867196,-35.0024921203811,
1.70842344717745));
#29628=CARTESIAN_POINT('Ctrl Pts',(-39.0692751810275,-33.8250296994275,
1.66228272262581));
#29629=CARTESIAN_POINT('Ctrl Pts',(-37.9187927175433,-31.297491510544,1.56380862229009));
#29630=CARTESIAN_POINT('Ctrl Pts',(-33.6495202958365,-30.3972103260493,
1.41300114617028));
#29631=CARTESIAN_POINT('Ctrl Pts',(-30.4158791260905,-33.5872717453,1.25600101881803));
#29632=CARTESIAN_POINT('Ctrl Pts',(-31.2929567559004,-38.0442500262742,
1.09900089146578));
#29633=CARTESIAN_POINT('Ctrl Pts',(-35.4939870016774,-39.7711987453336,
0.942000764113521));
#29634=CARTESIAN_POINT('Ctrl Pts',(-38.6106824762136,-37.6557923579424,
0.81180828268408));
#29635=CARTESIAN_POINT('Ctrl Pts',(-39.0675861975231,-35.6559423079101,
0.733949177038723));
#29636=CARTESIAN_POINT('Ctrl Pts',(-39.0671620604938,-35.0001591466914,
0.708423447177451));
#29637=CARTESIAN_POINT('Ctrl Pts',(-39.0674338139571,-34.9990828447087,
1.79157655282254));
#29638=CARTESIAN_POINT('Ctrl Pts',(-39.0686951758822,-34.3862014174905,
1.76771600385165));
#29639=CARTESIAN_POINT('Ctrl Pts',(-38.6530959670617,-32.4307105068614,
1.69152207909667));
#29640=CARTESIAN_POINT('Ctrl Pts',(-35.6435863248602,-30.2465363019221,
1.56299477855761));
#29641=CARTESIAN_POINT('Ctrl Pts',(-31.3902650003177,-31.8409668168855,
1.40599465120536));
#29642=CARTESIAN_POINT('Ctrl Pts',(-30.3738295074692,-36.2681502477922,
1.2489945238531));
#29643=CARTESIAN_POINT('Ctrl Pts',(-33.5057217955833,-39.5581358207848,
1.09199439650085));
#29644=CARTESIAN_POINT('Ctrl Pts',(-37.8485992014502,-38.7838596097918,
0.939521739490664));
#29645=CARTESIAN_POINT('Ctrl Pts',(-39.0715160393823,-36.2172762868091,
0.839382458264562));
#29646=CARTESIAN_POINT('Ctrl Pts',(-39.0787307957508,-34.9980517467571,
0.791576552822544));
#29647=CARTESIAN_POINT('Origin',(-35.,-35.,10.2084234471775));
#29648=CARTESIAN_POINT('',(-39.0758434671966,-35.0032082366984,2.79157655282255));
#29649=CARTESIAN_POINT('',(-39.0728771860086,-34.996494180098,2.70842344717745));
#29650=CARTESIAN_POINT('',(-39.0735,-34.9999999999999,10.2084234471775));
#29651=CARTESIAN_POINT('Ctrl Pts',(-39.0728771860086,-34.996494180098,2.70842344717745));
#29652=CARTESIAN_POINT('Ctrl Pts',(-39.075803701489,-34.6601099750312,2.69528301978107));
#29653=CARTESIAN_POINT('Ctrl Pts',(-38.8850710069041,-32.9873058773963,
2.62980921660061));
#29654=CARTESIAN_POINT('Ctrl Pts',(-36.5844983552314,-30.4724170292356,
2.51200203763606));
#29655=CARTESIAN_POINT('Ctrl Pts',(-32.0977199449364,-31.1807841743797,
2.3550019102838));
#29656=CARTESIAN_POINT('Ctrl Pts',(-30.2134432077683,-35.3138779741053,
2.19800178293155));
#29657=CARTESIAN_POINT('Ctrl Pts',(-32.621319267345,-39.1655160273689,2.04100165557929));
#29658=CARTESIAN_POINT('Ctrl Pts',(-37.1621783376115,-39.2818925846584,
1.88400152822705));
#29659=CARTESIAN_POINT('Ctrl Pts',(-38.9994904706692,-36.6528809760016,
1.77314212542643));
#29660=CARTESIAN_POINT('Ctrl Pts',(-39.0789669178819,-35.1605220209328,
1.7146160984099));
#29661=CARTESIAN_POINT('Ctrl Pts',(-39.0778200867196,-35.0024921203811,
1.70842344717745));
#29662=CARTESIAN_POINT('Ctrl Pts',(-39.0758434671966,-35.0032082366984,
2.79157655282255));
#29663=CARTESIAN_POINT('Ctrl Pts',(-39.0663197739578,-33.8995579722718,
2.74838292522283));
#29664=CARTESIAN_POINT('Ctrl Pts',(-38.037544158487,-31.4430705734335,2.65285592183902));
#29665=CARTESIAN_POINT('Ctrl Pts',(-33.9071517375455,-30.3293121048675,
2.50499554267113));
#29666=CARTESIAN_POINT('Ctrl Pts',(-30.5014133532831,-33.3349589868354,
2.34799541531887));
#29667=CARTESIAN_POINT('Ctrl Pts',(-31.12960079995,-37.8336643815683,2.19099528796663));
#29668=CARTESIAN_POINT('Ctrl Pts',(-35.2284122851668,-39.7913952114128,
2.03399516061437));
#29669=CARTESIAN_POINT('Ctrl Pts',(-38.5306036675732,-37.8080765974554,
1.90085558223301));
#29670=CARTESIAN_POINT('Ctrl Pts',(-39.0659286289889,-35.7304351180991,
1.82004937963574));
#29671=CARTESIAN_POINT('Ctrl Pts',(-39.0674338139571,-34.9990828447087,
1.79157655282254));
#29672=CARTESIAN_POINT('Origin',(-35.,-35.,10.2084234471775));
#29673=CARTESIAN_POINT('',(-39.0750717811968,-34.9966356393236,3.79157655282255));
#29674=CARTESIAN_POINT('',(-39.0687110107696,-35.0023266135852,3.70842344717746));
#29675=CARTESIAN_POINT('',(-39.0735,-34.9999999999999,10.2084234471775));
#29676=CARTESIAN_POINT('Ctrl Pts',(-39.0687110107696,-35.0023266135852,
3.70842344717746));
#29677=CARTESIAN_POINT('Ctrl Pts',(-39.0642694397141,-34.16887057793,3.67594994115225));
#29678=CARTESIAN_POINT('Ctrl Pts',(-38.4124447778773,-31.9858617174929,
3.59114305934296));
#29679=CARTESIAN_POINT('Ctrl Pts',(-34.8667814687478,-30.2050135847982,
3.45400280174957));
#29680=CARTESIAN_POINT('Ctrl Pts',(-30.9271137663599,-32.4659835103585,
3.29700267439732));
#29681=CARTESIAN_POINT('Ctrl Pts',(-30.6396422127733,-36.9992303202149,
3.14000254704507));
#29682=CARTESIAN_POINT('Ctrl Pts',(-34.2621453393335,-39.7397481467912,
2.98300241969281));
#29683=CARTESIAN_POINT('Ctrl Pts',(-38.1877200741971,-38.356442172659,2.83914271973695));
#29684=CARTESIAN_POINT('Ctrl Pts',(-39.0641484919776,-35.9998016365399,
2.74761639556516));
#29685=CARTESIAN_POINT('Ctrl Pts',(-39.0728771860086,-34.996494180098,2.70842344717745));
#29686=CARTESIAN_POINT('Ctrl Pts',(-39.0750717811968,-34.9966356393236,
3.79157655282255));
#29687=CARTESIAN_POINT('Ctrl Pts',(-39.0773739047593,-34.7360557814575,
3.78138322237809));
#29688=CARTESIAN_POINT('Ctrl Pts',(-38.9368588004177,-33.1401094404144,
3.71885651614954));
#29689=CARTESIAN_POINT('Ctrl Pts',(-36.8334388106793,-30.5673771631648,
3.6039964341369));
#29690=CARTESIAN_POINT('Ctrl Pts',(-32.3142506564274,-31.0255322944533,
3.44699630678465));
#29691=CARTESIAN_POINT('Ctrl Pts',(-30.2033997043049,-35.0476307446275,
3.28999617943239));
#29692=CARTESIAN_POINT('Ctrl Pts',(-32.3937062542216,-39.0270182530956,
3.13299605208014));
#29693=CARTESIAN_POINT('Ctrl Pts',(-36.9211014088136,-39.3953398526252,
2.97599592472789));
#29694=CARTESIAN_POINT('Ctrl Pts',(-38.9541949543872,-36.8053221809578,
2.86218942497536));
#29695=CARTESIAN_POINT('Ctrl Pts',(-39.077858675523,-35.2367400343503,2.80071630100691));
#29696=CARTESIAN_POINT('Ctrl Pts',(-39.0758434671966,-35.0032082366984,
2.79157655282255));
#29697=CARTESIAN_POINT('Origin',(-35.,-35.,10.2084234471775));
#29698=CARTESIAN_POINT('',(-39.0676603684793,-35.0013188448613,4.79157655282255));
#29699=CARTESIAN_POINT('',(-39.0799229210932,-35.0002389671693,4.70842344717745));
#29700=CARTESIAN_POINT('',(-39.0735,-34.9999999999999,10.2084234471775));
#29701=CARTESIAN_POINT('Ctrl Pts',(-39.0799229210932,-35.0002389671693,
4.70842344717745));
#29702=CARTESIAN_POINT('Ctrl Pts',(-39.0787772264229,-33.680000347528,4.65661686252342));
#29703=CARTESIAN_POINT('Ctrl Pts',(-37.6705857942339,-31.023995125205,4.5524769020853));
#29704=CARTESIAN_POINT('Ctrl Pts',(-33.1665612371704,-30.5673772788489,
4.39600356586309));
#29705=CARTESIAN_POINT('Ctrl Pts',(-30.291435328683,-34.0839974792893,4.23900343851084));
#29706=CARTESIAN_POINT('Ctrl Pts',(-31.6385245327839,-38.4220059271175,
4.08200331115859));
#29707=CARTESIAN_POINT('Ctrl Pts',(-35.9998810371616,-39.6914688314679,
3.92500318380634));
#29708=CARTESIAN_POINT('Ctrl Pts',(-38.7479938252585,-37.361615545083,3.80047656247929));
#29709=CARTESIAN_POINT('Ctrl Pts',(-39.0714273489013,-35.5120445450279,
3.72828331693633));
#29710=CARTESIAN_POINT('Ctrl Pts',(-39.0687110107696,-35.0023266135852,
3.70842344717746));
#29711=CARTESIAN_POINT('Ctrl Pts',(-39.0676603684793,-35.0013188448613,
4.79157655282255));
#29712=CARTESIAN_POINT('Ctrl Pts',(-39.065407667772,-34.2430102880461,4.76205014374926));
#29713=CARTESIAN_POINT('Ctrl Pts',(-38.5005818838826,-32.1375386968076,
4.68019035889189));
#29714=CARTESIAN_POINT('Ctrl Pts',(-35.1332185347277,-30.2050134596587,
4.54599719825043));
#29715=CARTESIAN_POINT('Ctrl Pts',(-31.0740923862265,-32.2437539129077,
4.38899707089817));
#29716=CARTESIAN_POINT('Ctrl Pts',(-30.535365261007,-36.7540466716456,4.23199694354592));
#29717=CARTESIAN_POINT('Ctrl Pts',(-34.0001189367432,-39.6914689539076,
4.07499681619366));
#29718=CARTESIAN_POINT('Ctrl Pts',(-38.0783117770221,-38.5044266833838,
3.92819001928587));
#29719=CARTESIAN_POINT('Ctrl Pts',(-39.0655546178097,-36.0738936645484,
3.83371659816217));
#29720=CARTESIAN_POINT('Ctrl Pts',(-39.0750717811968,-34.9966356393236,
3.79157655282255));
#29721=CARTESIAN_POINT('Origin',(-35.,-35.,10.2084234471775));
#29722=CARTESIAN_POINT('',(-39.0792024631389,-35.0015161209354,5.79157655282255));
#29723=CARTESIAN_POINT('',(-39.0692231423099,-34.9973709029543,5.70842344717745));
#29724=CARTESIAN_POINT('',(-39.0735,-34.9999999999999,10.2084234471775));
#29725=CARTESIAN_POINT('Ctrl Pts',(-39.0692231423099,-34.9973709029543,
5.70842344717745));
#29726=CARTESIAN_POINT('Ctrl Pts',(-39.072153886322,-34.5148469224124,5.68961715967868));
#29727=CARTESIAN_POINT('Ctrl Pts',(-38.7712973835496,-32.6931086863282,
5.61847749639582));
#29728=CARTESIAN_POINT('Ctrl Pts',(-36.0928482339355,-30.3293122267992,
5.49500445732888));
#29729=CARTESIAN_POINT('Ctrl Pts',(-31.7071424564414,-31.5119158276916,
5.33800432997661));
#29730=CARTESIAN_POINT('Ctrl Pts',(-30.2741736217725,-35.8223180338192,
5.18100420262437));
#29731=CARTESIAN_POINT('Ctrl Pts',(-33.0788986413239,-39.395339737909,5.02400407527211));
#29732=CARTESIAN_POINT('Ctrl Pts',(-37.6062936777584,-39.0270181479993,
4.86700394791986));
#29733=CARTESIAN_POINT('Ctrl Pts',(-39.0738472616523,-36.3607409549812,
4.76181040522164));
#29734=CARTESIAN_POINT('Ctrl Pts',(-39.0799345709982,-35.013663708426,4.7089502383075));
#29735=CARTESIAN_POINT('Ctrl Pts',(-39.0799229210932,-35.0002389671693,
4.70842344717745));
#29736=CARTESIAN_POINT('Ctrl Pts',(-39.0792024631389,-35.0015161209354,
5.79157655282255));
#29737=CARTESIAN_POINT('Ctrl Pts',(-39.0731679256319,-33.7557919674485,
5.74271706512043));
#29738=CARTESIAN_POINT('Ctrl Pts',(-37.8030027181165,-31.1651102767228,
5.64152420163424));
#29739=CARTESIAN_POINT('Ctrl Pts',(-33.4155016033557,-30.4724169111822,
5.48799796236394));
#29740=CARTESIAN_POINT('Ctrl Pts',(-30.3495576440316,-33.8239773440302,
5.3309978350117));
#29741=CARTESIAN_POINT('Ctrl Pts',(-31.4537101308888,-38.230088373826,5.17399770765944));
#29742=CARTESIAN_POINT('Ctrl Pts',(-35.7378546799324,-39.7397482704758,
5.01699758030718));
#29743=CARTESIAN_POINT('Ctrl Pts',(-38.6790876767283,-37.5146290150371,
4.88952386202822));
#29744=CARTESIAN_POINT('Ctrl Pts',(-39.0694004131258,-35.5870561070142,
4.81438351953334));
#29745=CARTESIAN_POINT('Ctrl Pts',(-39.0676603684793,-35.0013188448613,
4.79157655282255));
#29746=CARTESIAN_POINT('Origin',(-35.,-35.,10.2084234471775));
#29747=CARTESIAN_POINT('',(-39.0709664927331,-34.9967444357251,6.79157655282255));
#29748=CARTESIAN_POINT('',(-39.0721140267755,-35.0034548068065,6.70842344717746));
#29749=CARTESIAN_POINT('',(-39.0735,-34.9999999999999,10.2084234471775));
#29750=CARTESIAN_POINT('Ctrl Pts',(-39.0721140267755,-35.0034548068065,
6.70842344717746));
#29751=CARTESIAN_POINT('Ctrl Pts',(-39.0638862819908,-34.0266505561004,
6.67028408104986));
#29752=CARTESIAN_POINT('Ctrl Pts',(-38.2252022081515,-31.6968182141492,
6.57981133913816));
#29753=CARTESIAN_POINT('Ctrl Pts',(-34.3564136921927,-30.2465364275518,
6.4370052214424));
#29754=CARTESIAN_POINT('Ctrl Pts',(-30.6802034020135,-32.9145736277213,
6.28000509409013));
#29755=CARTESIAN_POINT('Ctrl Pts',(-30.8775957137286,-37.4526369907548,
6.12300496673789));
#29756=CARTESIAN_POINT('Ctrl Pts',(-34.7715877207675,-39.7913950861294,
5.96600483938563));
#29757=CARTESIAN_POINT('Ctrl Pts',(-38.3794222668459,-38.0681714287485,
5.82781099953215));
#29758=CARTESIAN_POINT('Ctrl Pts',(-39.0639983304887,-35.8575951283075,
5.74195053546276));
#29759=CARTESIAN_POINT('Ctrl Pts',(-39.0692231423099,-34.9973709029543,
5.70842344717745));
#29760=CARTESIAN_POINT('Ctrl Pts',(-39.0709664927331,-34.9967444357251,
6.79157655282255));
#29761=CARTESIAN_POINT('Ctrl Pts',(-39.074129342561,-34.5902726781194,6.77571736227569));
#29762=CARTESIAN_POINT('Ctrl Pts',(-38.8328831908397,-32.8461583454701,
6.70752479594475));
#29763=CARTESIAN_POINT('Ctrl Pts',(-36.3504797430715,-30.3972101963624,
6.58699885382972));
#29764=CARTESIAN_POINT('Ctrl Pts',(-31.905896825022,-31.3344599279876,6.42999872647746));
#29765=CARTESIAN_POINT('Ctrl Pts',(-30.2358028418083,-35.5586616666892,
6.27299859912522));
#29766=CARTESIAN_POINT('Ctrl Pts',(-32.83782160528,-39.2818926978495,6.11599847177295));
#29767=CARTESIAN_POINT('Ctrl Pts',(-37.3786807951101,-39.1655161353224,
5.95899834442071));
#29768=CARTESIAN_POINT('Ctrl Pts',(-39.0372097938135,-36.5125334877904,
5.85085770477057));
#29769=CARTESIAN_POINT('Ctrl Pts',(-39.0796315161011,-35.090086560245,5.79505044090452));
#29770=CARTESIAN_POINT('Ctrl Pts',(-39.0792024631389,-35.0015161209354,
5.79157655282255));
#29771=CARTESIAN_POINT('Origin',(-35.,-35.,10.2084234471775));
#29772=CARTESIAN_POINT('',(-39.0691247390887,-35.0040754761348,7.79157655282255));
#29773=CARTESIAN_POINT('',(-39.0784093524563,-34.997955826836,7.70842344717746));
#29774=CARTESIAN_POINT('',(-39.0735,-34.9999999999999,10.2084234471775));
#29775=CARTESIAN_POINT('',(-36.0520713770612,-38.9352951690526,8.));
#29776=CARTESIAN_POINT('Ctrl Pts',(-36.0520713770612,-38.9352951690526,
8.));
#29777=CARTESIAN_POINT('Ctrl Pts',(-37.3460763064865,-38.5893527455387,
7.94766662421592));
#29778=CARTESIAN_POINT('Ctrl Pts',(-38.8056934287649,-37.2206664159851,
7.87819214182344));
#29779=CARTESIAN_POINT('Ctrl Pts',(-39.0721265495934,-35.4436566771087,
7.80871765943095));
#29780=CARTESIAN_POINT('Ctrl Pts',(-39.0691247390887,-35.0040754761348,
7.79157655282255));
#29781=CARTESIAN_POINT('',(-33.9452801041878,-38.9416007879337,8.));
#29782=CARTESIAN_POINT('Origin',(-35.,-35.,8.));
#29783=CARTESIAN_POINT('Ctrl Pts',(-33.9452677648582,-38.941630165528,8.));
#29784=CARTESIAN_POINT('Ctrl Pts',(-35.1775571519718,-39.2670003808689,
7.95000212253756));
#29785=CARTESIAN_POINT('Ctrl Pts',(-37.9028288422611,-38.6929823061133,
7.85280993826337));
#29786=CARTESIAN_POINT('Ctrl Pts',(-39.0706575059758,-36.2016126262027,
7.75561775398919));
#29787=CARTESIAN_POINT('Ctrl Pts',(-39.0784093524563,-34.997955826836,7.70842344717745));
#29788=CARTESIAN_POINT('Origin',(35.,35.,10.2084234471775));
#29789=CARTESIAN_POINT('',(30.9212698233586,35.0019483146883,0.791576552822542));
#29790=CARTESIAN_POINT('',(30.9328374281389,34.9998406908479,0.708423447177449));
#29791=CARTESIAN_POINT('',(30.9265,35.0000000000001,10.2084234471775));
#29792=CARTESIAN_POINT('',(36.0520713770613,31.0647048309474,0.));
#29793=CARTESIAN_POINT('Ctrl Pts',(30.9328374281389,34.9998406908479,0.708423447177449));
#29794=CARTESIAN_POINT('Ctrl Pts',(30.9332828479214,35.688557610158,0.681615801254637));
#29795=CARTESIAN_POINT('Ctrl Pts',(31.423729103703,37.7222371568615,0.602474779547742));
#29796=CARTESIAN_POINT('Ctrl Pts',(34.620473026815,39.7808594262888,0.47100038205676));
#29797=CARTESIAN_POINT('Ctrl Pts',(38.7813013396977,37.9557820285754,0.314000254704507));
#29798=CARTESIAN_POINT('Ctrl Pts',(39.5450610063768,33.4726465453437,0.157000127352254));
#29799=CARTESIAN_POINT('Ctrl Pts',(37.3460763064866,31.4106472544613,0.0523333757840845));
#29800=CARTESIAN_POINT('Ctrl Pts',(36.0520713770613,31.0647048309474,0.));
#29801=CARTESIAN_POINT('',(33.9452806327216,31.0583991975554,1.9516645121422E-15));
#29802=CARTESIAN_POINT('Origin',(35.,35.,0.));
#29803=CARTESIAN_POINT('Ctrl Pts',(30.9212698233586,35.0019483146883,0.791576552822542));
#29804=CARTESIAN_POINT('Ctrl Pts',(30.9205865489415,35.1174152630019,0.787049082480475));
#29805=CARTESIAN_POINT('Ctrl Pts',(30.9769552830328,36.5668922956884,0.730188236354323));
#29806=CARTESIAN_POINT('Ctrl Pts',(32.7044910542971,39.2117680815463,0.620994014444087));
#29807=CARTESIAN_POINT('Ctrl Pts',(37.246817707304,39.2384377086451,0.463993887091833));
#29808=CARTESIAN_POINT('Ctrl Pts',(39.7742802645754,35.4632838929154,0.30699375973958));
#29809=CARTESIAN_POINT('Ctrl Pts',(38.0469271024438,31.3373709383794,0.152329130708969));
#29810=CARTESIAN_POINT('Ctrl Pts',(35.1775581103468,30.7329992432291,0.0499978774624438));
#29811=CARTESIAN_POINT('Ctrl Pts',(33.9452683089267,31.0583698510224,2.42915496745377E-15));
#29812=CARTESIAN_POINT('Origin',(35.,35.,10.2084234471775));
#29813=CARTESIAN_POINT('',(30.9325668217157,35.0009171562606,1.79157655282254));
#29814=CARTESIAN_POINT('',(30.9221793985577,34.9975078813789,1.70842344717745));
#29815=CARTESIAN_POINT('',(30.9265,35.0000000000001,10.2084234471775));
#29816=CARTESIAN_POINT('Ctrl Pts',(30.9221793985577,34.9975078813789,1.70842344717745));
#29817=CARTESIAN_POINT('Ctrl Pts',(30.9307243035611,36.174970446985,1.66228272262581));
#29818=CARTESIAN_POINT('Ctrl Pts',(32.0812069040633,38.7025089358584,1.56380862229009));
#29819=CARTESIAN_POINT('Ctrl Pts',(36.3504798927025,39.6027903023767,1.41300114617028));
#29820=CARTESIAN_POINT('Ctrl Pts',(39.5841214241815,36.41272834745,1.25600101881803));
#29821=CARTESIAN_POINT('Ctrl Pts',(38.7070437601939,31.9557497473198,1.09900089146578));
#29822=CARTESIAN_POINT('Ctrl Pts',(34.5060128656572,30.2288003607244,0.942000764113522));
#29823=CARTESIAN_POINT('Ctrl Pts',(31.3893171307454,32.344207693053,0.811808282684079));
#29824=CARTESIAN_POINT('Ctrl Pts',(30.9324133079056,34.3440575577889,0.733949177038721));
#29825=CARTESIAN_POINT('Ctrl Pts',(30.9328374281389,34.9998406908479,0.708423447177449));
#29826=CARTESIAN_POINT('Ctrl Pts',(30.9325668217157,35.0009171562606,1.79157655282254));
#29827=CARTESIAN_POINT('Ctrl Pts',(30.9313054599248,35.6137984881563,1.76771600385165));
#29828=CARTESIAN_POINT('Ctrl Pts',(31.3469046036967,37.5692890939049,1.69152207909667));
#29829=CARTESIAN_POINT('Ctrl Pts',(34.3564137772933,39.7534629455386,1.56299477855761));
#29830=CARTESIAN_POINT('Ctrl Pts',(38.6097344321268,38.159032706872,1.40599465120535));
#29831=CARTESIAN_POINT('Ctrl Pts',(39.6261697761982,33.7318499178854,1.2489945238531));
#29832=CARTESIAN_POINT('Ctrl Pts',(36.4942779564007,30.441864951573,1.09199439650085));
#29833=CARTESIAN_POINT('Ctrl Pts',(32.1514012728307,31.2161408778184,0.939521739490661));
#29834=CARTESIAN_POINT('Ctrl Pts',(30.9284845701608,33.7827239806345,0.839382458264559));
#29835=CARTESIAN_POINT('Ctrl Pts',(30.9212698233586,35.0019483146883,0.791576552822542));
#29836=CARTESIAN_POINT('Origin',(35.,35.,10.2084234471775));
#29837=CARTESIAN_POINT('',(30.9241571699662,34.9967917637985,2.79157655282254));
#29838=CARTESIAN_POINT('',(30.9271222988705,35.0035058204319,2.70842344717745));
#29839=CARTESIAN_POINT('',(30.9265,35.0000000000001,10.2084234471775));
#29840=CARTESIAN_POINT('Ctrl Pts',(30.9271222988705,35.0035058204319,2.70842344717745));
#29841=CARTESIAN_POINT('Ctrl Pts',(30.9241957830228,35.3398900680519,2.69528301978107));
#29842=CARTESIAN_POINT('Ctrl Pts',(31.1149285017256,37.0126943772598,2.62980921660061));
#29843=CARTESIAN_POINT('Ctrl Pts',(33.415501444059,39.52758354292,2.51200203763605));
#29844=CARTESIAN_POINT('Ctrl Pts',(37.902280422705,38.8192163097165,2.3550019102838));
#29845=CARTESIAN_POINT('Ctrl Pts',(39.7865573966804,34.6861219842625,2.19800178293155));
#29846=CARTESIAN_POINT('Ctrl Pts',(37.3786810353442,30.8344834494167,2.0410016555793));
#29847=CARTESIAN_POINT('Ctrl Pts',(32.8378213856151,30.7181068667712,1.88400152822704));
#29848=CARTESIAN_POINT('Ctrl Pts',(31.0005090266209,33.347118822167,1.77314212542643));
#29849=CARTESIAN_POINT('Ctrl Pts',(30.9210325674879,34.839477961413,1.7146160984099));
#29850=CARTESIAN_POINT('Ctrl Pts',(30.9221793985577,34.9975078813789,1.70842344717745));
#29851=CARTESIAN_POINT('Ctrl Pts',(30.9241571699662,34.9967917637985,2.79157655282254));
#29852=CARTESIAN_POINT('Ctrl Pts',(30.9336808617147,36.100441855715,2.74838292522282));
#29853=CARTESIAN_POINT('Ctrl Pts',(31.9624563163556,38.5569288706128,2.65285592183902));
#29854=CARTESIAN_POINT('Ctrl Pts',(36.0928480916297,39.6706871647746,2.50499554267113));
#29855=CARTESIAN_POINT('Ctrl Pts',(39.4985859434327,36.6650407532663,2.34799541531887));
#29856=CARTESIAN_POINT('Ctrl Pts',(38.8703985950797,32.1663360606625,2.19099528796662));
#29857=CARTESIAN_POINT('Ctrl Pts',(34.7715877503781,30.208605539026,2.03399516061437));
#29858=CARTESIAN_POINT('Ctrl Pts',(31.4693968846214,32.1919238394657,1.90085558223301));
#29859=CARTESIAN_POINT('Ctrl Pts',(30.9340720065237,34.2695649966187,1.82004937963573));
#29860=CARTESIAN_POINT('Ctrl Pts',(30.9325668217157,35.0009171562606,1.79157655282254));
#29861=CARTESIAN_POINT('Origin',(35.,35.,10.2084234471775));
#29862=CARTESIAN_POINT('',(30.9249288558452,35.0033643601501,3.79157655282254));
#29863=CARTESIAN_POINT('',(30.9312884745882,34.9976733861211,3.70842344717745));
#29864=CARTESIAN_POINT('',(30.9265,35.0000000000001,10.2084234471775));
#29865=CARTESIAN_POINT('Ctrl Pts',(30.9312884745882,34.9976733861211,3.70842344717745));
#29866=CARTESIAN_POINT('Ctrl Pts',(30.935730046206,35.8311295271992,3.67594994115225));
#29867=CARTESIAN_POINT('Ctrl Pts',(31.587554790492,38.0141386637623,3.59114305934295));
#29868=CARTESIAN_POINT('Ctrl Pts',(35.1332185480963,39.7949870216991,3.45400280174957));
#29869=CARTESIAN_POINT('Ctrl Pts',(39.0728867488228,37.5340168101838,3.29700267439732));
#29870=CARTESIAN_POINT('Ctrl Pts',(39.360358338736,33.0007694268683,3.14000254704507));
#29871=CARTESIAN_POINT('Ctrl Pts',(35.7378547540399,30.2602512537625,2.98300241969282));
#29872=CARTESIAN_POINT('Ctrl Pts',(31.8122795225231,31.6435574026667,2.83914271973694));
#29873=CARTESIAN_POINT('Ctrl Pts',(30.9358509939969,34.0001982370698,2.74761639556516));
#29874=CARTESIAN_POINT('Ctrl Pts',(30.9271222988705,35.0035058204319,2.70842344717745));
#29875=CARTESIAN_POINT('Ctrl Pts',(30.9249288558452,35.0033643601501,3.79157655282255));
#29876=CARTESIAN_POINT('Ctrl Pts',(30.9226267326427,35.2639441772806,3.78138322237808));
#29877=CARTESIAN_POINT('Ctrl Pts',(31.0631418150181,36.8598902688347,3.71885651614953));
#29878=CARTESIAN_POINT('Ctrl Pts',(33.1665614759356,39.4326221439007,3.60399643413691));
#29879=CARTESIAN_POINT('Ctrl Pts',(37.6857489237188,38.9744670842276,3.44699630678464));
#29880=CARTESIAN_POINT('Ctrl Pts',(39.7965995458586,34.9523692628263,3.2899961794324));
#29881=CARTESIAN_POINT('Ctrl Pts',(37.6062933383462,30.9729823764193,3.13299605208014));
#29882=CARTESIAN_POINT('Ctrl Pts',(33.078898891504,30.6046608345122,2.97599592472789));
#29883=CARTESIAN_POINT('Ctrl Pts',(31.0458056637607,33.1946781012295,2.86218942497536));
#29884=CARTESIAN_POINT('Ctrl Pts',(30.9221419619551,34.7632600026498,2.80071630100691));
#29885=CARTESIAN_POINT('Ctrl Pts',(30.9241571699662,34.9967917637985,2.79157655282254));
#29886=CARTESIAN_POINT('Origin',(35.,35.,10.2084234471775));
#29887=CARTESIAN_POINT('',(30.9323402673974,34.9986811553562,4.79157655282255));
#29888=CARTESIAN_POINT('',(30.920076562846,34.9997610327988,4.70842344717745));
#29889=CARTESIAN_POINT('',(30.9265,35.0000000000001,10.2084234471775));
#29890=CARTESIAN_POINT('Ctrl Pts',(30.920076562846,34.9997610327988,4.70842344717745));
#29891=CARTESIAN_POINT('Ctrl Pts',(30.9212222576611,36.3199998194329,4.65661686252342));
#29892=CARTESIAN_POINT('Ctrl Pts',(32.3294138679696,38.9760053777146,4.5524769020853));
#29893=CARTESIAN_POINT('Ctrl Pts',(36.833438994737,39.4326232818222,4.39600356586309));
#29894=CARTESIAN_POINT('Ctrl Pts',(39.7085652668935,35.9160026365752,4.23900343851085));
#29895=CARTESIAN_POINT('Ctrl Pts',(38.3614758924016,31.5779936400392,4.08200331115859));
#29896=CARTESIAN_POINT('Ctrl Pts',(34.0001188363665,30.3085305751198,3.92500318380634));
#29897=CARTESIAN_POINT('Ctrl Pts',(31.2520057006646,32.6383841561994,3.80047656247929));
#29898=CARTESIAN_POINT('Ctrl Pts',(30.9285721361126,34.4879553902047,3.72828331693633));
#29899=CARTESIAN_POINT('Ctrl Pts',(30.9312884745882,34.9976733861211,3.70842344717745));
#29900=CARTESIAN_POINT('Ctrl Pts',(30.9323402673974,34.9986811553562,4.79157655282255));
#29901=CARTESIAN_POINT('Ctrl Pts',(30.9345929677557,35.7569895936223,4.76205014374926));
#29902=CARTESIAN_POINT('Ctrl Pts',(31.4994186633631,37.8624608556942,4.68019035889188));
#29903=CARTESIAN_POINT('Ctrl Pts',(34.86678148609,39.7949857907703,4.54599719825042));
#29904=CARTESIAN_POINT('Ctrl Pts',(38.9259070000539,37.7562456562111,4.38899707089817));
#29905=CARTESIAN_POINT('Ctrl Pts',(39.4646340410498,33.2459536025622,4.23199694354592));
#29906=CARTESIAN_POINT('Ctrl Pts',(35.9998809069499,30.3085317794917,4.07499681619366));
#29907=CARTESIAN_POINT('Ctrl Pts',(31.9216887041993,31.4955738644524,3.92819001928588));
#29908=CARTESIAN_POINT('Ctrl Pts',(30.9344460177445,33.9261065033295,3.83371659816217));
#29909=CARTESIAN_POINT('Ctrl Pts',(30.9249288558452,35.0033643601501,3.79157655282255));
#29910=CARTESIAN_POINT('Origin',(35.,35.,10.2084234471775));
#29911=CARTESIAN_POINT('',(30.9207981741727,34.9984838800189,5.79157655282254));
#29912=CARTESIAN_POINT('',(30.93077634299,35.0026290974327,5.70842344717745));
#29913=CARTESIAN_POINT('',(30.9265,35.0000000000001,10.2084234471775));
#29914=CARTESIAN_POINT('Ctrl Pts',(30.93077634299,35.0026290974327,5.70842344717745));
#29915=CARTESIAN_POINT('Ctrl Pts',(30.9278455986019,35.4851531389532,5.68961715967867));
#29916=CARTESIAN_POINT('Ctrl Pts',(31.2287021394076,37.3068916052531,5.61847749639582));
#29917=CARTESIAN_POINT('Ctrl Pts',(33.9071516278456,39.6706883641509,5.49500445732887));
#29918=CARTESIAN_POINT('Ctrl Pts',(38.2928579600589,38.4880846134226,5.33800432997661));
#29919=CARTESIAN_POINT('Ctrl Pts',(39.72582697599,34.1776818622125,5.18100420262437));
#29920=CARTESIAN_POINT('Ctrl Pts',(36.9211016016709,30.6046597061106,5.0240040752721));
#29921=CARTESIAN_POINT('Ctrl Pts',(32.3937059925777,30.9729813426439,4.86700394791986));
#29922=CARTESIAN_POINT('Ctrl Pts',(30.9261522230555,33.6392588729013,4.76181040522164));
#29923=CARTESIAN_POINT('Ctrl Pts',(30.9200649129395,34.986336289844,4.7089502383075));
#29924=CARTESIAN_POINT('Ctrl Pts',(30.920076562846,34.9997610327988,4.70842344717745));
#29925=CARTESIAN_POINT('Ctrl Pts',(30.9207981741727,34.9984838800189,5.79157655282254));
#29926=CARTESIAN_POINT('Ctrl Pts',(30.9268327105953,36.2442078390725,5.74271706512043));
#29927=CARTESIAN_POINT('Ctrl Pts',(32.1969977207135,38.8348891225654,5.64152420163423));
#29928=CARTESIAN_POINT('Ctrl Pts',(36.5844981485848,39.5275823816942,5.48799796236394));
#29929=CARTESIAN_POINT('Ctrl Pts',(39.6504416291735,36.1760224717832,5.33099783501169));
#29930=CARTESIAN_POINT('Ctrl Pts',(38.5462893146292,31.7699121313011,5.17399770765944));
#29931=CARTESIAN_POINT('Ctrl Pts',(34.2621454354683,30.2602524703801,5.01699758030718));
#29932=CARTESIAN_POINT('Ctrl Pts',(31.3209128983978,32.4853713780877,4.88952386202822));
#29933=CARTESIAN_POINT('Ctrl Pts',(30.9306002230203,34.4129439847737,4.81438351953334));
#29934=CARTESIAN_POINT('Ctrl Pts',(30.9323402673974,34.9986811553562,4.79157655282255));
#29935=CARTESIAN_POINT('Origin',(35.,35.,10.2084234471775));
#29936=CARTESIAN_POINT('',(30.9290341434093,35.0032555560525,6.79157655282255));
#29937=CARTESIAN_POINT('',(30.9278854598697,34.9965452008231,6.70842344717745));
#29938=CARTESIAN_POINT('',(30.9265,35.0000000000001,10.2084234471775));
#29939=CARTESIAN_POINT('Ctrl Pts',(30.9278854598697,34.9965452008231,6.70842344717745));
#29940=CARTESIAN_POINT('Ctrl Pts',(30.9361132054557,35.973349573232,6.67028408104985));
#29941=CARTESIAN_POINT('Ctrl Pts',(31.7747973816342,38.3031821914714,6.57981133913817));
#29942=CARTESIAN_POINT('Ctrl Pts',(35.6435863904507,39.7534641813021,6.43700522144238));
#29943=CARTESIAN_POINT('Ctrl Pts',(39.3197971438036,37.085426632005,6.28000509409014));
#29944=CARTESIAN_POINT('Ctrl Pts',(39.122404807981,32.5473627011697,6.12300496673788));
#29945=CARTESIAN_POINT('Ctrl Pts',(35.2284123079944,30.2086043066787,5.96600483938564));
#29946=CARTESIAN_POINT('Ctrl Pts',(31.6205773057362,31.9318281835565,5.82781099953215));
#29947=CARTESIAN_POINT('Ctrl Pts',(30.9360011554815,34.1424047633691,5.74195053546276));
#29948=CARTESIAN_POINT('Ctrl Pts',(30.93077634299,35.0026290974327,5.70842344717745));
#29949=CARTESIAN_POINT('Ctrl Pts',(30.9290341434093,35.0032555560525,6.79157655282255));
#29950=CARTESIAN_POINT('Ctrl Pts',(30.9258712893501,35.4097272653281,6.77571736227569));
#29951=CARTESIAN_POINT('Ctrl Pts',(31.167117385295,37.1538413864501,6.70752479594475));
#29952=CARTESIAN_POINT('Ctrl Pts',(33.6495204900336,39.6027890266495,6.58699885382972));
#29953=CARTESIAN_POINT('Ctrl Pts',(38.0941026784935,38.6655395297167,6.42999872647747));
#29954=CARTESIAN_POINT('Ctrl Pts',(39.7641964207046,34.4413384042963,6.27299859912521));
#29955=CARTESIAN_POINT('Ctrl Pts',(37.1621780526355,30.7181079801836,6.11599847177296));
#29956=CARTESIAN_POINT('Ctrl Pts',(32.6213195789955,30.8344845112897,5.95899834442071));
#29957=CARTESIAN_POINT('Ctrl Pts',(30.9627908371619,33.4874667488915,5.85085770477057));
#29958=CARTESIAN_POINT('Ctrl Pts',(30.9203691212877,34.9099134545334,5.79505044090451));
#29959=CARTESIAN_POINT('Ctrl Pts',(30.9207981741727,34.9984838800189,5.79157655282254));
#29960=CARTESIAN_POINT('Origin',(35.,35.,10.2084234471775));
#29961=CARTESIAN_POINT('',(30.9308749498806,34.995920959377,7.79157655282255));
#29962=CARTESIAN_POINT('',(30.9215901961247,35.0020443570103,7.70842344717745));
#29963=CARTESIAN_POINT('',(30.9265,35.0000000000001,10.2084234471775));
#29964=CARTESIAN_POINT('',(33.9479286229388,31.0647048309474,8.));
#29965=CARTESIAN_POINT('Ctrl Pts',(33.9479286229388,31.0647048309474,8.));
#29966=CARTESIAN_POINT('Ctrl Pts',(32.6539236935135,31.4106472544613,7.94766662421592));
#29967=CARTESIAN_POINT('Ctrl Pts',(31.1943056926496,32.7793278989778,7.87819214182343));
#29968=CARTESIAN_POINT('Ctrl Pts',(30.927873001558,34.5563391849396,7.80871765943095));
#29969=CARTESIAN_POINT('Ctrl Pts',(30.9308749498806,34.995920959377,7.79157655282255));
#29970=CARTESIAN_POINT('',(36.0547204053665,31.0583992220146,8.));
#29971=CARTESIAN_POINT('Origin',(35.,35.,8.));
#29972=CARTESIAN_POINT('Ctrl Pts',(36.0547327596422,31.0583698145405,8.));
#29973=CARTESIAN_POINT('Ctrl Pts',(34.8224437745751,30.7329999802434,7.95000212253756));
#29974=CARTESIAN_POINT('Ctrl Pts',(32.0971699315749,31.3070160119469,7.85280993826337));
#29975=CARTESIAN_POINT('Ctrl Pts',(30.9293418770678,33.7983871843493,7.75561775398919));
#29976=CARTESIAN_POINT('Ctrl Pts',(30.9215901961247,35.0020443570103,7.70842344717745));
#29977=CARTESIAN_POINT('Origin',(35.,35.,10.2084234471775));
#29978=CARTESIAN_POINT('Ctrl Pts',(30.9215901961247,35.0020443570103,7.70842344717745));
#29979=CARTESIAN_POINT('Ctrl Pts',(30.9207461022984,35.1331126499304,7.70328437820511));
#29980=CARTESIAN_POINT('Ctrl Pts',(30.985475579174,36.5980980633283,7.64581193344868));
#29981=CARTESIAN_POINT('Ctrl Pts',(32.753181262015,39.238437809064,7.53600611290817));
#29982=CARTESIAN_POINT('Ctrl Pts',(37.2955097522044,39.2117697306779,7.37900598555592));
#29983=CARTESIAN_POINT('Ctrl Pts',(39.7793716811886,35.4089491092894,7.22200585820366));
#29984=CARTESIAN_POINT('Ctrl Pts',(37.9775554192851,31.2391311721338,7.06500573085141));
#29985=CARTESIAN_POINT('Ctrl Pts',(33.5057216363881,30.441863683446,6.90800560349916));
#29986=CARTESIAN_POINT('Ctrl Pts',(31.1346462527125,32.9326274967327,6.7891448422745));
#29987=CARTESIAN_POINT('Ctrl Pts',(30.9248234084473,34.6330160680086,6.72261745683393));
#29988=CARTESIAN_POINT('Ctrl Pts',(30.9278854598697,34.9965452008231,6.70842344717745));
#29989=CARTESIAN_POINT('Ctrl Pts',(30.9308749498806,34.995920959377,7.79157655282255));
#29990=CARTESIAN_POINT('Ctrl Pts',(30.9370382260235,35.8984227922016,7.75638428364686));
#29991=CARTESIAN_POINT('Ctrl Pts',(31.6729751170447,38.1550462153353,7.66885863868709));
#29992=CARTESIAN_POINT('Ctrl Pts',(35.3795268052061,39.7808547962683,7.52899961794324));
#29993=CARTESIAN_POINT('Ctrl Pts',(39.1969168896572,37.3225573472918,7.37199949059099));
#29994=CARTESIAN_POINT('Ctrl Pts',(39.2524338890068,32.7797860374403,7.21499936323873));
#29995=CARTESIAN_POINT('Ctrl Pts',(35.4939868648458,30.2288021766129,7.05799923588648));
#29996=CARTESIAN_POINT('Ctrl Pts',(31.7173195455156,31.7813045011721,6.91685829908108));
#29997=CARTESIAN_POINT('Ctrl Pts',(30.9363083182476,34.0684206807159,6.82805073805977));
#29998=CARTESIAN_POINT('Ctrl Pts',(30.9290341434093,35.0032555560525,6.79157655282255));
#29999=CARTESIAN_POINT('Ctrl Pts',(37.6735319337713,37.2858331630076,8.));
#30000=CARTESIAN_POINT('Ctrl Pts',(38.4251602751564,36.4067215963626,7.94766662421592));
#30001=CARTESIAN_POINT('Ctrl Pts',(38.981419710079,33.8637820915388,7.84299987264775));
#30002=CARTESIAN_POINT('Ctrl Pts',(36.2450923914777,31.0470745569746,7.68599974529549));
#30003=CARTESIAN_POINT('Ctrl Pts',(32.3914750767338,31.7834880469926,7.52899961794325));
#30004=CARTESIAN_POINT('Ctrl Pts',(30.877370367455,35.4000509161799,7.37199949059098));
#30005=CARTESIAN_POINT('Ctrl Pts',(33.0598539558457,38.6599251241887,7.21499936323874));
#30006=CARTESIAN_POINT('Ctrl Pts',(36.9821911263972,38.6368970240971,7.05799923588648));
#30007=CARTESIAN_POINT('Ctrl Pts',(39.1270258717517,35.3531308437279,6.90099910853422));
#30008=CARTESIAN_POINT('Ctrl Pts',(37.5711430434112,31.75245953062,6.74399898118198));
#30009=CARTESIAN_POINT('Ctrl Pts',(33.7096786193679,31.0640126442915,6.58699885382972));
#30010=CARTESIAN_POINT('Ctrl Pts',(31.0052641890983,33.9049419734146,6.42999872647747));
#30011=CARTESIAN_POINT('Ctrl Pts',(31.882964491631,37.7278508156672,6.27299859912521));
#30012=CARTESIAN_POINT('Ctrl Pts',(35.5557420224402,39.1046545373095,6.11599847177296));
#30013=CARTESIAN_POINT('Ctrl Pts',(38.7301795638466,36.8007826630852,5.9589983444207));
#30014=CARTESIAN_POINT('Ctrl Pts',(38.559729694875,32.8821279738221,5.80199821706846));
#30015=CARTESIAN_POINT('Ctrl Pts',(35.1972358643355,30.8625912971014,5.64499808971619));
#30016=CARTESIAN_POINT('Ctrl Pts',(31.6578788381682,32.5531077792767,5.48799796236396));
#30017=CARTESIAN_POINT('Ctrl Pts',(31.1154338729727,36.437776445535,5.33099783501168));
#30018=CARTESIAN_POINT('Ctrl Pts',(34.0563166443959,39.033176953701,5.17399770765944));
#30019=CARTESIAN_POINT('Ctrl Pts',(37.843409322329,38.0119891070858,5.01699758030718));
#30020=CARTESIAN_POINT('Ctrl Pts',(39.0807895883257,34.2899216767724,4.85999745295493));
#30021=CARTESIAN_POINT('Ctrl Pts',(36.6588866782563,31.2045883187048,4.70299732560268));
#30022=CARTESIAN_POINT('Ctrl Pts',(32.7494441705885,31.5226370130723,4.54599719825042));
#30023=CARTESIAN_POINT('Ctrl Pts',(30.8580966653042,34.9588704649406,4.38899707089817));
#30024=CARTESIAN_POINT('Ctrl Pts',(32.6808336162004,38.4319851620801,4.23199694354592));
#30025=CARTESIAN_POINT('Ctrl Pts',(36.5831893123819,38.8276058411217,4.07499681619366));
#30026=CARTESIAN_POINT('Ctrl Pts',(39.0658839637408,35.7909756411325,3.91799668884141));
#30027=CARTESIAN_POINT('Ctrl Pts',(37.9026614585792,32.0450699960324,3.76099656148916));
#30028=CARTESIAN_POINT('Ctrl Pts',(34.1365945763887,30.9488784332844,3.6039964341369));
#30029=CARTESIAN_POINT('Ctrl Pts',(31.1447516212191,33.4853664448484,3.44699630678465));
#30030=CARTESIAN_POINT('Ctrl Pts',(31.6099468717921,37.3800408947213,3.2899961794324));
#30031=CARTESIAN_POINT('Ctrl Pts',(35.1150352873275,39.1405098438263,3.13299605208014));
#30032=CARTESIAN_POINT('Ctrl Pts',(38.5169704526781,37.1881438885041,2.97599592472789));
#30033=CARTESIAN_POINT('Ctrl Pts',(38.7652044817734,33.2736483267483,2.81899579737564));
#30034=CARTESIAN_POINT('Ctrl Pts',(35.6371435122955,30.9071888511377,2.66199567002338));
#30035=CARTESIAN_POINT('Ctrl Pts',(31.9377498791963,32.2107924399309,2.50499554267113));
#30036=CARTESIAN_POINT('Ctrl Pts',(30.9843052341107,36.0155051205153,2.34799541531888));
#30037=CARTESIAN_POINT('Ctrl Pts',(33.6317727579422,38.9096047900383,2.19099528796662));
#30038=CARTESIAN_POINT('Ctrl Pts',(37.5061424786706,38.297923989058,2.03399516061437));
#30039=CARTESIAN_POINT('Ctrl Pts',(39.1332307948504,34.7289638099038,1.87699503326212));
#30040=CARTESIAN_POINT('Ctrl Pts',(37.0540101980664,31.4030429687795,1.71999490590986));
#30041=CARTESIAN_POINT('Ctrl Pts',(33.1329413830615,31.3025508540242,1.56299477855761));
#30042=CARTESIAN_POINT('Ctrl Pts',(30.8860770418796,34.5175911198794,1.40599465120536));
#30043=CARTESIAN_POINT('Ctrl Pts',(32.3282167572518,38.1652236231046,1.2489945238531));
#30044=CARTESIAN_POINT('Ctrl Pts',(36.1661502448953,38.9745464314742,1.09199439650085));
#30045=CARTESIAN_POINT('Ctrl Pts',(38.9584257050592,36.219902286033,0.934994269148596));
#30046=CARTESIAN_POINT('Ctrl Pts',(38.2010620907038,32.3712654317411,0.777994141796343));
#30047=CARTESIAN_POINT('Ctrl Pts',(34.5734381379524,30.8800307521414,0.620994014444089));
#30048=CARTESIAN_POINT('Ctrl Pts',(31.3279883656859,33.0828278259953,0.463993887091835));
#30049=CARTESIAN_POINT('Ctrl Pts',(31.3759274478189,37.0055458008236,0.306993759739581));
#30050=CARTESIAN_POINT('Ctrl Pts',(34.6722754073454,39.1283105516069,0.149993632387328));
#30051=CARTESIAN_POINT('Ctrl Pts',(38.2651841076192,37.5523415454803,-0.007006494964925));
#30052=CARTESIAN_POINT('Ctrl Pts',(38.9246967202481,33.681118012335,-0.164006622317179));
#30053=CARTESIAN_POINT('Ctrl Pts',(37.0258557525633,31.9005650466596,-0.268673373885348));
#30054=CARTESIAN_POINT('Ctrl Pts',(35.9084720925035,31.6018409826581,-0.321006749669432));
#30055=CARTESIAN_POINT('Ctrl Pts',(37.8143974874483,37.4062712808594,8.10700224988981));
#30056=CARTESIAN_POINT('Ctrl Pts',(38.6056283266121,36.4808402609044,8.05466887410573));
#30057=CARTESIAN_POINT('Ctrl Pts',(39.1911964794515,33.80391597857,7.95000212253756));
#30058=CARTESIAN_POINT('Ctrl Pts',(36.3106949851439,30.8387991202229,7.7930019951853));
#30059=CARTESIAN_POINT('Ctrl Pts',(32.2540346732905,31.6140134536857,7.63600186783305));
#30060=CARTESIAN_POINT('Ctrl Pts',(30.6601533974768,35.4211291734076,7.4790017404808));
#30061=CARTESIAN_POINT('Ctrl Pts',(32.9576297245688,38.8527626858139,7.32200161312855));
#30062=CARTESIAN_POINT('Ctrl Pts',(37.0866306683329,38.828521259624,7.16500148577629));
#30063=CARTESIAN_POINT('Ctrl Pts',(39.3444744748973,35.3717369322484,7.00800135842404));
#30064=CARTESIAN_POINT('Ctrl Pts',(37.7066138353691,31.5813500777913,6.85100123107178));
#30065=CARTESIAN_POINT('Ctrl Pts',(33.6416929583746,30.856629657343,6.69400110371953));
#30066=CARTESIAN_POINT('Ctrl Pts',(30.7947858085381,33.8472445308389,6.53700097636727));
#30067=CARTESIAN_POINT('Ctrl Pts',(31.7187312063761,37.8715783734507,6.38000084901503));
#30068=CARTESIAN_POINT('Ctrl Pts',(35.5850234784437,39.3209244186404,6.22300072166276));
#30069=CARTESIAN_POINT('Ctrl Pts',(38.9267187571656,36.8956639860585,6.06600059431053));
#30070=CARTESIAN_POINT('Ctrl Pts',(38.7472880659103,32.7705395496047,5.90900046695826));
#30071=CARTESIAN_POINT('Ctrl Pts',(35.2076280122218,30.6445956336272,5.75200033960601));
#30072=CARTESIAN_POINT('Ctrl Pts',(31.4817860292625,32.4241836309969,5.59500021225375));
#30073=CARTESIAN_POINT('Ctrl Pts',(30.9107602158652,36.5135313570458,5.4380000849015));
#30074=CARTESIAN_POINT('Ctrl Pts',(34.0065949722125,39.2456807571843,5.28099995754925));
#30075=CARTESIAN_POINT('Ctrl Pts',(37.9932255349056,38.1706876091981,5.12399983019699));
#30076=CARTESIAN_POINT('Ctrl Pts',(39.2958020508805,34.2525084052524,4.96699970284474));
#30077=CARTESIAN_POINT('Ctrl Pts',(36.7462916527279,31.0046121145067,4.80999957549249));
#30078=CARTESIAN_POINT('Ctrl Pts',(32.6308647779182,31.3394184562628,4.65299944814024));
#30079=CARTESIAN_POINT('Ctrl Pts',(30.6398641844617,34.956703393489,4.49599932078798));
#30080=CARTESIAN_POINT('Ctrl Pts',(32.5586392064025,38.612812809568,4.33899919343573));
#30081=CARTESIAN_POINT('Ctrl Pts',(36.6666058731669,39.0292783213552,4.18199906608348));
#30082=CARTESIAN_POINT('Ctrl Pts',(39.2801110647917,35.8326513062801,4.02499893873122));
#30083=CARTESIAN_POINT('Ctrl Pts',(38.0555996031866,31.889377877368,3.86799881137897));
#30084=CARTESIAN_POINT('Ctrl Pts',(34.0911026630479,30.7354291472295,3.71099868402672));
#30085=CARTESIAN_POINT('Ctrl Pts',(30.9416226850806,33.4055620139871,3.55399855667446));
#30086=CARTESIAN_POINT('Ctrl Pts',(31.4313285785645,37.5054427177457,3.39699842932221));
#30087=CARTESIAN_POINT('Ctrl Pts',(35.1210963742505,39.3586689031172,3.23999830196995));
#30088=CARTESIAN_POINT('Ctrl Pts',(38.7022758847263,37.3034348623974,3.0829981746177));
#30089=CARTESIAN_POINT('Ctrl Pts',(38.9635891007609,33.1826886934549,2.92599804726545));
#30090=CARTESIAN_POINT('Ctrl Pts',(35.6707139262103,30.691542985346,2.76899791991319));
#30091=CARTESIAN_POINT('Ctrl Pts',(31.7764031777353,32.0638320605518,2.61199779256094));
#30092=CARTESIAN_POINT('Ctrl Pts',(30.7727225485069,36.0690110050931,2.45499766520869));
#30093=CARTESIAN_POINT('Ctrl Pts',(33.5596823199811,39.1155977076656,2.29799753785643));
#30094=CARTESIAN_POINT('Ctrl Pts',(37.6381884600154,38.4716880959441,2.14099741050418));
#30095=CARTESIAN_POINT('Ctrl Pts',(39.3510063287937,34.7146832013567,1.98399728315193));
#30096=CARTESIAN_POINT('Ctrl Pts',(37.1622338104923,31.2135231289919,1.82699715579967));
#30097=CARTESIAN_POINT('Ctrl Pts',(33.0345680505794,31.1077361916065,1.66999702844742));
#30098=CARTESIAN_POINT('Ctrl Pts',(30.6693188173153,34.4921735091382,1.51299690109517));
#30099=CARTESIAN_POINT('Ctrl Pts',(32.1874433402447,38.3319958888659,1.35599677374292));
#30100=CARTESIAN_POINT('Ctrl Pts',(36.227593460831,39.1839610551084,1.19899664639066));
#30101=CARTESIAN_POINT('Ctrl Pts',(39.1669909447667,36.2841776398386,1.04199651903841));
#30102=CARTESIAN_POINT('Ctrl Pts',(38.3697226472005,32.2327602036007,0.884996391686153));
#30103=CARTESIAN_POINT('Ctrl Pts',(34.5509630471873,30.6629539550025,0.727996264333901));
#30104=CARTESIAN_POINT('Ctrl Pts',(31.1345139786991,32.9818140634986,0.570996136981646));
#30105=CARTESIAN_POINT('Ctrl Pts',(31.1849789200754,37.1112158757118,0.413996009629392));
#30106=CARTESIAN_POINT('Ctrl Pts',(34.6550079471686,39.3458268431676,0.256995882277139));
#30107=CARTESIAN_POINT('Ctrl Pts',(38.4372231849787,37.6868217065119,0.0999957549248859));
#30108=CARTESIAN_POINT('Ctrl Pts',(39.1314848156243,33.611627523338,-0.0570043724273679));
#30109=CARTESIAN_POINT('Ctrl Pts',(37.1325959372044,31.7372591159268,-0.161671123995537));
#30110=CARTESIAN_POINT('Ctrl Pts',(35.9563385206894,31.4227955987545,-0.214004499779622));
#30111=CARTESIAN_POINT('Ctrl Pts',(37.9552630411254,37.5267093987114,8.21400449977962));
#30112=CARTESIAN_POINT('Ctrl Pts',(38.7860963780679,36.5549589254462,8.16167112399554));
#30113=CARTESIAN_POINT('Ctrl Pts',(39.4009732488241,33.744049865601,8.05700437242737));
#30114=CARTESIAN_POINT('Ctrl Pts',(36.37629757881,30.6305236834712,7.90000424507512));
#30115=CARTESIAN_POINT('Ctrl Pts',(32.1165942698471,31.4445388603786,7.74300411772287));
#30116=CARTESIAN_POINT('Ctrl Pts',(30.4429364274986,35.4422074306354,7.58600399037061));
#30117=CARTESIAN_POINT('Ctrl Pts',(32.8554054932919,39.0456002474389,7.42900386301836));
#30118=CARTESIAN_POINT('Ctrl Pts',(37.1910702102687,39.020145495151,7.2720037356661));
#30119=CARTESIAN_POINT('Ctrl Pts',(39.561923078043,35.3903430207689,7.11500360831385));
#30120=CARTESIAN_POINT('Ctrl Pts',(37.8420846273271,31.4102406249626,6.95800348096159));
#30121=CARTESIAN_POINT('Ctrl Pts',(33.5737072973814,30.6492466703945,6.80100335360934));
#30122=CARTESIAN_POINT('Ctrl Pts',(30.5843074279779,33.789547088263,6.64400322625708));
#30123=CARTESIAN_POINT('Ctrl Pts',(31.5544979211211,38.0153059312343,6.48700309890484));
#30124=CARTESIAN_POINT('Ctrl Pts',(35.6143049344472,39.5371942999712,6.33000297155258));
#30125=CARTESIAN_POINT('Ctrl Pts',(39.1232579504846,36.9905453090318,6.17300284420033));
#30126=CARTESIAN_POINT('Ctrl Pts',(38.9348464369457,32.6589511253872,6.01600271684807));
#30127=CARTESIAN_POINT('Ctrl Pts',(35.2180201601081,30.4265999701529,5.85900258949582));
#30128=CARTESIAN_POINT('Ctrl Pts',(31.3056932203567,32.2952594827172,5.70200246214357));
#30129=CARTESIAN_POINT('Ctrl Pts',(30.7060865587576,36.5892862685565,5.54500233479131));
#30130=CARTESIAN_POINT('Ctrl Pts',(33.956873300029,39.4581845606676,5.38800220743906));
#30131=CARTESIAN_POINT('Ctrl Pts',(38.1430417474823,38.3293861113103,5.2310020800868));
#30132=CARTESIAN_POINT('Ctrl Pts',(39.5108145134353,34.2150951337324,5.07400195273456));
#30133=CARTESIAN_POINT('Ctrl Pts',(36.8336966271993,30.8046359103087,4.9170018253823));
#30134=CARTESIAN_POINT('Ctrl Pts',(32.512285385248,31.1561998994534,4.76000169803005));
#30135=CARTESIAN_POINT('Ctrl Pts',(30.4216317036192,34.9545363220374,4.60300157067779));
#30136=CARTESIAN_POINT('Ctrl Pts',(32.4364447966046,38.7936404570559,4.44600144332554));
#30137=CARTESIAN_POINT('Ctrl Pts',(36.750022433952,39.2309508015887,4.28900131597329));
#30138=CARTESIAN_POINT('Ctrl Pts',(39.4943381658426,35.8743269714277,4.13200118862103));
#30139=CARTESIAN_POINT('Ctrl Pts',(38.2085377477941,31.7336857587036,3.97500106126878));
#30140=CARTESIAN_POINT('Ctrl Pts',(34.0456107497072,30.5219798611747,3.81800093391652));
#30141=CARTESIAN_POINT('Ctrl Pts',(30.738493748942,33.3257575831257,3.66100080656427));
#30142=CARTESIAN_POINT('Ctrl Pts',(31.252710285337,37.6308445407701,3.50400067921202));
#30143=CARTESIAN_POINT('Ctrl Pts',(35.1271574611734,39.5768279624082,3.34700055185977));
#30144=CARTESIAN_POINT('Ctrl Pts',(38.8875813167745,37.4187258362905,3.19000042450751));
#30145=CARTESIAN_POINT('Ctrl Pts',(39.1619737197485,33.0917290601617,3.03300029715526));
#30146=CARTESIAN_POINT('Ctrl Pts',(35.7042843401251,30.4758971195542,2.876000169803));
#30147=CARTESIAN_POINT('Ctrl Pts',(31.6150564762743,31.9168716811727,2.71900004245075));
#30148=CARTESIAN_POINT('Ctrl Pts',(30.5611398629031,36.1225168896708,2.5619999150985));
#30149=CARTESIAN_POINT('Ctrl Pts',(33.48759188202,39.3215906252928,2.40499978774624));
#30150=CARTESIAN_POINT('Ctrl Pts',(37.7702344413602,38.6454522028303,2.24799966039399));
#30151=CARTESIAN_POINT('Ctrl Pts',(39.568781862737,34.7004025928096,2.09099953304174));
#30152=CARTESIAN_POINT('Ctrl Pts',(37.2704574229183,31.0240032892043,1.93399940568949));
#30153=CARTESIAN_POINT('Ctrl Pts',(32.9361947180972,30.9129215291889,1.77699927833723));
#30154=CARTESIAN_POINT('Ctrl Pts',(30.4525605927511,34.4667558983969,1.61999915098498));
#30155=CARTESIAN_POINT('Ctrl Pts',(32.0466699232375,38.4987681546272,1.46299902363272));
#30156=CARTESIAN_POINT('Ctrl Pts',(36.2890366767668,39.3933756787425,1.30599889628047));
#30157=CARTESIAN_POINT('Ctrl Pts',(39.3755561844741,36.3484529936443,1.14899876892822));
#30158=CARTESIAN_POINT('Ctrl Pts',(38.5383832036972,32.0942549754603,0.991998641575964));
#30159=CARTESIAN_POINT('Ctrl Pts',(34.5284879564222,30.4458771578634,0.834998514223711));
#30160=CARTESIAN_POINT('Ctrl Pts',(30.9410395917123,32.8808003010019,0.677998386871457));
#30161=CARTESIAN_POINT('Ctrl Pts',(30.9940303923319,37.2168859506,0.520998259519203));
#30162=CARTESIAN_POINT('Ctrl Pts',(34.6377404869918,39.5633431347282,0.36399813216695));
#30163=CARTESIAN_POINT('Ctrl Pts',(38.6092622623382,37.8213018675437,0.206998004814697));
#30164=CARTESIAN_POINT('Ctrl Pts',(39.3382729110006,33.5421370343408,0.0499978774624429));
#30165=CARTESIAN_POINT('Ctrl Pts',(37.2393361218455,31.5739531851941,-0.0546688741057264));
#30166=CARTESIAN_POINT('Ctrl Pts',(36.0042049488753,31.243750214851,-0.107002249889811));
#30167=CARTESIAN_POINT('Ctrl Pts',(38.0961285948024,37.6471475165633,8.32100674966943));
#30168=CARTESIAN_POINT('Ctrl Pts',(38.9665644295237,36.6290775899881,8.26867337388535));
#30169=CARTESIAN_POINT('Ctrl Pts',(39.6107500181967,33.6841837526321,8.16400662231718));
#30170=CARTESIAN_POINT('Ctrl Pts',(36.441900172476,30.4222482467195,8.00700649496493));
#30171=CARTESIAN_POINT('Ctrl Pts',(31.9791538664038,31.2750642670716,7.85000636761267));
#30172=CARTESIAN_POINT('Ctrl Pts',(30.2257194575204,35.4632856878632,7.69300624026042));
#30173=CARTESIAN_POINT('Ctrl Pts',(32.753181262015,39.238437809064,7.53600611290817));
#30174=CARTESIAN_POINT('Ctrl Pts',(37.2955097522044,39.2117697306779,7.37900598555592));
#30175=CARTESIAN_POINT('Ctrl Pts',(39.7793716811886,35.4089491092894,7.22200585820366));
#30176=CARTESIAN_POINT('Ctrl Pts',(37.9775554192851,31.2391311721338,7.06500573085141));
#30177=CARTESIAN_POINT('Ctrl Pts',(33.5057216363881,30.441863683446,6.90800560349916));
#30178=CARTESIAN_POINT('Ctrl Pts',(30.3738290474178,33.7318496456872,6.75100547614689));
#30179=CARTESIAN_POINT('Ctrl Pts',(31.3902646358661,38.1590334890178,6.59400534879465));
#30180=CARTESIAN_POINT('Ctrl Pts',(35.6435863904507,39.7534641813021,6.43700522144238));
#30181=CARTESIAN_POINT('Ctrl Pts',(39.3197971438036,37.085426632005,6.28000509409014));
#30182=CARTESIAN_POINT('Ctrl Pts',(39.122404807981,32.5473627011697,6.12300496673788));
#30183=CARTESIAN_POINT('Ctrl Pts',(35.2284123079944,30.2086043066787,5.96600483938564));
#30184=CARTESIAN_POINT('Ctrl Pts',(31.1296004114509,32.1663353344374,5.80900471203338));
#30185=CARTESIAN_POINT('Ctrl Pts',(30.5014129016501,36.6650411800673,5.65200458468112));
#30186=CARTESIAN_POINT('Ctrl Pts',(33.9071516278456,39.6706883641509,5.49500445732887));
#30187=CARTESIAN_POINT('Ctrl Pts',(38.2928579600589,38.4880846134226,5.33800432997661));
#30188=CARTESIAN_POINT('Ctrl Pts',(39.72582697599,34.1776818622125,5.18100420262437));
#30189=CARTESIAN_POINT('Ctrl Pts',(36.9211016016709,30.6046597061106,5.0240040752721));
#30190=CARTESIAN_POINT('Ctrl Pts',(32.3937059925777,30.9729813426439,4.86700394791986));
#30191=CARTESIAN_POINT('Ctrl Pts',(30.2033992227766,34.9523692505858,4.7100038205676));
#30192=CARTESIAN_POINT('Ctrl Pts',(32.3142503868067,38.9744681045439,4.55300369321535));
#30193=CARTESIAN_POINT('Ctrl Pts',(36.833438994737,39.4326232818222,4.39600356586309));
#30194=CARTESIAN_POINT('Ctrl Pts',(39.7085652668935,35.9160026365752,4.23900343851085));
#30195=CARTESIAN_POINT('Ctrl Pts',(38.3614758924016,31.5779936400392,4.08200331115859));
#30196=CARTESIAN_POINT('Ctrl Pts',(34.0001188363665,30.3085305751198,3.92500318380634));
#30197=CARTESIAN_POINT('Ctrl Pts',(30.5353648128034,33.2459531522644,3.76800305645408));
#30198=CARTESIAN_POINT('Ctrl Pts',(31.0740919921095,37.7562463637945,3.61100292910183));
#30199=CARTESIAN_POINT('Ctrl Pts',(35.1332185480963,39.7949870216991,3.45400280174957));
#30200=CARTESIAN_POINT('Ctrl Pts',(39.0728867488228,37.5340168101838,3.29700267439732));
#30201=CARTESIAN_POINT('Ctrl Pts',(39.360358338736,33.0007694268683,3.14000254704507));
#30202=CARTESIAN_POINT('Ctrl Pts',(35.7378547540399,30.2602512537625,2.98300241969282));
#30203=CARTESIAN_POINT('Ctrl Pts',(31.4537097748133,31.7699113017935,2.82600229234056));
#30204=CARTESIAN_POINT('Ctrl Pts',(30.3495571772993,36.1760227742485,2.66900216498831));
#30205=CARTESIAN_POINT('Ctrl Pts',(33.415501444059,39.52758354292,2.51200203763605));
#30206=CARTESIAN_POINT('Ctrl Pts',(37.902280422705,38.8192163097165,2.3550019102838));
#30207=CARTESIAN_POINT('Ctrl Pts',(39.7865573966804,34.6861219842625,2.19800178293155));
#30208=CARTESIAN_POINT('Ctrl Pts',(37.3786810353442,30.8344834494167,2.0410016555793));
#30209=CARTESIAN_POINT('Ctrl Pts',(32.8378213856151,30.7181068667712,1.88400152822704));
#30210=CARTESIAN_POINT('Ctrl Pts',(30.2358023681867,34.4413382876556,1.72700140087479));
#30211=CARTESIAN_POINT('Ctrl Pts',(31.9058965062304,38.6655404203885,1.57000127352254));
#30212=CARTESIAN_POINT('Ctrl Pts',(36.3504798927025,39.6027903023767,1.41300114617028));
#30213=CARTESIAN_POINT('Ctrl Pts',(39.5841214241815,36.41272834745,1.25600101881803));
#30214=CARTESIAN_POINT('Ctrl Pts',(38.7070437601939,31.9557497473198,1.09900089146578));
#30215=CARTESIAN_POINT('Ctrl Pts',(34.5060128656572,30.2288003607244,0.942000764113522));
#30216=CARTESIAN_POINT('Ctrl Pts',(30.7475652047255,32.7797865385051,0.785000636761267));
#30217=CARTESIAN_POINT('Ctrl Pts',(30.8030818645885,37.3225560254883,0.628000509409015));
#30218=CARTESIAN_POINT('Ctrl Pts',(34.620473026815,39.7808594262888,0.47100038205676));
#30219=CARTESIAN_POINT('Ctrl Pts',(38.7813013396977,37.9557820285754,0.314000254704507));
#30220=CARTESIAN_POINT('Ctrl Pts',(39.5450610063768,33.4726465453437,0.157000127352254));
#30221=CARTESIAN_POINT('Ctrl Pts',(37.3460763064866,31.4106472544613,0.0523333757840845));
#30222=CARTESIAN_POINT('Ctrl Pts',(36.0520713770613,31.0647048309474,0.));
#30223=CARTESIAN_POINT('Ctrl Pts',(36.0520713770613,31.0647048309474,0.));
#30224=CARTESIAN_POINT('Ctrl Pts',(36.1681792227746,31.1043194052127,-1.93406836379874E-16));
#30225=CARTESIAN_POINT('Ctrl Pts',(36.2820220087194,31.1494844117486,-1.00024874895392E-15));
#30226=CARTESIAN_POINT('Ctrl Pts',(36.3933738437048,31.1998422365254,-1.16573417585641E-15));
#30227=CARTESIAN_POINT('Ctrl Pts',(36.5072229375308,31.2513294232309,-1.33493090168249E-15));
#30228=CARTESIAN_POINT('Ctrl Pts',(36.6184687230184,31.3082454542348,-1.64395861563978E-15));
#30229=CARTESIAN_POINT('Ctrl Pts',(36.7268454950609,31.3702566870239,-9.99200722162641E-16));
#30230=CARTESIAN_POINT('Ctrl Pts',(36.8407839045068,31.435450188349,-3.21355391692774E-16));
#30231=CARTESIAN_POINT('Ctrl Pts',(36.9515522547681,31.5062756815887,8.02288849704332E-16));
#30232=CARTESIAN_POINT('Ctrl Pts',(37.058802639455,31.5823916741173,9.99200722162641E-16));
#30233=CARTESIAN_POINT('Ctrl Pts',(37.1526467260561,31.6489931675798,1.17149861056366E-15));
#30234=CARTESIAN_POINT('Ctrl Pts',(37.2437970657742,31.7196462572752,8.48680262035355E-16));
#30235=CARTESIAN_POINT('Ctrl Pts',(37.3319890907744,31.7941443117117,9.99200722162641E-16));
#30236=CARTESIAN_POINT('Ctrl Pts',(37.3493641971328,31.8088215075162,1.02885543304851E-15));
#30237=CARTESIAN_POINT('Ctrl Pts',(37.3666243754182,31.8236479962496,-1.0299785826125E-15));
#30238=CARTESIAN_POINT('Ctrl Pts',(37.3837674478979,31.8386222687341,-1.0547118733939E-15));
#30239=CARTESIAN_POINT('Ctrl Pts',(37.3963017832026,31.8495708634207,-1.07279587555905E-15));
#30240=CARTESIAN_POINT('Ctrl Pts',(37.4087723034701,31.8605974704649,-2.60456824673694E-15));
#30241=CARTESIAN_POINT('Ctrl Pts',(37.4211693573137,31.8716933759855,-2.4980018054066E-15));
#30242=CARTESIAN_POINT('Ctrl Pts',(37.5137485970205,31.954555845562,-1.70218045614906E-15));
#30243=CARTESIAN_POINT('Ctrl Pts',(37.6023719888639,32.0414000295362,-2.33877871405102E-15));
#30244=CARTESIAN_POINT('Ctrl Pts',(37.6867781087441,32.1319050017937,-1.99840144432528E-15));
#30245=CARTESIAN_POINT('Ctrl Pts',(37.7709925191637,32.2222044124232,-1.65879726478403E-15));
#30246=CARTESIAN_POINT('Ctrl Pts',(37.8510093104121,32.3161487056446,-9.47721428060247E-16));
#30247=CARTESIAN_POINT('Ctrl Pts',(37.9265284067741,32.4134511741487,-1.30451205393456E-15));
#30248=CARTESIAN_POINT('Ctrl Pts',(38.0010152019123,32.5094235756611,-1.65642556372184E-15));
#30249=CARTESIAN_POINT('Ctrl Pts',(38.0711268225993,32.6086636566059,-6.10757404334397E-16));
#30250=CARTESIAN_POINT('Ctrl Pts',(38.1365292929227,32.710917134839,-5.27355936696949E-16));
#30251=CARTESIAN_POINT('Ctrl Pts',(38.1898350382321,32.7942579909372,-4.59380256721482E-16));
#30252=CARTESIAN_POINT('Ctrl Pts',(38.2400117946351,32.8796011515617,-1.29327937900734E-15));
#30253=CARTESIAN_POINT('Ctrl Pts',(38.28685279593,32.9668147810226,-1.63757896132211E-15));
#30254=CARTESIAN_POINT('Ctrl Pts',(38.298752249944,32.9889704682297,-1.72504457763057E-15));
#30255=CARTESIAN_POINT('Ctrl Pts',(38.3104363019817,33.0112468837781,3.54805112116964E-15));
#30256=CARTESIAN_POINT('Ctrl Pts',(38.3219012991264,33.0336418915139,3.66373598126302E-15));
#30257=CARTESIAN_POINT('Ctrl Pts',(38.3300587509266,33.0495761472196,3.74604683213415E-15));
#30258=CARTESIAN_POINT('Ctrl Pts',(38.3381015974855,33.0655632618739,-7.08373702740619E-16));
#30259=CARTESIAN_POINT('Ctrl Pts',(38.3460261690062,33.0815968043693,-6.93889390390723E-16));
#30260=CARTESIAN_POINT('Ctrl Pts',(38.3989870883303,33.1887510080204,-5.97088888833881E-16));
#30261=CARTESIAN_POINT('Ctrl Pts',(38.4467091567301,33.2980550637735,1.26900815615077E-15));
#30262=CARTESIAN_POINT('Ctrl Pts',(38.4889135757351,33.409246351529,1.0547118733939E-15));
#30263=CARTESIAN_POINT('Ctrl Pts',(38.5302818373033,33.5182347083035,8.44661246299018E-16));
#30264=CARTESIAN_POINT('Ctrl Pts',(38.5663491876186,33.6290368908256,3.13106813660632E-16));
#30265=CARTESIAN_POINT('Ctrl Pts',(38.5968048600256,33.7414193655312,4.9960036108132E-16));
#30266=CARTESIAN_POINT('Ctrl Pts',(38.6012591757497,33.7578559431745,5.26876105632901E-16));
#30267=CARTESIAN_POINT('Ctrl Pts',(38.6055933637529,33.7743263394091,3.42924457172855E-16));
#30268=CARTESIAN_POINT('Ctrl Pts',(38.6098063577125,33.7908298367184,3.33066907387547E-16));
#30269=CARTESIAN_POINT('Ctrl Pts',(38.6394749188516,33.9070500410733,3.19833619294622E-16));
#30270=CARTESIAN_POINT('Ctrl Pts',(38.6631375043611,34.0249121336904,2.13657224701249E-16));
#30271=CARTESIAN_POINT('Ctrl Pts',(38.6808849682855,34.1439802784308,6.10622663543836E-16));
#30272=CARTESIAN_POINT('Ctrl Pts',(38.6908685193634,34.2109601528418,8.33929201973265E-16));
#30273=CARTESIAN_POINT('Ctrl Pts',(38.6989793099884,34.2783216258907,1.0776972087123E-15));
#30274=CARTESIAN_POINT('Ctrl Pts',(38.705226464765,34.3459856591442,1.13797860024079E-15));
#30275=CARTESIAN_POINT('Ctrl Pts',(38.7081089504882,34.3772063695005,1.1657929023787E-15));
#30276=CARTESIAN_POINT('Ctrl Pts',(38.7105946047039,34.4084914721069,9.83922849187538E-16));
#30277=CARTESIAN_POINT('Ctrl Pts',(38.7126839762627,34.4398330679179,1.02695629777827E-15));
#30278=CARTESIAN_POINT('Ctrl Pts',(38.7138850693151,34.4578500514573,1.05169444256127E-15));
#30279=CARTESIAN_POINT('Ctrl Pts',(38.7149546915907,34.4758786502346,-4.64302084245928E-16));
#30280=CARTESIAN_POINT('Ctrl Pts',(38.715892912359,34.4939090237972,-4.44089209850063E-16));
#30281=CARTESIAN_POINT('Ctrl Pts',(38.7222038666684,34.6151905681615,-3.08127044991787E-16));
#30282=CARTESIAN_POINT('Ctrl Pts',(38.7225822971166,34.7366693867671,-2.99144274726584E-15));
#30283=CARTESIAN_POINT('Ctrl Pts',(38.7171864105867,34.8578982328034,-2.05391259555654E-15));
#30284=CARTESIAN_POINT('Ctrl Pts',(38.71190245704,34.9766122916381,-1.13583069320137E-15));
#30285=CARTESIAN_POINT('Ctrl Pts',(38.7010807679502,35.0950875649844,1.78168855748587E-15));
#30286=CARTESIAN_POINT('Ctrl Pts',(38.6848165352731,35.2128980770419,1.76247905159244E-15));
#30287=CARTESIAN_POINT('Ctrl Pts',(38.6687112067838,35.3295575613132,1.74345722568323E-15));
#30288=CARTESIAN_POINT('Ctrl Pts',(38.6472688142291,35.4455660470931,1.26625388930718E-16));
#30289=CARTESIAN_POINT('Ctrl Pts',(38.62053500354,35.5604910223212,1.80411241501588E-16));
#30290=CARTESIAN_POINT('Ctrl Pts',(38.6031281268642,35.6353207910372,2.15432201045671E-16));
#30291=CARTESIAN_POINT('Ctrl Pts',(38.5834769893052,35.7096907862118,1.51379352364637E-15));
#30292=CARTESIAN_POINT('Ctrl Pts',(38.5615843902035,35.7834747121961,1.2490009027033E-15));
#30293=CARTESIAN_POINT('Ctrl Pts',(38.5541960332861,35.8083754550181,1.15963817406959E-15));
#30294=CARTESIAN_POINT('Ctrl Pts',(38.5465523248095,35.8332093935643,2.32778305945499E-15));
#30295=CARTESIAN_POINT('Ctrl Pts',(38.5386531847276,35.8579714965102,2.3037127760972E-15));
#30296=CARTESIAN_POINT('Ctrl Pts',(38.5335667575399,35.8739163502969,2.28821339990993E-15));
#30297=CARTESIAN_POINT('Ctrl Pts',(38.528375210839,35.8898288067619,1.8799349255917E-16));
#30298=CARTESIAN_POINT('Ctrl Pts',(38.5230814037796,35.9056994997334,2.77555756156289E-16));
#30299=CARTESIAN_POINT('Ctrl Pts',(38.4861837480683,36.016317691632,9.0180169672523E-16));
#30300=CARTESIAN_POINT('Ctrl Pts',(38.4442853792632,36.1250244064477,1.67610385059537E-15));
#30301=CARTESIAN_POINT('Ctrl Pts',(38.3974510894444,36.2314004501635,1.54737334057131E-15));
#30302=CARTESIAN_POINT('Ctrl Pts',(38.3593370450265,36.3179699544917,1.44261162867242E-15));
#30303=CARTESIAN_POINT('Ctrl Pts',(38.3179530965748,36.4029957144323,1.09861093914672E-15));
#30304=CARTESIAN_POINT('Ctrl Pts',(38.27331318169,36.4862361414904,1.49186218934005E-15));
#30305=CARTESIAN_POINT('Ctrl Pts',(38.2516982037212,36.526541773829,1.68227736219745E-15));
#30306=CARTESIAN_POINT('Ctrl Pts',(38.2293195714479,36.5664285801089,1.70359564472489E-15));
#30307=CARTESIAN_POINT('Ctrl Pts',(38.2061773939932,36.6058676078699,1.76247905159244E-15));
#30308=CARTESIAN_POINT('Ctrl Pts',(38.1925910511184,36.629021529097,1.79704840691352E-15));
#30309=CARTESIAN_POINT('Ctrl Pts',(38.1787394785284,36.652024183054,3.81993764399042E-15));
#30310=CARTESIAN_POINT('Ctrl Pts',(38.1646367510805,36.6748472188681,3.75394160201381E-15));
#30311=CARTESIAN_POINT('Ctrl Pts',(38.1062052960737,36.7694092952617,3.48050195910614E-15));
#30312=CARTESIAN_POINT('Ctrl Pts',(38.0434225704545,36.8609661715359,-8.52927663010733E-16));
#30313=CARTESIAN_POINT('Ctrl Pts',(37.9763226192313,36.9491271397218,-6.21031004399697E-16));
#30314=CARTESIAN_POINT('Ctrl Pts',(37.9162919198372,37.0279999925776,-4.13565598690696E-16));
#30315=CARTESIAN_POINT('Ctrl Pts',(37.8528051248739,37.1041547391556,2.13873726282784E-15));
#30316=CARTESIAN_POINT('Ctrl Pts',(37.7858631238401,37.1772850733286,2.38004060904018E-15));
#30317=CARTESIAN_POINT('Ctrl Pts',(37.7510082002317,37.215362097793,2.52360662668101E-15));
#30318=CARTESIAN_POINT('Ctrl Pts',(37.71521617243,37.2526187144799,1.78459625189646E-16));
#30319=CARTESIAN_POINT('Ctrl Pts',(37.6785244495408,37.2890395253442,2.4980018054066E-16));
#30320=CARTESIAN_POINT('Ctrl Pts',(37.6735319337713,37.2858331630076,8.));
#30321=CARTESIAN_POINT('Ctrl Pts',(37.7506743707736,37.2087205217211,8.));
#30322=CARTESIAN_POINT('Ctrl Pts',(37.8237044431802,37.1279857045437,8.));
#30323=CARTESIAN_POINT('Ctrl Pts',(37.8926298478593,37.044047215584,8.));
#30324=CARTESIAN_POINT('Ctrl Pts',(37.9633151675467,36.957965473245,8.));
#30325=CARTESIAN_POINT('Ctrl Pts',(38.0296839050274,36.8685139150261,8.));
#30326=CARTESIAN_POINT('Ctrl Pts',(38.0917144885261,36.7760977905708,8.));
#30327=CARTESIAN_POINT('Ctrl Pts',(38.1550361362519,36.681758176998,8.));
#30328=CARTESIAN_POINT('Ctrl Pts',(38.213837583624,36.5843287225808,8.));
#30329=CARTESIAN_POINT('Ctrl Pts',(38.2680590919843,36.4842010613249,8.));
#30330=CARTESIAN_POINT('Ctrl Pts',(38.3198483094818,36.3885649681376,8.));
#30331=CARTESIAN_POINT('Ctrl Pts',(38.367459260449,36.2904664802624,8.));
#30332=CARTESIAN_POINT('Ctrl Pts',(38.4108043761726,36.1902222494829,8.));
#30333=CARTESIAN_POINT('Ctrl Pts',(38.4178413961439,36.1739477363751,8.));
#30334=CARTESIAN_POINT('Ctrl Pts',(38.4247659020623,36.1576166279166,8.));
#30335=CARTESIAN_POINT('Ctrl Pts',(38.4315774256463,36.1412302363951,8.));
#30336=CARTESIAN_POINT('Ctrl Pts',(38.4380879567714,36.1255679384209,8.));
#30337=CARTESIAN_POINT('Ctrl Pts',(38.444492253249,36.1098623247479,8.));
#30338=CARTESIAN_POINT('Ctrl Pts',(38.4507880993566,36.0941200527897,8.));
#30339=CARTESIAN_POINT('Ctrl Pts',(38.4941733303702,35.9856386677758,8.));
#30340=CARTESIAN_POINT('Ctrl Pts',(38.5324447107219,35.8753402935035,8.));
#30341=CARTESIAN_POINT('Ctrl Pts',(38.5655736281431,35.7636567372894,8.));
#30342=CARTESIAN_POINT('Ctrl Pts',(38.5991370998293,35.6505082202659,8.));
#30343=CARTESIAN_POINT('Ctrl Pts',(38.6274227108421,35.5359371924552,8.));
#30344=CARTESIAN_POINT('Ctrl Pts',(38.6503580685478,35.4203601525596,8.));
#30345=CARTESIAN_POINT('Ctrl Pts',(38.6743329744418,35.2995445677074,8.));
#30346=CARTESIAN_POINT('Ctrl Pts',(38.6924624153241,35.1776288913195,8.));
#30347=CARTESIAN_POINT('Ctrl Pts',(38.7046079739425,35.0550654857614,8.));
#30348=CARTESIAN_POINT('Ctrl Pts',(38.7137171429063,34.9631429315928,8.));
#30349=CARTESIAN_POINT('Ctrl Pts',(38.7194592548969,34.8708554330634,8.));
#30350=CARTESIAN_POINT('Ctrl Pts',(38.7217527860176,34.7783903770868,8.));
#30351=CARTESIAN_POINT('Ctrl Pts',(38.7223003505608,34.7563149905001,8.));
#30352=CARTESIAN_POINT('Ctrl Pts',(38.7226511975219,34.7342249565511,8.));
#30353=CARTESIAN_POINT('Ctrl Pts',(38.7228041151383,34.7121518890107,8.));
#30354=CARTESIAN_POINT('Ctrl Pts',(38.7236388754478,34.5916574611757,8.));
#30355=CARTESIAN_POINT('Ctrl Pts',(38.7185854897377,34.4715178604479,8.));
#30356=CARTESIAN_POINT('Ctrl Pts',(38.7075750014661,34.3521591261975,8.));
#30357=CARTESIAN_POINT('Ctrl Pts',(38.6966351615249,34.2335662521979,8.));
#30358=CARTESIAN_POINT('Ctrl Pts',(38.6798146688512,34.1157433795803,8.));
#30359=CARTESIAN_POINT('Ctrl Pts',(38.6569964506754,33.9990955538343,8.));
#30360=CARTESIAN_POINT('Ctrl Pts',(38.6541228094095,33.9844053618549,8.));
#30361=CARTESIAN_POINT('Ctrl Pts',(38.6511539769623,33.9697337993248,8.));
#30362=CARTESIAN_POINT('Ctrl Pts',(38.6480896603102,33.9550816715453,8.));
#30363=CARTESIAN_POINT('Ctrl Pts',(38.6241791602958,33.840752853322,8.));
#30364=CARTESIAN_POINT('Ctrl Pts',(38.5944594648021,33.7276067766126,8.));
#30365=CARTESIAN_POINT('Ctrl Pts',(38.5592367168361,33.6159099315205,8.));
#30366=CARTESIAN_POINT('Ctrl Pts',(38.5372714828272,33.5462547375853,8.));
#30367=CARTESIAN_POINT('Ctrl Pts',(38.5131650961288,33.4771632221397,8.));
#30368=CARTESIAN_POINT('Ctrl Pts',(38.4869819486326,33.4087021985955,8.));
#30369=CARTESIAN_POINT('Ctrl Pts',(38.4780327050517,33.385302629251,8.));
#30370=CARTESIAN_POINT('Ctrl Pts',(38.4688407862625,33.3619767358619,8.));
#30371=CARTESIAN_POINT('Ctrl Pts',(38.4594085763077,33.3387272549231,8.));
#30372=CARTESIAN_POINT('Ctrl Pts',(38.4526591454727,33.3220905638083,8.));
#30373=CARTESIAN_POINT('Ctrl Pts',(38.4457861267366,33.3054918782784,8.));
#30374=CARTESIAN_POINT('Ctrl Pts',(38.438797464252,33.2889485050412,8.));
#30375=CARTESIAN_POINT('Ctrl Pts',(38.3928761431039,33.180244792853,8.));
#30376=CARTESIAN_POINT('Ctrl Pts',(38.3419017974374,33.073767495779,8.));
#30377=CARTESIAN_POINT('Ctrl Pts',(38.2862328647479,32.9697709587171,8.));
#30378=CARTESIAN_POINT('Ctrl Pts',(38.2286487527766,32.8621966269402,8.));
#30379=CARTESIAN_POINT('Ctrl Pts',(38.1660413106006,32.757275993628,8.));
#30380=CARTESIAN_POINT('Ctrl Pts',(38.0987518751312,32.6552979021095,8.));
#30381=CARTESIAN_POINT('Ctrl Pts',(38.0308292899206,32.5523602632,8.));
#30382=CARTESIAN_POINT('Ctrl Pts',(37.9581357532083,32.4524200570822,8.));
#30383=CARTESIAN_POINT('Ctrl Pts',(37.8809718147757,32.3557926317859,8.));
#30384=CARTESIAN_POINT('Ctrl Pts',(37.8265588287192,32.2876547573834,8.));
#30385=CARTESIAN_POINT('Ctrl Pts',(37.7699218575833,32.221164530513,8.));
#30386=CARTESIAN_POINT('Ctrl Pts',(37.7111532334385,32.156441009698,8.));
#30387=CARTESIAN_POINT('Ctrl Pts',(37.6849201407301,32.1275497748485,8.));
#30388=CARTESIAN_POINT('Ctrl Pts',(37.6582621737227,32.0990106723795,8.));
#30389=CARTESIAN_POINT('Ctrl Pts',(37.6311869343715,32.0708348649218,8.));
#30390=CARTESIAN_POINT('Ctrl Pts',(37.6195644247842,32.0587399176506,8.));
#30391=CARTESIAN_POINT('Ctrl Pts',(37.6078664443942,32.0467134553255,8.));
#30392=CARTESIAN_POINT('Ctrl Pts',(37.5961000985213,32.0347627427216,8.));
#30393=CARTESIAN_POINT('Ctrl Pts',(37.5076578370054,31.9449346804806,8.));
#30394=CARTESIAN_POINT('Ctrl Pts',(37.4152562466455,31.8592792534028,8.));
#30395=CARTESIAN_POINT('Ctrl Pts',(37.3192240628069,31.7781146097001,8.));
#30396=CARTESIAN_POINT('Ctrl Pts',(37.2371844701374,31.7087762478888,8.));
#30397=CARTESIAN_POINT('Ctrl Pts',(37.1524942030697,31.6427153977926,8.));
#30398=CARTESIAN_POINT('Ctrl Pts',(37.0653339993003,31.5801479843188,8.));
#30399=CARTESIAN_POINT('Ctrl Pts',(37.026223350155,31.552072646602,8.));
#30400=CARTESIAN_POINT('Ctrl Pts',(36.9866151034059,31.5247009668187,8.));
#30401=CARTESIAN_POINT('Ctrl Pts',(36.9465243462331,31.4980538108418,8.));
#30402=CARTESIAN_POINT('Ctrl Pts',(36.9192915198287,31.4799529461023,8.));
#30403=CARTESIAN_POINT('Ctrl Pts',(36.891830409748,31.4621830185383,8.));
#30404=CARTESIAN_POINT('Ctrl Pts',(36.8641757039143,31.4447693408987,8.));
#30405=CARTESIAN_POINT('Ctrl Pts',(36.7573714959831,31.3775166259847,8.));
#30406=CARTESIAN_POINT('Ctrl Pts',(36.6476205511297,31.3155307102762,8.));
#30407=CARTESIAN_POINT('Ctrl Pts',(36.53522484258,31.2591452484686,8.));
#30408=CARTESIAN_POINT('Ctrl Pts',(36.4331310435836,31.2079279370747,8.));
#30409=CARTESIAN_POINT('Ctrl Pts',(36.328854296794,31.161331443821,8.));
#30410=CARTESIAN_POINT('Ctrl Pts',(36.2225975660985,31.1196349359533,8.));
#30411=CARTESIAN_POINT('Ctrl Pts',(36.1671670804927,31.0978833004188,8.));
#30412=CARTESIAN_POINT('Ctrl Pts',(36.1111974373468,31.0774656305418,8.));
#30413=CARTESIAN_POINT('Ctrl Pts',(36.0547327596422,31.0583698145405,8.));
#30414=CARTESIAN_POINT('Ctrl Pts',(31.4836963557363,34.997016753135,6.38741669750802));
#30415=CARTESIAN_POINT('Ctrl Pts',(31.4810522497149,34.6831064242593,6.4016107071645));
#30416=CARTESIAN_POINT('Ctrl Pts',(31.5197088623892,34.3698361384337,6.41580471682098));
#30417=CARTESIAN_POINT('Ctrl Pts',(31.602283311232,34.0686052256029,6.42999872647746));
#30418=CARTESIAN_POINT('Ctrl Pts',(31.9067356658548,32.9579655303736,6.48233210226155));
#30419=CARTESIAN_POINT('Ctrl Pts',(32.8082071426114,32.0109890873326,6.53466547804563));
#30420=CARTESIAN_POINT('Ctrl Pts',(33.9025202849968,31.6522420135335,6.58699885382972));
#30421=CARTESIAN_POINT('Ctrl Pts',(34.9968334273823,31.2934949397344,6.6393322296138));
#30422=CARTESIAN_POINT('Ctrl Pts',(36.2839882353967,31.5229772351772,6.69166560539789));
#30423=CARTESIAN_POINT('Ctrl Pts',(37.1868794441274,32.2378302684166,6.74399898118197));
#30424=CARTESIAN_POINT('Ctrl Pts',(38.089770652858,32.952683301656,6.79633235696606));
#30425=CARTESIAN_POINT('Ctrl Pts',(38.6083982623049,34.1529070726919,6.84866573275014));
#30426=CARTESIAN_POINT('Ctrl Pts',(38.5102396094692,35.3003133216048,6.90099910853422));
#30427=CARTESIAN_POINT('Ctrl Pts',(38.4120809566336,36.4477195705176,6.95333248431831));
#30428=CARTESIAN_POINT('Ctrl Pts',(37.6971360415154,37.5423082973073,7.00566586010239));
#30429=CARTESIAN_POINT('Ctrl Pts',(36.6859407221977,38.0934406773841,7.05799923588648));
#30430=CARTESIAN_POINT('Ctrl Pts',(35.67474540288,38.6445730574609,7.11033261167056));
#30431=CARTESIAN_POINT('Ctrl Pts',(34.3672996793629,38.6522490908248,7.16266598745465));
#30432=CARTESIAN_POINT('Ctrl Pts',(33.3498295528725,38.1127747395053,7.21499936323873));
#30433=CARTESIAN_POINT('Ctrl Pts',(32.3323594263822,37.5733003881858,7.26733273902282));
#30434=CARTESIAN_POINT('Ctrl Pts',(31.6048648969186,36.4866756521828,7.3196661148069));
#30435=CARTESIAN_POINT('Ctrl Pts',(31.4934684170666,35.3406028059835,7.37199949059098));
#30436=CARTESIAN_POINT('Ctrl Pts',(31.4825294286169,35.2280599532493,7.37713855956333));
#30437=CARTESIAN_POINT('Ctrl Pts',(31.4775314630746,35.1149438434099,7.38227762853567));
#30438=CARTESIAN_POINT('Ctrl Pts',(31.47826034488,35.0017653187145,7.38741669750802));
#30439=CARTESIAN_POINT('Ctrl Pts',(33.9479286229388,31.0647048309474,8.));
#30440=CARTESIAN_POINT('Ctrl Pts',(32.6539236935135,31.4106472544613,7.94766662421592));
#30441=CARTESIAN_POINT('Ctrl Pts',(30.454936822078,33.4726324908028,7.84299987264775));
#30442=CARTESIAN_POINT('Ctrl Pts',(31.2187005389846,37.9557872897229,7.6859997452955));
#30443=CARTESIAN_POINT('Ctrl Pts',(35.3795268052061,39.7808547962683,7.52899961794324));
#30444=CARTESIAN_POINT('Ctrl Pts',(39.1969168896572,37.3225573472918,7.37199949059099));
#30445=CARTESIAN_POINT('Ctrl Pts',(39.2524338890068,32.7797860374403,7.21499936323873));
#30446=CARTESIAN_POINT('Ctrl Pts',(35.4939868648458,30.2288021766129,7.05799923588648));
#30447=CARTESIAN_POINT('Ctrl Pts',(31.2929572874421,31.9557502059188,6.90099910853422));
#30448=CARTESIAN_POINT('Ctrl Pts',(30.4158796925061,36.4127281597254,6.74399898118197));
#30449=CARTESIAN_POINT('Ctrl Pts',(33.6495204900336,39.6027890266495,6.58699885382972));
#30450=CARTESIAN_POINT('Ctrl Pts',(38.0941026784935,38.6655395297167,6.42999872647747));
#30451=CARTESIAN_POINT('Ctrl Pts',(39.7641964207046,34.4413384042963,6.27299859912521));
#30452=CARTESIAN_POINT('Ctrl Pts',(37.1621780526355,30.7181079801836,6.11599847177296));
#30453=CARTESIAN_POINT('Ctrl Pts',(32.6213195789955,30.8344845112897,5.95899834442071));
#30454=CARTESIAN_POINT('Ctrl Pts',(30.2134438300848,34.686122068773,5.80199821706845));
#30455=CARTESIAN_POINT('Ctrl Pts',(32.0977203234525,38.8192153272012,5.6449980897162));
#30456=CARTESIAN_POINT('Ctrl Pts',(36.5844981485848,39.5275823816942,5.48799796236394));
#30457=CARTESIAN_POINT('Ctrl Pts',(39.6504416291735,36.1760224717832,5.33099783501169));
#30458=CARTESIAN_POINT('Ctrl Pts',(38.5462893146292,31.7699121313011,5.17399770765944));
#30459=CARTESIAN_POINT('Ctrl Pts',(34.2621454354683,30.2602524703801,5.01699758030718));
#30460=CARTESIAN_POINT('Ctrl Pts',(30.6396427805907,33.0007699401812,4.85999745295493));
#30461=CARTESIAN_POINT('Ctrl Pts',(30.927114296777,37.5340161596205,4.70299732560268));
#30462=CARTESIAN_POINT('Ctrl Pts',(34.86678148609,39.7949857907703,4.54599719825042));
#30463=CARTESIAN_POINT('Ctrl Pts',(38.9259070000539,37.7562456562111,4.38899707089817));
#30464=CARTESIAN_POINT('Ctrl Pts',(39.4646340410498,33.2459536025622,4.23199694354592));
#30465=CARTESIAN_POINT('Ctrl Pts',(35.9998809069499,30.3085317794917,4.07499681619366));
#30466=CARTESIAN_POINT('Ctrl Pts',(31.6385249705421,31.5779945185253,3.91799668884141));
#30467=CARTESIAN_POINT('Ctrl Pts',(30.291435941871,35.9160024014201,3.76099656148915));
#30468=CARTESIAN_POINT('Ctrl Pts',(33.1665614759356,39.4326221439007,3.60399643413691));
#30469=CARTESIAN_POINT('Ctrl Pts',(37.6857489237188,38.9744670842276,3.44699630678464));
#30470=CARTESIAN_POINT('Ctrl Pts',(39.7965995458586,34.9523692628263,3.2899961794324));
#30471=CARTESIAN_POINT('Ctrl Pts',(37.6062933383462,30.9729823764193,3.13299605208014));
#30472=CARTESIAN_POINT('Ctrl Pts',(33.078898891504,30.6046608345122,2.97599592472789));
#30473=CARTESIAN_POINT('Ctrl Pts',(30.2741742372111,34.1776820732232,2.81899579737563));
#30474=CARTESIAN_POINT('Ctrl Pts',(31.7071428852578,38.4880837181509,2.66199567002338));
#30475=CARTESIAN_POINT('Ctrl Pts',(36.0928480916297,39.6706871647746,2.50499554267113));
#30476=CARTESIAN_POINT('Ctrl Pts',(39.4985859434327,36.6650407532663,2.34799541531887));
#30477=CARTESIAN_POINT('Ctrl Pts',(38.8703985950797,32.1663360606625,2.19099528796662));
#30478=CARTESIAN_POINT('Ctrl Pts',(34.7715877503781,30.208605539026,2.03399516061437));
#30479=CARTESIAN_POINT('Ctrl Pts',(30.8775962508689,32.547363326415,1.87699503326212));
#30480=CARTESIAN_POINT('Ctrl Pts',(30.6802039639638,37.0854261049008,1.71999490590986));
#30481=CARTESIAN_POINT('Ctrl Pts',(34.3564137772933,39.7534629455386,1.56299477855761));
#30482=CARTESIAN_POINT('Ctrl Pts',(38.6097344321268,38.159032706872,1.40599465120535));
#30483=CARTESIAN_POINT('Ctrl Pts',(39.6261697761982,33.7318499178854,1.2489945238531));
#30484=CARTESIAN_POINT('Ctrl Pts',(36.4942779564007,30.441864951573,1.09199439650085));
#30485=CARTESIAN_POINT('Ctrl Pts',(32.0224453946446,31.2391319593762,0.934994269148593));
#30486=CARTESIAN_POINT('Ctrl Pts',(30.2206294419397,35.4089493247815,0.77799414179634));
#30487=CARTESIAN_POINT('Ctrl Pts',(32.7044910542971,39.2117680815463,0.620994014444087));
#30488=CARTESIAN_POINT('Ctrl Pts',(37.246817707304,39.2384377086451,0.463993887091833));
#30489=CARTESIAN_POINT('Ctrl Pts',(39.7742802645754,35.4632838929154,0.30699375973958));
#30490=CARTESIAN_POINT('Ctrl Pts',(38.0208433725288,31.2750679875305,0.149993632387326));
#30491=CARTESIAN_POINT('Ctrl Pts',(33.5581043558821,30.4222449751611,-0.00700649496492684));
#30492=CARTESIAN_POINT('Ctrl Pts',(30.3892402311535,33.6841941049532,-0.164006622317179));
#30493=CARTESIAN_POINT('Ctrl Pts',(31.0334355704763,36.629077589988,-0.26867337388535));
#30494=CARTESIAN_POINT('Ctrl Pts',(31.9038714051976,37.6471475165632,-0.321006749669435));
#30495=CARTESIAN_POINT('Ctrl Pts',(33.9957950511247,31.243750214851,8.10700224988981));
#30496=CARTESIAN_POINT('Ctrl Pts',(32.7606638781546,31.573953185194,8.05466887410573));
#30497=CARTESIAN_POINT('Ctrl Pts',(30.6617250162538,33.5421236192438,7.95000212253755));
#30498=CARTESIAN_POINT('Ctrl Pts',(31.3907395308691,37.8213068893232,7.79300199518531));
#30499=CARTESIAN_POINT('Ctrl Pts',(35.3622593526719,39.5633387153612,7.63600186783305));
#30500=CARTESIAN_POINT('Ctrl Pts',(39.0059684185923,37.2168872122651,7.4790017404808));
#30501=CARTESIAN_POINT('Ctrl Pts',(39.0589595432527,32.8807998227341,7.32200161312854));
#30502=CARTESIAN_POINT('Ctrl Pts',(35.4715117863422,30.4458788911338,7.16500148577629));
#30503=CARTESIAN_POINT('Ctrl Pts',(31.4616177962741,32.0942554131942,7.00800135842404));
#30504=CARTESIAN_POINT('Ctrl Pts',(30.6244448814073,36.3484528144607,6.85100123107178));
#30505=CARTESIAN_POINT('Ctrl Pts',(33.7109636885558,39.3933744610575,6.69400110371954));
#30506=CARTESIAN_POINT('Ctrl Pts',(37.9533292985792,38.4987673044786,6.53700097636727));
#30507=CARTESIAN_POINT('Ctrl Pts',(39.5474382512424,34.4667560097307,6.38000084901502));
#30508=CARTESIAN_POINT('Ctrl Pts',(37.0638047457115,30.9129225919439,6.22300072166277));
#30509=CARTESIAN_POINT('Ctrl Pts',(32.7295431634706,31.0240043027649,6.06600059431052));
#30510=CARTESIAN_POINT('Ctrl Pts',(30.4312193082136,34.7004026734751,5.90900046695826));
#30511=CARTESIAN_POINT('Ctrl Pts',(32.2297662708491,38.6454512650169,5.75200033960601));
#30512=CARTESIAN_POINT('Ctrl Pts',(36.5124077291574,39.3215895168996,5.59500021225375));
#30513=CARTESIAN_POINT('Ctrl Pts',(39.4388589978718,36.1225166009669,5.4380000849015));
#30514=CARTESIAN_POINT('Ctrl Pts',(38.3849426545962,31.9168724729398,5.28099995754925));
#30515=CARTESIAN_POINT('Ctrl Pts',(34.295715840761,30.4758982808191,5.12399983019699));
#30516=CARTESIAN_POINT('Ctrl Pts',(30.8380273486519,33.0917295501202,4.96699970284475));
#30517=CARTESIAN_POINT('Ctrl Pts',(31.1124196812533,37.4187252153261,4.80999957549248));
#30518=CARTESIAN_POINT('Ctrl Pts',(34.8728425714575,39.5768267874833,4.65299944814023));
#30519=CARTESIAN_POINT('Ctrl Pts',(38.7472887526802,37.6308438653799,4.49599932078798));
#30520=CARTESIAN_POINT('Ctrl Pts',(39.2615051570579,33.3257580129361,4.33899919343573));
#30521=CARTESIAN_POINT('Ctrl Pts',(35.9543890052876,30.5219810107509,4.18199906608348));
#30522=CARTESIAN_POINT('Ctrl Pts',(31.7914630758879,31.7336865972209,4.02499893873122));
#30523=CARTESIAN_POINT('Ctrl Pts',(30.5056629879263,35.8743267469715,3.86799881137897));
#30524=CARTESIAN_POINT('Ctrl Pts',(33.2499780153063,39.2309497154396,3.71099868402671));
#30525=CARTESIAN_POINT('Ctrl Pts',(37.5635545452901,38.7936394831613,3.55399855667446));
#30526=CARTESIAN_POINT('Ctrl Pts',(39.5783671210399,34.954536333721,3.39699842932221));
#30527=CARTESIAN_POINT('Ctrl Pts',(37.4877139761171,31.1562008861948,3.23999830196995));
#30528=CARTESIAN_POINT('Ctrl Pts',(33.1663038435374,30.804636987371,3.0829981746177));
#30529=CARTESIAN_POINT('Ctrl Pts',(30.4891866445685,34.2150953351428,2.92599804726545));
#30530=CARTESIAN_POINT('Ctrl Pts',(31.8569590593748,38.3293852567711,2.76899791991319));
#30531=CARTESIAN_POINT('Ctrl Pts',(36.0431264322094,39.4581834158598,2.61199779256094));
#30532=CARTESIAN_POINT('Ctrl Pts',(39.2939123388708,36.5892858611738,2.45499766520869));
#30533=CARTESIAN_POINT('Ctrl Pts',(38.6943058313741,32.295260175901,2.29799753785643));
#30534=CARTESIAN_POINT('Ctrl Pts',(34.7819798956087,30.4266011464317,2.14099741050418));
#30535=CARTESIAN_POINT('Ctrl Pts',(31.0651545737294,32.6589517221855,1.98399728315193));
#30536=CARTESIAN_POINT('Ctrl Pts',(30.8767431068824,36.9905448059094,1.82699715579967));
#30537=CARTESIAN_POINT('Ctrl Pts',(34.3856952256649,39.5371931204316,1.66999702844742));
#30538=CARTESIAN_POINT('Ctrl Pts',(38.4455011892756,38.015305184674,1.51299690109516));
#30539=CARTESIAN_POINT('Ctrl Pts',(39.4156914491603,33.789547348077,1.35599677374291));
#30540=CARTESIAN_POINT('Ctrl Pts',(36.4262923139345,30.6492478808251,1.19899664639066));
#30541=CARTESIAN_POINT('Ctrl Pts',(32.1579161495709,31.4102413763875,1.0419965190384));
#30542=CARTESIAN_POINT('Ctrl Pts',(30.438077993986,35.3903432264567,0.884996391686151));
#30543=CARTESIAN_POINT('Ctrl Pts',(32.8089305595391,39.0201439210504,0.727996264333897));
#30544=CARTESIAN_POINT('Ctrl Pts',(37.1445935229203,39.0456001515887,0.570996136981644));
#30545=CARTESIAN_POINT('Ctrl Pts',(39.5570633072411,35.4422057173529,0.413996009629391));
#30546=CARTESIAN_POINT('Ctrl Pts',(37.8834030947066,31.4445424115665,0.256995882277137));
#30547=CARTESIAN_POINT('Ctrl Pts',(33.6237067435201,30.63052056076,0.0999957549248841));
#30548=CARTESIAN_POINT('Ctrl Pts',(30.5990174441545,33.7440597469193,-0.0570043724273687));
#30549=CARTESIAN_POINT('Ctrl Pts',(31.2139036219321,36.5549589254462,-0.161671123995539));
#30550=CARTESIAN_POINT('Ctrl Pts',(32.0447369588746,37.5267093987113,-0.214004499779624));
#30551=CARTESIAN_POINT('Ctrl Pts',(34.0436614793107,31.4227955987545,8.21400449977962));
#30552=CARTESIAN_POINT('Ctrl Pts',(32.8674040627957,31.7372591159268,8.16167112399554));
#30553=CARTESIAN_POINT('Ctrl Pts',(30.8685132104295,33.6116147476849,8.05700437242736));
#30554=CARTESIAN_POINT('Ctrl Pts',(31.5627785227536,37.6868264889233,7.90000424507513));
#30555=CARTESIAN_POINT('Ctrl Pts',(35.3449919001376,39.3458226344541,7.74300411772285));
#30556=CARTESIAN_POINT('Ctrl Pts',(38.8150199475273,37.1112170772383,7.58600399037062));
#30557=CARTESIAN_POINT('Ctrl Pts',(38.8654851974986,32.9818136080279,7.42900386301834));
#30558=CARTESIAN_POINT('Ctrl Pts',(35.4490367078385,30.6629556056548,7.27200373566611));
#30559=CARTESIAN_POINT('Ctrl Pts',(31.6302783051062,32.2327606204696,7.11500360831384));
#30560=CARTESIAN_POINT('Ctrl Pts',(30.8330100703084,36.284177469196,6.9580034809616));
#30561=CARTESIAN_POINT('Ctrl Pts',(33.7724068870781,39.1839598954654,6.80100335360933));
#30562=CARTESIAN_POINT('Ctrl Pts',(37.812555918665,38.3319950792405,6.64400322625709));
#30563=CARTESIAN_POINT('Ctrl Pts',(39.3306800817804,34.4921736151651,6.48700309890483));
#30564=CARTESIAN_POINT('Ctrl Pts',(36.9654314387874,31.1077372037044,6.33000297155258));
#30565=CARTESIAN_POINT('Ctrl Pts',(32.8377667479458,31.2135240942401,6.17300284420033));
#30566=CARTESIAN_POINT('Ctrl Pts',(30.6489947863424,34.7146832781773,6.01600271684807));
#30567=CARTESIAN_POINT('Ctrl Pts',(32.3618122182458,38.4716872028325,5.85900258949582));
#30568=CARTESIAN_POINT('Ctrl Pts',(36.4403173097299,39.1155966521051,5.70200246214356));
#30569=CARTESIAN_POINT('Ctrl Pts',(39.2272763665704,36.0690107301504,5.54500233479131));
#30570=CARTESIAN_POINT('Ctrl Pts',(38.2235959945632,32.0638328145787,5.38800220743906));
#30571=CARTESIAN_POINT('Ctrl Pts',(34.3292862460537,30.6915440912579,5.2310020800868));
#30572=CARTESIAN_POINT('Ctrl Pts',(31.0364119167131,33.1826891600592,5.07400195273456));
#30573=CARTESIAN_POINT('Ctrl Pts',(31.2977250657295,37.3034342710318,4.9170018253823));
#30574=CARTESIAN_POINT('Ctrl Pts',(34.8789036568251,39.3586677841964,4.76000169803004));
#30575=CARTESIAN_POINT('Ctrl Pts',(38.5686705053066,37.5054420745486,4.60300157067779));
#30576=CARTESIAN_POINT('Ctrl Pts',(39.0583762730659,33.4055624233101,4.44600144332554));
#30577=CARTESIAN_POINT('Ctrl Pts',(35.9088971036253,30.7354302420101,4.28900131597329));
#30578=CARTESIAN_POINT('Ctrl Pts',(31.9444011812337,31.8893786759165,4.13200118862103));
#30579=CARTESIAN_POINT('Ctrl Pts',(30.7198900339817,35.8326510925229,3.97500106126878));
#30580=CARTESIAN_POINT('Ctrl Pts',(33.333394554677,39.0292772869785,3.81800093391652));
#30581=CARTESIAN_POINT('Ctrl Pts',(37.4413601668615,38.6128118820951,3.66100080656427));
#30582=CARTESIAN_POINT('Ctrl Pts',(39.3601346962212,34.9567034046157,3.50400067921202));
#30583=CARTESIAN_POINT('Ctrl Pts',(37.3691346138881,31.3394193959702,3.34700055185976));
#30584=CARTESIAN_POINT('Ctrl Pts',(33.2537087955707,31.0046131402298,3.19000042450751));
#30585=CARTESIAN_POINT('Ctrl Pts',(30.7041990519258,34.2525085970623,3.03300029715526));
#30586=CARTESIAN_POINT('Ctrl Pts',(32.0067752334918,38.1706867953913,2.876000169803));
#30587=CARTESIAN_POINT('Ctrl Pts',(35.9934047727891,39.2456796669448,2.71900004245075));
#30588=CARTESIAN_POINT('Ctrl Pts',(39.0892387343089,36.5135309690814,2.5619999150985));
#30589=CARTESIAN_POINT('Ctrl Pts',(38.5182130676685,32.4241842911394,2.40499978774624));
#30590=CARTESIAN_POINT('Ctrl Pts',(34.7923720408392,30.6445967538374,2.24799966039399));
#30591=CARTESIAN_POINT('Ctrl Pts',(31.25271289659,32.770540117956,2.09099953304174));
#30592=CARTESIAN_POINT('Ctrl Pts',(31.0732822498009,36.8956635069179,1.93399940568948));
#30593=CARTESIAN_POINT('Ctrl Pts',(34.4149766740365,39.3209232953247,1.77699927833723));
#30594=CARTESIAN_POINT('Ctrl Pts',(38.2812679464245,37.8715776624759,1.61999915098497));
#30595=CARTESIAN_POINT('Ctrl Pts',(39.2052131221224,33.8472447782685,1.46299902363272));
#30596=CARTESIAN_POINT('Ctrl Pts',(36.3583066714682,30.8566308100772,1.30599889628047));
#30597=CARTESIAN_POINT('Ctrl Pts',(32.2933869044973,31.5813507933988,1.14899876892822));
#30598=CARTESIAN_POINT('Ctrl Pts',(30.6555265460323,35.3717371281319,0.991998641575962));
#30599=CARTESIAN_POINT('Ctrl Pts',(32.9133700647812,38.8285197605545,0.834998514223708));
#30600=CARTESIAN_POINT('Ctrl Pts',(37.0423693385366,38.8527625945324,0.677998386871455));
#30601=CARTESIAN_POINT('Ctrl Pts',(39.3398463499068,35.4211275417905,0.520998259519202));
#30602=CARTESIAN_POINT('Ctrl Pts',(37.7459628168843,31.6140168356026,0.363998132166948));
#30603=CARTESIAN_POINT('Ctrl Pts',(33.6893091311581,30.8387961463588,0.206998004814695));
#30604=CARTESIAN_POINT('Ctrl Pts',(30.8087946571555,33.8039253888853,0.0499978774624422));
#30605=CARTESIAN_POINT('Ctrl Pts',(31.3943716733878,36.4808402609044,-0.0546688741057282));
#30606=CARTESIAN_POINT('Ctrl Pts',(32.1856025125517,37.4062712808594,-0.107002249889813));
#30607=CARTESIAN_POINT('Ctrl Pts',(34.0915279074966,31.601840982658,8.32100674966943));
#30608=CARTESIAN_POINT('Ctrl Pts',(32.9741442474368,31.9005650466595,8.26867337388535));
#30609=CARTESIAN_POINT('Ctrl Pts',(31.0753014046052,33.6811058761259,8.16400662231717));
#30610=CARTESIAN_POINT('Ctrl Pts',(31.7348175146381,37.5523460885235,8.00700649496493));
#30611=CARTESIAN_POINT('Ctrl Pts',(35.3277244476034,39.128306553547,7.85000636761267));
#30612=CARTESIAN_POINT('Ctrl Pts',(38.6240714764623,37.0055469422116,7.69300624026043));
#30613=CARTESIAN_POINT('Ctrl Pts',(38.6720108517446,33.0828273933217,7.53600611290816));
#30614=CARTESIAN_POINT('Ctrl Pts',(35.4265616293347,30.8800323201757,7.37900598555592));
#30615=CARTESIAN_POINT('Ctrl Pts',(31.7989388139383,32.371265827745,7.22200585820365));
#30616=CARTESIAN_POINT('Ctrl Pts',(31.0415752592096,36.2199021239313,7.06500573085141));
#30617=CARTESIAN_POINT('Ctrl Pts',(33.8338500856003,38.9745453298735,6.90800560349915));
#30618=CARTESIAN_POINT('Ctrl Pts',(37.6717825387507,38.1652228540024,6.75100547614691));
#30619=CARTESIAN_POINT('Ctrl Pts',(39.1139219123182,34.5175912205995,6.59400534879464));
#30620=CARTESIAN_POINT('Ctrl Pts',(36.8670581318634,31.3025518154648,6.4370052214424));
#30621=CARTESIAN_POINT('Ctrl Pts',(32.9459903324209,31.4030438857154,6.28000509409014));
#30622=CARTESIAN_POINT('Ctrl Pts',(30.8667702644712,34.7289638828794,6.12300496673789));
#30623=CARTESIAN_POINT('Ctrl Pts',(32.4938581656424,38.2979231406482,5.96600483938563));
#30624=CARTESIAN_POINT('Ctrl Pts',(36.3682268903025,38.9096037873106,5.80900471203337));
#30625=CARTESIAN_POINT('Ctrl Pts',(39.0156937352688,36.0155048593341,5.65200458468113));
#30626=CARTESIAN_POINT('Ctrl Pts',(38.0622493345301,32.2107931562174,5.49500445732887));
#30627=CARTESIAN_POINT('Ctrl Pts',(34.3628566513464,30.9071899016968,5.33800432997662));
#30628=CARTESIAN_POINT('Ctrl Pts',(31.2347964847743,33.2736487699982,5.18100420262436));
#30629=CARTESIAN_POINT('Ctrl Pts',(31.4830304502057,37.1881433267374,5.02400407527211));
#30630=CARTESIAN_POINT('Ctrl Pts',(34.8849647421926,39.1405087809095,4.86700394791985));
#30631=CARTESIAN_POINT('Ctrl Pts',(38.3900522579329,37.3800402837173,4.71000382056761));
#30632=CARTESIAN_POINT('Ctrl Pts',(38.855247389074,33.4853668336842,4.55300369321535));
#30633=CARTESIAN_POINT('Ctrl Pts',(35.863405201963,30.9488794732692,4.3960035658631));
#30634=CARTESIAN_POINT('Ctrl Pts',(32.0973392865795,32.0450707546122,4.23900343851084));
#30635=CARTESIAN_POINT('Ctrl Pts',(30.9341170800371,35.7909754380742,4.08200331115859));
#30636=CARTESIAN_POINT('Ctrl Pts',(33.4168110940477,38.8276048585174,3.92500318380633));
#30637=CARTESIAN_POINT('Ctrl Pts',(37.3191657884328,38.4319842810288,3.76800305645409));
#30638=CARTESIAN_POINT('Ctrl Pts',(39.1419022714024,34.9588704755104,3.61100292910183));
#30639=CARTESIAN_POINT('Ctrl Pts',(37.250555251659,31.5226379057457,3.45400280174958));
#30640=CARTESIAN_POINT('Ctrl Pts',(33.3411137476041,31.2045892930886,3.29700267439732));
#30641=CARTESIAN_POINT('Ctrl Pts',(30.9192114592832,34.2899218589819,3.14000254704507));
#30642=CARTESIAN_POINT('Ctrl Pts',(32.1565914076088,38.0119883340115,2.98300241969281));
#30643=CARTESIAN_POINT('Ctrl Pts',(35.9436831133688,39.0331759180299,2.82600229234056));
#30644=CARTESIAN_POINT('Ctrl Pts',(38.884565129747,36.4377760769889,2.66900216498831));
#30645=CARTESIAN_POINT('Ctrl Pts',(38.3421203039629,32.5531084063779,2.51200203763606));
#30646=CARTESIAN_POINT('Ctrl Pts',(34.8027641860698,30.8625923612432,2.3550019102838));
#30647=CARTESIAN_POINT('Ctrl Pts',(31.4402712194505,32.8821285137264,2.19800178293155));
#30648=CARTESIAN_POINT('Ctrl Pts',(31.2698213927195,36.8007822079265,2.04100165557929));
#30649=CARTESIAN_POINT('Ctrl Pts',(34.4442581224081,39.1046534702177,1.88400152822704));
#30650=CARTESIAN_POINT('Ctrl Pts',(38.1170347035733,37.7278501402779,1.72700140087479));
#30651=CARTESIAN_POINT('Ctrl Pts',(38.9947347950846,33.90494220846,1.57000127352253));
#30652=CARTESIAN_POINT('Ctrl Pts',(36.290321029002,31.0640137393293,1.41300114617028));
#30653=CARTESIAN_POINT('Ctrl Pts',(32.4288576594237,31.7524602104101,1.25600101881803));
#30654=CARTESIAN_POINT('Ctrl Pts',(30.8729750980786,35.353131029807,1.09900089146577));
#30655=CARTESIAN_POINT('Ctrl Pts',(33.0178095700233,38.6368956000587,0.94200076411352));
#30656=CARTESIAN_POINT('Ctrl Pts',(36.9401451541529,38.6599250374761,0.785000636761265));
#30657=CARTESIAN_POINT('Ctrl Pts',(39.1226293925725,35.400049366228,0.628000509409013));
#30658=CARTESIAN_POINT('Ctrl Pts',(37.6085225390622,31.7834912596387,0.471000382056759));
#30659=CARTESIAN_POINT('Ctrl Pts',(33.754911518796,31.0470717319576,0.314000254704506));
#30660=CARTESIAN_POINT('Ctrl Pts',(31.0185718701565,33.8637910308514,0.157000127352253));
#30661=CARTESIAN_POINT('Ctrl Pts',(31.5748397248436,36.4067215963626,0.0523333757840826));
#30662=CARTESIAN_POINT('Ctrl Pts',(32.3264680662287,37.2858331630075,-2.22044604925031E-15));
#30663=CARTESIAN_POINT('Ctrl Pts',(32.3264680662287,37.2858331630075,-2.16493489801906E-15));
#30664=CARTESIAN_POINT('Ctrl Pts',(32.2493253814486,37.208720274039,-2.02930540817935E-15));
#30665=CARTESIAN_POINT('Ctrl Pts',(32.1762950504991,37.1279852253981,-2.22088175559797E-15));
#30666=CARTESIAN_POINT('Ctrl Pts',(32.1073693836416,37.0440465177293,-2.44249065417534E-15));
#30667=CARTESIAN_POINT('Ctrl Pts',(32.0366838276613,36.957964590773,-2.66975792514024E-15));
#30668=CARTESIAN_POINT('Ctrl Pts',(31.9703148460741,36.8685128644539,-1.62037951577862E-15));
#30669=CARTESIAN_POINT('Ctrl Pts',(31.9082840182324,36.7760965840633,-1.60982338570648E-15));
#30670=CARTESIAN_POINT('Ctrl Pts',(31.8449621738338,36.681756889908,-1.59904755618531E-15));
#30671=CARTESIAN_POINT('Ctrl Pts',(31.7861605220008,36.5843273727301,-2.0500807145436E-15));
#30672=CARTESIAN_POINT('Ctrl Pts',(31.7319388093681,36.4841996609406,-1.27675647831893E-15));
#30673=CARTESIAN_POINT('Ctrl Pts',(31.6801495481474,36.3885637990409,-5.38124499843711E-16));
#30674=CARTESIAN_POINT('Ctrl Pts',(31.6325385292086,36.2904655679991,-4.81778164441647E-15));
#30675=CARTESIAN_POINT('Ctrl Pts',(31.5891933275412,36.1902216120283,-5.77315972805081E-15));
#30676=CARTESIAN_POINT('Ctrl Pts',(31.5821551531175,36.1739445059149,-5.92828918493564E-15));
#30677=CARTESIAN_POINT('Ctrl Pts',(31.5752295287451,36.1576107865788,-2.14687895786075E-15));
#30678=CARTESIAN_POINT('Ctrl Pts',(31.5684169229622,36.1412217669136,-2.1094237467878E-15));
#30679=CARTESIAN_POINT('Ctrl Pts',(31.5619076362096,36.1255624388982,-2.07363616168158E-15));
#30680=CARTESIAN_POINT('Ctrl Pts',(31.5555045468442,36.1098598194457,-5.01667023260332E-15));
#30681=CARTESIAN_POINT('Ctrl Pts',(31.5492098653947,36.0941205526839,-4.94049245958195E-15));
#30682=CARTESIAN_POINT('Ctrl Pts',(31.5058243818098,35.9856391775398,-4.41544452070402E-15));
#30683=CARTESIAN_POINT('Ctrl Pts',(31.4675527596774,35.875340817696,2.70422581427715E-15));
#30684=CARTESIAN_POINT('Ctrl Pts',(31.4344236193294,35.7636572747171,2.16493489801906E-15));
#30685=CARTESIAN_POINT('Ctrl Pts',(31.4008599589415,35.6505088963383,1.61857067083336E-15));
#30686=CARTESIAN_POINT('Ctrl Pts',(31.3725741668882,35.5359380090966,1.5704555898309E-16));
#30687=CARTESIAN_POINT('Ctrl Pts',(31.3496386440377,35.4203611044154,3.88578058618805E-16));
#30688=CARTESIAN_POINT('Ctrl Pts',(31.3256636190246,35.2995459305591,6.30604259909078E-16));
#30689=CARTESIAN_POINT('Ctrl Pts',(31.3075340503036,35.1776306642325,-4.77206768499493E-16));
#30690=CARTESIAN_POINT('Ctrl Pts',(31.2953883637021,35.0550676565495,-7.49400541621981E-16));
#30691=CARTESIAN_POINT('Ctrl Pts',(31.2862790987509,34.9631454007872,-9.53545871463847E-16));
#30692=CARTESIAN_POINT('Ctrl Pts',(31.2805368906832,34.8708581938176,-1.66063273915206E-15));
#30693=CARTESIAN_POINT('Ctrl Pts',(31.2782432669551,34.7783934177904,-1.83186799063151E-15));
#30694=CARTESIAN_POINT('Ctrl Pts',(31.2776956893352,34.7563184621811,-1.87274853712248E-15));
#30695=CARTESIAN_POINT('Ctrl Pts',(31.2773448230031,34.7342288592592,-1.15850189636716E-15));
#30696=CARTESIAN_POINT('Ctrl Pts',(31.2771918797387,34.7121562214804,-1.19348975147204E-15));
#30697=CARTESIAN_POINT('Ctrl Pts',(31.2763569642807,34.5916619548496,-1.38448803559665E-15));
#30698=CARTESIAN_POINT('Ctrl Pts',(31.2814102215213,34.471522491006,-2.99090776565717E-15));
#30699=CARTESIAN_POINT('Ctrl Pts',(31.2924206159431,34.3521638613563,-2.66453525910038E-15));
#30700=CARTESIAN_POINT('Ctrl Pts',(31.3033603504718,34.2335712231593,-2.34025726846702E-15));
#30701=CARTESIAN_POINT('Ctrl Pts',(31.3201807588279,34.1157485527733,3.70943136885229E-16));
#30702=CARTESIAN_POINT('Ctrl Pts',(31.342998921253,33.9991008864625,6.93889390390723E-16));
#30703=CARTESIAN_POINT('Ctrl Pts',(31.3458725738232,33.9844106208813,7.34560296054722E-16));
#30704=CARTESIAN_POINT('Ctrl Pts',(31.348841419242,33.9697389843081,-2.36384243829245E-16));
#30705=CARTESIAN_POINT('Ctrl Pts',(31.3519057505532,33.9550867820407,-2.22044604925031E-16));
#30706=CARTESIAN_POINT('Ctrl Pts',(31.3758162053254,33.8407581458576,-1.09500521307372E-16));
#30707=CARTESIAN_POINT('Ctrl Pts',(31.405535880703,33.7276122083523,-1.31284998081472E-15));
#30708=CARTESIAN_POINT('Ctrl Pts',(31.4407586285186,33.6159154648327,-2.41473507855972E-15));
#30709=CARTESIAN_POINT('Ctrl Pts',(31.4627238926124,33.5462602385377,-3.10188184234126E-15));
#30710=CARTESIAN_POINT('Ctrl Pts',(31.4868303230444,33.4771686776378,-2.63257088976062E-16));
#30711=CARTESIAN_POINT('Ctrl Pts',(31.5130135264214,33.4087075970126,-2.22044604925031E-16));
#30712=CARTESIAN_POINT('Ctrl Pts',(31.5219635139129,33.385306112999,-2.0795728293307E-16));
#30713=CARTESIAN_POINT('Ctrl Pts',(31.5311562173418,33.361978315516,-2.32755725796262E-15));
#30714=CARTESIAN_POINT('Ctrl Pts',(31.5405892520308,33.3387269417829,-2.58126853225349E-15));
#30715=CARTESIAN_POINT('Ctrl Pts',(31.5473379087033,33.3220922591317,-2.76278066918334E-15));
#30716=CARTESIAN_POINT('Ctrl Pts',(31.5542101234624,33.3054955734371,-8.17270399285879E-16));
#30717=CARTESIAN_POINT('Ctrl Pts',(31.5611979545174,33.288954186216,-7.7715611723761E-16));
#30718=CARTESIAN_POINT('Ctrl Pts',(31.6071192859873,33.1802505670847,-5.13540522049862E-16));
#30719=CARTESIAN_POINT('Ctrl Pts',(31.6580936513602,33.0737733268919,-1.22043518676627E-15));
#30720=CARTESIAN_POINT('Ctrl Pts',(31.713762608453,32.9697768155529,-8.60422844084496E-16));
#30721=CARTESIAN_POINT('Ctrl Pts',(31.7713468082815,32.8622023934125,-4.88024585443386E-16));
#30722=CARTESIAN_POINT('Ctrl Pts',(31.8339543542604,32.7572816421653,-1.6844387016455E-15));
#30723=CARTESIAN_POINT('Ctrl Pts',(31.9012439032021,32.6553034111749,-1.60982338570648E-15));
#30724=CARTESIAN_POINT('Ctrl Pts',(31.9691666425039,32.5523655715406,-1.53450594440749E-15));
#30725=CARTESIAN_POINT('Ctrl Pts',(32.0418603487199,32.4524251462352,-2.14412608245669E-16));
#30726=CARTESIAN_POINT('Ctrl Pts',(32.119024465224,32.3557974897081,-1.11022302462516E-16));
#30727=CARTESIAN_POINT('Ctrl Pts',(32.1734376325243,32.2876593825328,-3.81154351168831E-17));
#30728=CARTESIAN_POINT('Ctrl Pts',(32.2300747937192,32.2211689202647,2.3957932567246E-15));
#30729=CARTESIAN_POINT('Ctrl Pts',(32.2888436140898,32.1564451639975,2.85882428840978E-15));
#30730=CARTESIAN_POINT('Ctrl Pts',(32.3150756619651,32.1275550712175,3.06550279776831E-15));
#30731=CARTESIAN_POINT('Ctrl Pts',(32.3417325486905,32.0990170804093,1.33832078810492E-15));
#30732=CARTESIAN_POINT('Ctrl Pts',(32.3688066730543,32.0708423529797,1.58206781009085E-15));
#30733=CARTESIAN_POINT('Ctrl Pts',(32.3804284156068,32.0587481694606,1.68669779181855E-15));
#30734=CARTESIAN_POINT('Ctrl Pts',(32.3921256212299,32.0467224591722,5.62787663488911E-16));
#30735=CARTESIAN_POINT('Ctrl Pts',(32.4038911827787,32.0347724888588,5.27355936696949E-16));
#30736=CARTESIAN_POINT('Ctrl Pts',(32.4923334498706,31.9449440126051,2.61014017404201E-16));
#30737=CARTESIAN_POINT('Ctrl Pts',(32.584735051869,31.8592881592603,-7.81291389151021E-17));
#30738=CARTESIAN_POINT('Ctrl Pts',(32.6807672456031,31.778123082898,1.11022302462516E-16));
#30739=CARTESIAN_POINT('Ctrl Pts',(32.7628075187761,31.7087837834614,2.72614319871455E-16));
#30740=CARTESIAN_POINT('Ctrl Pts',(32.8474985084852,31.6427220447333,9.36044375735486E-16));
#30741=CARTESIAN_POINT('Ctrl Pts',(32.9346594679295,31.5801538004245,1.38777878078145E-16));
#30742=CARTESIAN_POINT('Ctrl Pts',(32.9737706916096,31.5520779208788,-2.18974819016821E-16));
#30743=CARTESIAN_POINT('Ctrl Pts',(33.0133795255453,31.5247057193814,-1.25086984652678E-15));
#30744=CARTESIAN_POINT('Ctrl Pts',(33.0534708815057,31.4980580630162,-1.7277845820729E-15));
#30745=CARTESIAN_POINT('Ctrl Pts',(33.0807055590029,31.479955898353,-2.0517601300469E-15));
#30746=CARTESIAN_POINT('Ctrl Pts',(33.1081685502538,31.462184715489,8.66601268491E-16));
#30747=CARTESIAN_POINT('Ctrl Pts',(33.1358251623594,31.4447698310871,9.5062846483529E-16));
#30748=CARTESIAN_POINT('Ctrl Pts',(33.2426295858021,31.377516955689,1.27512505265964E-15));
#30749=CARTESIAN_POINT('Ctrl Pts',(33.3523807267505,31.315530896685,3.7726686237795E-15));
#30750=CARTESIAN_POINT('Ctrl Pts',(33.4647766052556,31.2591453155976,2.97331603782425E-15));
#30751=CARTESIAN_POINT('Ctrl Pts',(33.5668702670808,31.2079280421183,2.24723218426034E-15));
#30752=CARTESIAN_POINT('Ctrl Pts',(33.6711468426795,31.1613315802118,-1.73124610826904E-15));
#30753=CARTESIAN_POINT('Ctrl Pts',(33.7774033647392,31.1196350998879,-2.12763834328555E-15));
#30754=CARTESIAN_POINT('Ctrl Pts',(33.8328339031569,31.0978834152884,-2.36077539403599E-15));
#30755=CARTESIAN_POINT('Ctrl Pts',(33.8888035920626,31.0774657030867,3.31895026664625E-16));
#30756=CARTESIAN_POINT('Ctrl Pts',(33.9452683089267,31.0583698510224,1.66533453693773E-16));
#30757=CARTESIAN_POINT('Ctrl Pts',(31.4846882532079,35.0028111988253,7.11258330249198));
#30758=CARTESIAN_POINT('Ctrl Pts',(31.4819571032991,35.3538027877235,7.09672411194513));
#30759=CARTESIAN_POINT('Ctrl Pts',(31.5304045241347,35.7040585316776,7.08086492139827));
#30760=CARTESIAN_POINT('Ctrl Pts',(31.6331816560628,36.037569942224,7.06500573085141));
#30761=CARTESIAN_POINT('Ctrl Pts',(31.9723335346732,37.138116525912,7.01267235506733));
#30762=CARTESIAN_POINT('Ctrl Pts',(32.9030918101368,38.0563309278927,6.96033897928324));
#30763=CARTESIAN_POINT('Ctrl Pts',(34.008126356727,38.3805510495713,6.90800560349915));
#30764=CARTESIAN_POINT('Ctrl Pts',(35.1131609033171,38.7047711712498,6.85567222771507));
#30765=CARTESIAN_POINT('Ctrl Pts',(36.3924717210339,38.4349970126261,6.80333885193099));
#30766=CARTESIAN_POINT('Ctrl Pts',(37.2724836921536,37.6921713277471,6.75100547614691));
#30767=CARTESIAN_POINT('Ctrl Pts',(38.1524956632732,36.9493456428681,6.69867210036282));
#30768=CARTESIAN_POINT('Ctrl Pts',(38.6332087877957,35.7334684317338,6.64633872457873));
#30769=CARTESIAN_POINT('Ctrl Pts',(38.4990880533145,34.5896899253109,6.59400534879465));
#30770=CARTESIAN_POINT('Ctrl Pts',(38.3649673188333,33.4459114188879,6.54167197301056));
#30771=CARTESIAN_POINT('Ctrl Pts',(37.6160127253483,32.3742316171763,6.48933859722648));
#30772=CARTESIAN_POINT('Ctrl Pts',(36.5880241286988,31.8551403946957,6.4370052214424));
#30773=CARTESIAN_POINT('Ctrl Pts',(35.5600355320492,31.336049172215,6.38467184565831));
#30774=CARTESIAN_POINT('Ctrl Pts',(34.2530129322351,31.3695465289652,6.33233846987422));
#30775=CARTESIAN_POINT('Ctrl Pts',(33.2529649543364,31.9406152068676,6.28000509409014));
#30776=CARTESIAN_POINT('Ctrl Pts',(32.2529169764377,32.51168388477,6.22767171830605));
#30777=CARTESIAN_POINT('Ctrl Pts',(31.5598436204544,33.6203238838247,6.17533834252197));
#30778=CARTESIAN_POINT('Ctrl Pts',(31.4844882593247,34.7694704263135,6.12300496673789));
#30779=CARTESIAN_POINT('Ctrl Pts',(31.4794861724725,34.8457507430058,6.11953107865592));
#30780=CARTESIAN_POINT('Ctrl Pts',(31.4772059369411,34.9222095437145,6.11605719057395));
#30781=CARTESIAN_POINT('Ctrl Pts',(31.4775764275568,34.998690818207,6.11258330249198));
#30782=CARTESIAN_POINT('Ctrl Pts',(33.9479286229388,31.0647048309474,8.));
#30783=CARTESIAN_POINT('Ctrl Pts',(33.8318204903556,31.1043195030892,8.));
#30784=CARTESIAN_POINT('Ctrl Pts',(33.7179774196666,31.1494845762766,8.));
#30785=CARTESIAN_POINT('Ctrl Pts',(33.6066253055996,31.1998424449166,8.));
#30786=CARTESIAN_POINT('Ctrl Pts',(33.4927760432216,31.2513296236524,8.));
#30787=CARTESIAN_POINT('Ctrl Pts',(33.3815300897553,31.3082456117247,8.));
#30788=CARTESIAN_POINT('Ctrl Pts',(33.2731531534421,31.3702567766217,8.));
#30789=CARTESIAN_POINT('Ctrl Pts',(33.1592147882362,31.4354500824416,8.));
#30790=CARTESIAN_POINT('Ctrl Pts',(33.0484464742462,31.5062753311388,8.));
#30791=CARTESIAN_POINT('Ctrl Pts',(32.9411961197039,31.5823910435948,8.));
#30792=CARTESIAN_POINT('Ctrl Pts',(32.8473520594793,31.6489922919938,8.));
#30793=CARTESIAN_POINT('Ctrl Pts',(32.7562017414451,31.719645109407,8.));
#30794=CARTESIAN_POINT('Ctrl Pts',(32.6680097346461,31.7941428733673,8.));
#30795=CARTESIAN_POINT('Ctrl Pts',(32.6506331562116,31.8088212584686,8.));
#30796=CARTESIAN_POINT('Ctrl Pts',(32.6333715252365,31.8236489611523,8.));
#30797=CARTESIAN_POINT('Ctrl Pts',(32.6162270200198,31.8386244719266,8.));
#30798=CARTESIAN_POINT('Ctrl Pts',(32.6036927426372,31.8495730063766,8.));
#30799=CARTESIAN_POINT('Ctrl Pts',(32.5912222824502,31.8605995500244,8.));
#30800=CARTESIAN_POINT('Ctrl Pts',(32.5788252877513,31.8716953917,8.));
#30801=CARTESIAN_POINT('Ctrl Pts',(32.4862461171128,31.9545577179984,8.));
#30802=CARTESIAN_POINT('Ctrl Pts',(32.397622799937,32.0414017436923,8.));
#30803=CARTESIAN_POINT('Ctrl Pts',(32.3132167630922,32.1319065542212,8.));
#30804=CARTESIAN_POINT('Ctrl Pts',(32.2290025191065,32.2222057138629,8.));
#30805=CARTESIAN_POINT('Ctrl Pts',(32.1489858942929,32.3161497454154,8.));
#30806=CARTESIAN_POINT('Ctrl Pts',(32.0734669664008,32.4134519537301,8.));
#30807=CARTESIAN_POINT('Ctrl Pts',(31.9989803737659,32.5094240517922,8.));
#30808=CARTESIAN_POINT('Ctrl Pts',(31.9288689532965,32.6086638275202,8.));
#30809=CARTESIAN_POINT('Ctrl Pts',(31.8634666824091,32.7109170108275,8.));
#30810=CARTESIAN_POINT('Ctrl Pts',(31.8101613092083,32.7942572989124,8.));
#30811=CARTESIAN_POINT('Ctrl Pts',(31.7599848998086,32.8795998826136,8.));
#30812=CARTESIAN_POINT('Ctrl Pts',(31.7131442187192,32.9668129344489,8.));
#30813=CARTESIAN_POINT('Ctrl Pts',(31.7012430571606,32.9889718056646,8.));
#30814=CARTESIAN_POINT('Ctrl Pts',(31.6895573606131,33.0112514414787,8.));
#30815=CARTESIAN_POINT('Ctrl Pts',(31.6780907836173,33.033649704911,8.));
#30816=CARTESIAN_POINT('Ctrl Pts',(31.6699353210994,33.0495801955843,8.));
#30817=CARTESIAN_POINT('Ctrl Pts',(31.6618944152098,33.0655635106099,8.));
#30818=CARTESIAN_POINT('Ctrl Pts',(31.6539717264445,33.0815932364824,8.));
#30819=CARTESIAN_POINT('Ctrl Pts',(31.6010109140258,33.1887471750268,8.));
#30820=CARTESIAN_POINT('Ctrl Pts',(31.5532889518817,33.2980509944504,8.));
#30821=CARTESIAN_POINT('Ctrl Pts',(31.5110846398564,33.4092420858783,8.));
#30822=CARTESIAN_POINT('Ctrl Pts',(31.469716484976,33.5182302453998,8.));
#30823=CARTESIAN_POINT('Ctrl Pts',(31.4336492415757,33.6290322689246,8.));
#30824=CARTESIAN_POINT('Ctrl Pts',(31.4031936775095,33.7414146337669,8.));
#30825=CARTESIAN_POINT('Ctrl Pts',(31.39873956261,33.7578505127609,8.));
#30826=CARTESIAN_POINT('Ctrl Pts',(31.3944055654848,33.7743202085893,8.));
#30827=CARTESIAN_POINT('Ctrl Pts',(31.3901927523269,33.7908230038594,8.));
#30828=CARTESIAN_POINT('Ctrl Pts',(31.3605242058421,33.9070431945601,8.));
#30829=CARTESIAN_POINT('Ctrl Pts',(31.3368616451868,34.0249053317963,8.));
#30830=CARTESIAN_POINT('Ctrl Pts',(31.3191142145135,34.1439735700009,8.));
#30831=CARTESIAN_POINT('Ctrl Pts',(31.3091306818643,34.210953498841,8.));
#30832=CARTESIAN_POINT('Ctrl Pts',(31.3010199124296,34.2783150418024,8.));
#30833=CARTESIAN_POINT('Ctrl Pts',(31.294772781286,34.3459791587903,8.));
#30834=CARTESIAN_POINT('Ctrl Pts',(31.2918903120279,34.3771998475526,8.));
#30835=CARTESIAN_POINT('Ctrl Pts',(31.2894046732663,34.4084849312592,8.));
#30836=CARTESIAN_POINT('Ctrl Pts',(31.2873153161224,34.4398265107474,8.));
#30837=CARTESIAN_POINT('Ctrl Pts',(31.2861142259533,34.4578435659536,8.));
#30838=CARTESIAN_POINT('Ctrl Pts',(31.2850446073883,34.4758722375043,8.));
#30839=CARTESIAN_POINT('Ctrl Pts',(31.2841063911591,34.4939026846615,8.));
#30840=CARTESIAN_POINT('Ctrl Pts',(31.2777954835053,34.6151844142158,8.));
#30841=CARTESIAN_POINT('Ctrl Pts',(31.2774171066952,34.7366634572185,8.));
#30842=CARTESIAN_POINT('Ctrl Pts',(31.2828130518753,34.8578925565699,8.));
#30843=CARTESIAN_POINT('Ctrl Pts',(31.2880970630825,34.976606868563,8.));
#30844=CARTESIAN_POINT('Ctrl Pts',(31.2989188151177,35.0950824227959,8.));
#30845=CARTESIAN_POINT('Ctrl Pts',(31.3151831142098,35.2128932340069,8.));
#30846=CARTESIAN_POINT('Ctrl Pts',(31.3312885029229,35.3295529743629,8.));
#30847=CARTESIAN_POINT('Ctrl Pts',(31.3527309554357,35.4455617346014,8.));
#30848=CARTESIAN_POINT('Ctrl Pts',(31.3794648241005,35.5604869939325,8.));
#30849=CARTESIAN_POINT('Ctrl Pts',(31.3968717446295,35.6353169738744,8.));
#30850=CARTESIAN_POINT('Ctrl Pts',(31.4165229267736,35.7096871840419,8.));
#30851=CARTESIAN_POINT('Ctrl Pts',(31.438415570696,35.7834713262069,8.));
#30852=CARTESIAN_POINT('Ctrl Pts',(31.4458039136858,35.8083720440668,8.));
#30853=CARTESIAN_POINT('Ctrl Pts',(31.4534476062533,35.833205958311,8.));
#30854=CARTESIAN_POINT('Ctrl Pts',(31.4613467284242,35.8579680375739,8.));
#30855=CARTESIAN_POINT('Ctrl Pts',(31.4664331210497,35.8739128039203,8.));
#30856=CARTESIAN_POINT('Ctrl Pts',(31.4716246314855,35.8898251737367,8.));
#30857=CARTESIAN_POINT('Ctrl Pts',(31.4769184005249,35.9056957806736,8.));
#30858=CARTESIAN_POINT('Ctrl Pts',(31.5138160950465,36.0163142837243,8.));
#30859=CARTESIAN_POINT('Ctrl Pts',(31.5557145002446,36.1250213095504,8.));
#30860=CARTESIAN_POINT('Ctrl Pts',(31.6025488222259,36.2313976553429,8.));
#30861=CARTESIAN_POINT('Ctrl Pts',(31.6406629285514,36.3179674866662,8.));
#30862=CARTESIAN_POINT('Ctrl Pts',(31.6820469422375,36.4029935647969,8.));
#30863=CARTESIAN_POINT('Ctrl Pts',(31.7266869246432,36.4862342957322,8.));
#30864=CARTESIAN_POINT('Ctrl Pts',(31.7483019214948,36.5265400494563,8.));
#30865=CARTESIAN_POINT('Ctrl Pts',(31.7706805722115,36.5664269742985,8.));
#30866=CARTESIAN_POINT('Ctrl Pts',(31.7938227675543,36.605866117211,8.));
#30867=CARTESIAN_POINT('Ctrl Pts',(31.8074092117442,36.6290202608064,8.));
#30868=CARTESIAN_POINT('Ctrl Pts',(31.8212608890592,36.6520231340321,8.));
#30869=CARTESIAN_POINT('Ctrl Pts',(31.8353637243995,36.6748463853764,8.));
#30870=CARTESIAN_POINT('Ctrl Pts',(31.8937951632988,36.7694086052589,8.));
#30871=CARTESIAN_POINT('Ctrl Pts',(31.9565778581775,36.8609656088156,8.));
#30872=CARTESIAN_POINT('Ctrl Pts',(32.0236777625255,36.9491266811452,8.));
#30873=CARTESIAN_POINT('Ctrl Pts',(32.0837085788304,37.0279998358789,8.));
#30874=CARTESIAN_POINT('Ctrl Pts',(32.1471954960693,37.1041548514456,8.));
#30875=CARTESIAN_POINT('Ctrl Pts',(32.2141376235347,37.177285414151,8.));
#30876=CARTESIAN_POINT('Ctrl Pts',(32.248992559173,37.2153624988329,8.));
#30877=CARTESIAN_POINT('Ctrl Pts',(32.2847845972398,37.2526191672925,8.));
#30878=CARTESIAN_POINT('Ctrl Pts',(32.321476328717,37.2890400220485,8.));
#30879=CARTESIAN_POINT('Origin',(0.,0.,8.));
#30880=CARTESIAN_POINT('',(-50.,50.,8.));
#30881=CARTESIAN_POINT('',(-50.,-50.,8.));
#30882=CARTESIAN_POINT('',(-50.,50.,8.));
#30883=CARTESIAN_POINT('',(50.,-50.,8.));
#30884=CARTESIAN_POINT('',(-50.,-50.,8.));
#30885=CARTESIAN_POINT('',(50.,50.,8.));
#30886=CARTESIAN_POINT('',(50.,-50.,8.));
#30887=CARTESIAN_POINT('',(50.,50.,8.));
#30888=CARTESIAN_POINT('Ctrl Pts',(37.6735319337713,-32.7141668369925,8.));
#30889=CARTESIAN_POINT('Ctrl Pts',(37.7506744257016,-32.7912795331857,8.));
#30890=CARTESIAN_POINT('Ctrl Pts',(37.8237045554225,-32.8720144016735,8.));
#30891=CARTESIAN_POINT('Ctrl Pts',(37.8926300182219,-32.9559529391151,8.));
#30892=CARTESIAN_POINT('Ctrl Pts',(37.9633153902931,-33.0420347223805,8.));
#30893=CARTESIAN_POINT('Ctrl Pts',(38.0296841818896,-33.1314863178634,8.));
#30894=CARTESIAN_POINT('Ctrl Pts',(38.0917148195566,-33.2239024768849,8.));
#30895=CARTESIAN_POINT('Ctrl Pts',(38.1550365108844,-33.3182421083212,8.));
#30896=CARTESIAN_POINT('Ctrl Pts',(38.2138380035849,-33.4156715766502,8.));
#30897=CARTESIAN_POINT('Ctrl Pts',(38.268059557232,-33.515799249106,8.));
#30898=CARTESIAN_POINT('Ctrl Pts',(38.3198487844224,-33.6114352910132,8.));
#30899=CARTESIAN_POINT('Ctrl Pts',(38.3674597504585,-33.7095337219438,8.));
#30900=CARTESIAN_POINT('Ctrl Pts',(38.410804885236,-33.8097778917925,8.));
#30901=CARTESIAN_POINT('Ctrl Pts',(38.4178421610283,-33.8260529794907,8.));
#30902=CARTESIAN_POINT('Ctrl Pts',(38.4247669147912,-33.8423846664997,8.));
#30903=CARTESIAN_POINT('Ctrl Pts',(38.4315786781863,-33.8587716403974,8.));
#30904=CARTESIAN_POINT('Ctrl Pts',(38.4380889335058,-33.8744332800934,8.));
#30905=CARTESIAN_POINT('Ctrl Pts',(38.4444929624372,-33.8901382301107,8.));
#30906=CARTESIAN_POINT('Ctrl Pts',(38.4507885504088,-33.9058798359799,8.));
#30907=CARTESIAN_POINT('Ctrl Pts',(38.4941738374283,-34.014361218793,8.));
#30908=CARTESIAN_POINT('Ctrl Pts',(38.5324452713943,-34.124659589853,8.));
#30909=CARTESIAN_POINT('Ctrl Pts',(38.5655742382515,-34.2363431431182,8.));
#30910=CARTESIAN_POINT('Ctrl Pts',(38.5991377517882,-34.3494916293961,8.));
#30911=CARTESIAN_POINT('Ctrl Pts',(38.6274234029538,-34.4640626260336,8.));
#30912=CARTESIAN_POINT('Ctrl Pts',(38.6503587972893,-34.5796396359417,8.));
#30913=CARTESIAN_POINT('Ctrl Pts',(38.6743337296149,-34.7004551296896,8.));
#30914=CARTESIAN_POINT('Ctrl Pts',(38.692463198861,-34.8223707151795,8.));
#30915=CARTESIAN_POINT('Ctrl Pts',(38.7046087858744,-34.9449340325394,8.));
#30916=CARTESIAN_POINT('Ctrl Pts',(38.7137179761345,-35.0368565205594,8.));
#30917=CARTESIAN_POINT('Ctrl Pts',(38.7194601094409,-35.1291439544571,8.));
#30918=CARTESIAN_POINT('Ctrl Pts',(38.721753661108,-35.2216089483748,8.));
#30919=CARTESIAN_POINT('Ctrl Pts',(38.7223012285573,-35.2436842395473,8.));
#30920=CARTESIAN_POINT('Ctrl Pts',(38.7226520798176,-35.2657741780712,8.));
#30921=CARTESIAN_POINT('Ctrl Pts',(38.7228050031224,-35.2878471504668,8.));
#30922=CARTESIAN_POINT('Ctrl Pts',(38.723639797835,-35.4083415425535,8.));
#30923=CARTESIAN_POINT('Ctrl Pts',(38.7185864406144,-35.528481112922,8.));
#30924=CARTESIAN_POINT('Ctrl Pts',(38.7075759731584,-35.6478398239672,8.));
#30925=CARTESIAN_POINT('Ctrl Pts',(38.6966361565965,-35.766432645673,8.));
#30926=CARTESIAN_POINT('Ctrl Pts',(38.6798156826268,-35.8842554734363,8.));
#30927=CARTESIAN_POINT('Ctrl Pts',(38.6569974768235,-36.0009032638125,8.));
#30928=CARTESIAN_POINT('Ctrl Pts',(38.6541238330716,-36.0155934720123,8.));
#30929=CARTESIAN_POINT('Ctrl Pts',(38.6511549977698,-36.0302650508608,8.));
#30930=CARTESIAN_POINT('Ctrl Pts',(38.6480906778903,-36.0449171950576,8.));
#30931=CARTESIAN_POINT('Ctrl Pts',(38.6241801879288,-36.1592459728997,8.));
#30932=CARTESIAN_POINT('Ctrl Pts',(38.5944604969197,-36.2723920187216,8.));
#30933=CARTESIAN_POINT('Ctrl Pts',(38.5592377490131,-36.3840888412668,8.));
#30934=CARTESIAN_POINT('Ctrl Pts',(38.5372725083531,-36.4537440423509,8.));
#30935=CARTESIAN_POINT('Ctrl Pts',(38.5131661119788,-36.5228355678477,8.));
#30936=CARTESIAN_POINT('Ctrl Pts',(38.4869829521143,-36.5912966040202,8.));
#30937=CARTESIAN_POINT('Ctrl Pts',(38.4780335436947,-36.614696597631,8.));
#30938=CARTESIAN_POINT('Ctrl Pts',(38.4688414510417,-36.6380229129432,8.));
#30939=CARTESIAN_POINT('Ctrl Pts',(38.4594090583389,-36.6612728133014,8.));
#30940=CARTESIAN_POINT('Ctrl Pts',(38.4526597990907,-36.677909059263,8.));
#30941=CARTESIAN_POINT('Ctrl Pts',(38.4457869585498,-36.6945073015523,8.));
#30942=CARTESIAN_POINT('Ctrl Pts',(38.4387984803451,-36.7110502346119,8.));
#30943=CARTESIAN_POINT('Ctrl Pts',(38.3928771569434,-36.8197539261443,8.));
#30944=CARTESIAN_POINT('Ctrl Pts',(38.3419028069428,-36.9262312105814,8.));
#30945=CARTESIAN_POINT('Ctrl Pts',(38.286233868877,-37.0302277419135,8.));
#30946=CARTESIAN_POINT('Ctrl Pts',(38.2286497374683,-37.1378020936858,8.));
#30947=CARTESIAN_POINT('Ctrl Pts',(38.1660422723199,-37.2427227531059,8.));
#30948=CARTESIAN_POINT('Ctrl Pts',(38.0987528117336,-37.3447008755076,8.));
#30949=CARTESIAN_POINT('Ctrl Pts',(38.0308301924039,-37.447638558876,8.));
#30950=CARTESIAN_POINT('Ctrl Pts',(37.9581366181552,-37.5475788135467,8.));
#30951=CARTESIAN_POINT('Ctrl Pts',(37.8809726402855,-37.6442062900679,8.));
#30952=CARTESIAN_POINT('Ctrl Pts',(37.8265596140724,-37.7123442160536,8.));
#30953=CARTESIAN_POINT('Ctrl Pts',(37.7699226008246,-37.7788344950898,8.));
#30954=CARTESIAN_POINT('Ctrl Pts',(37.7111539331996,-37.8435580680838,8.));
#30955=CARTESIAN_POINT('Ctrl Pts',(37.6849210722466,-37.8724490496109,8.));
#30956=CARTESIAN_POINT('Ctrl Pts',(37.6582633448569,-37.9009879055023,8.));
#30957=CARTESIAN_POINT('Ctrl Pts',(37.6311883528209,-37.9291634733987,8.));
#30958=CARTESIAN_POINT('Ctrl Pts',(37.6195660136439,-37.9412582509764,8.));
#30959=CARTESIAN_POINT('Ctrl Pts',(37.6078682053827,-37.9532845462101,8.));
#30960=CARTESIAN_POINT('Ctrl Pts',(37.5961020337617,-37.9652350938879,8.));
#30961=CARTESIAN_POINT('Ctrl Pts',(37.507659771091,-38.055063247923,8.));
#30962=CARTESIAN_POINT('Ctrl Pts',(37.415258178228,-38.1407187695167,8.));
#30963=CARTESIAN_POINT('Ctrl Pts',(37.3192259922681,-38.2218835091588,8.));
#30964=CARTESIAN_POINT('Ctrl Pts',(37.2371862486548,-38.2912220789739,8.));
#30965=CARTESIAN_POINT('Ctrl Pts',(37.152495821289,-38.3572831262055,8.));
#30966=CARTESIAN_POINT('Ctrl Pts',(37.0653354498859,-38.4198507239943,8.));
#30967=CARTESIAN_POINT('Ctrl Pts',(37.0262246732672,-38.4479261819266,8.));
#30968=CARTESIAN_POINT('Ctrl Pts',(36.9866162962358,-38.4752979774627,8.));
#30969=CARTESIAN_POINT('Ctrl Pts',(36.9465254062051,-38.5019452444609,8.));
#30970=CARTESIAN_POINT('Ctrl Pts',(36.9192921690604,-38.5200463976374,8.));
#30971=CARTESIAN_POINT('Ctrl Pts',(36.8918306415648,-38.5378166037371,8.));
#30972=CARTESIAN_POINT('Ctrl Pts',(36.8641755127457,-38.555230549143,8.));
#30973=CARTESIAN_POINT('Ctrl Pts',(36.7573712570443,-38.6224832996203,8.));
#30974=CARTESIAN_POINT('Ctrl Pts',(36.6476202687202,-38.6844692470865,8.));
#30975=CARTESIAN_POINT('Ctrl Pts',(36.5352245224892,-38.7408547353335,8.));
#30976=CARTESIAN_POINT('Ctrl Pts',(36.4331307539574,-38.7920720382892,8.));
#30977=CARTESIAN_POINT('Ctrl Pts',(36.3288540451722,-38.8386685245707,8.));
#30978=CARTESIAN_POINT('Ctrl Pts',(36.2225973607791,-38.8803650263204,8.));
#30979=CARTESIAN_POINT('Ctrl Pts',(36.1671668634624,-38.9021166727374,8.));
#30980=CARTESIAN_POINT('Ctrl Pts',(36.1111972101676,-38.9225343520043,8.));
#30981=CARTESIAN_POINT('Ctrl Pts',(36.054732523776,-38.9416301760088,8.));
#30982=CARTESIAN_POINT('Ctrl Pts',(33.9479286229388,-38.9352951690526,8.));
#30983=CARTESIAN_POINT('Ctrl Pts',(33.8318204065611,-38.8956804683211,8.));
#30984=CARTESIAN_POINT('Ctrl Pts',(33.7179772526967,-38.8505153756638,8.));
#30985=CARTESIAN_POINT('Ctrl Pts',(33.6066250571068,-38.8001574942087,8.));
#30986=CARTESIAN_POINT('Ctrl Pts',(33.4927757454994,-38.7486703178014,8.));
#30987=CARTESIAN_POINT('Ctrl Pts',(33.3815297429693,-38.6917543422691,8.));
#30988=CARTESIAN_POINT('Ctrl Pts',(33.2731527586738,-38.6297431972011,8.));
#30989=CARTESIAN_POINT('Ctrl Pts',(33.1592144063828,-38.5645499484809,8.));
#30990=CARTESIAN_POINT('Ctrl Pts',(33.0484461029789,-38.4937247712042,8.));
#30991=CARTESIAN_POINT('Ctrl Pts',(32.9411957572322,-38.4176091405434,8.));
#30992=CARTESIAN_POINT('Ctrl Pts',(32.8473517047039,-38.3510079637152,8.));
#30993=CARTESIAN_POINT('Ctrl Pts',(32.7562013929947,-38.2803552258207,8.));
#30994=CARTESIAN_POINT('Ctrl Pts',(32.668009391503,-38.2058575466902,8.));
#30995=CARTESIAN_POINT('Ctrl Pts',(32.6506323829748,-38.1911788141103,8.));
#30996=CARTESIAN_POINT('Ctrl Pts',(32.6333703275703,-38.1763507567444,8.));
#30997=CARTESIAN_POINT('Ctrl Pts',(32.6162254037543,-38.1613748841763,8.));
#30998=CARTESIAN_POINT('Ctrl Pts',(32.603691142847,-38.1504263669302,8.));
#30999=CARTESIAN_POINT('Ctrl Pts',(32.5912206997708,-38.139399841404,8.));
#31000=CARTESIAN_POINT('Ctrl Pts',(32.5788237219142,-38.1283040179759,8.));
#31001=CARTESIAN_POINT('Ctrl Pts',(32.4862445714949,-38.0454417334689,8.));
#31002=CARTESIAN_POINT('Ctrl Pts',(32.3976212761744,-37.9585977539474,8.));
#31003=CARTESIAN_POINT('Ctrl Pts',(32.3132152636303,-37.8680929905958,8.));
#31004=CARTESIAN_POINT('Ctrl Pts',(32.2290010683149,-37.7777939042141,8.));
#31005=CARTESIAN_POINT('Ctrl Pts',(32.1489844921721,-37.6838499490402,8.));
#31006=CARTESIAN_POINT('Ctrl Pts',(32.0734656135458,-37.5865478166696,8.));
#31007=CARTESIAN_POINT('Ctrl Pts',(31.9989790801238,-37.4905758071975,8.));
#31008=CARTESIAN_POINT('Ctrl Pts',(31.9288677181994,-37.3913361205739,8.));
#31009=CARTESIAN_POINT('Ctrl Pts',(31.8634655056288,-37.2890830233624,8.));
#31010=CARTESIAN_POINT('Ctrl Pts',(31.8101602412414,-37.2057429012617,8.));
#31011=CARTESIAN_POINT('Ctrl Pts',(31.7599839333137,-37.1204004861509,8.));
#31012=CARTESIAN_POINT('Ctrl Pts',(31.7131433458597,-37.0331876031136,8.));
#31013=CARTESIAN_POINT('Ctrl Pts',(31.7012416847729,-37.011027800414,8.));
#31014=CARTESIAN_POINT('Ctrl Pts',(31.6895555071392,-36.9887472225083,8.));
#31015=CARTESIAN_POINT('Ctrl Pts',(31.6780884679743,-36.9663480066189,8.));
#31016=CARTESIAN_POINT('Ctrl Pts',(31.6699335871488,-36.9504186168665,8.));
#31017=CARTESIAN_POINT('Ctrl Pts',(31.6618932487394,-36.9344364128785,8.));
#31018=CARTESIAN_POINT('Ctrl Pts',(31.6539711105215,-36.918407803011,8.));
#31019=CARTESIAN_POINT('Ctrl Pts',(31.6010103294039,-36.8112539418358,8.));
#31020=CARTESIAN_POINT('Ctrl Pts',(31.553288398372,-36.7019501913722,8.));
#31021=CARTESIAN_POINT('Ctrl Pts',(31.5110841176717,-36.5907591572156,8.));
#31022=CARTESIAN_POINT('Ctrl Pts',(31.4697159940302,-36.4817710552385,8.));
#31023=CARTESIAN_POINT('Ctrl Pts',(31.433648781936,-36.3709690780795,8.));
#31024=CARTESIAN_POINT('Ctrl Pts',(31.4031932495943,-36.2585867452464,8.));
#31025=CARTESIAN_POINT('Ctrl Pts',(31.3987391935523,-36.2421510709998,8.));
#31026=CARTESIAN_POINT('Ctrl Pts',(31.3944052523692,-36.2256815804349,8.));
#31027=CARTESIAN_POINT('Ctrl Pts',(31.3901924922002,-36.2091789909079,8.));
#31028=CARTESIAN_POINT('Ctrl Pts',(31.3605239499998,-36.0929588041061,8.));
#31029=CARTESIAN_POINT('Ctrl Pts',(31.3368613966103,-35.9750966537399,8.));
#31030=CARTESIAN_POINT('Ctrl Pts',(31.319113975657,-35.8560283881328,8.));
#31031=CARTESIAN_POINT('Ctrl Pts',(31.3091304483948,-35.7890484433355,8.));
#31032=CARTESIAN_POINT('Ctrl Pts',(31.3010196851544,-35.7216868798927,8.));
#31033=CARTESIAN_POINT('Ctrl Pts',(31.2947725609189,-35.6540227383851,8.));
#31034=CARTESIAN_POINT('Ctrl Pts',(31.2918900964785,-35.6228020559662,8.));
#31035=CARTESIAN_POINT('Ctrl Pts',(31.2894044622378,-35.591516977816,8.));
#31036=CARTESIAN_POINT('Ctrl Pts',(31.2873151093096,-35.5601754031315,8.));
#31037=CARTESIAN_POINT('Ctrl Pts',(31.2861140199798,-35.542158326923,8.));
#31038=CARTESIAN_POINT('Ctrl Pts',(31.2850444024964,-35.5241296340464,8.));
#31039=CARTESIAN_POINT('Ctrl Pts',(31.2841061875917,-35.5060991653233,8.));
#31040=CARTESIAN_POINT('Ctrl Pts',(31.2777952935748,-35.3848173815625,8.));
#31041=CARTESIAN_POINT('Ctrl Pts',(31.2774169324427,-35.2633382728991,8.));
#31042=CARTESIAN_POINT('Ctrl Pts',(31.2828128947659,-35.142109099441,8.));
#31043=CARTESIAN_POINT('Ctrl Pts',(31.2880969228261,-35.0233947134034,8.));
#31044=CARTESIAN_POINT('Ctrl Pts',(31.2989186932579,-34.9049190770275,8.));
#31045=CARTESIAN_POINT('Ctrl Pts',(31.3151830117592,-34.7871081783408,8.));
#31046=CARTESIAN_POINT('Ctrl Pts',(31.3312884180702,-34.67044836311,8.));
#31047=CARTESIAN_POINT('Ctrl Pts',(31.3527308881008,-34.5544395226326,8.));
#31048=CARTESIAN_POINT('Ctrl Pts',(31.3794647737014,-34.4395141802506,8.));
#31049=CARTESIAN_POINT('Ctrl Pts',(31.396871707047,-34.3646841385402,8.));
#31050=CARTESIAN_POINT('Ctrl Pts',(31.416522902222,-34.2903138655065,8.));
#31051=CARTESIAN_POINT('Ctrl Pts',(31.4384155592443,-34.2165296601315,8.));
#31052=CARTESIAN_POINT('Ctrl Pts',(31.4458038981696,-34.1916289495378,8.));
#31053=CARTESIAN_POINT('Ctrl Pts',(31.4534475860939,-34.1667950423673,8.));
#31054=CARTESIAN_POINT('Ctrl Pts',(31.461346703037,-34.1420329699976,8.));
#31055=CARTESIAN_POINT('Ctrl Pts',(31.46643308557,-34.1260882291753,8.));
#31056=CARTESIAN_POINT('Ctrl Pts',(31.471624585416,-34.1101758846519,8.));
#31057=CARTESIAN_POINT('Ctrl Pts',(31.476918343353,-34.0943053028287,8.));
#31058=CARTESIAN_POINT('Ctrl Pts',(31.513816049212,-33.9836867088362,8.));
#31059=CARTESIAN_POINT('Ctrl Pts',(31.5557144650388,-33.8749795921173,8.));
#31060=CARTESIAN_POINT('Ctrl Pts',(31.6025487964097,-33.7686031580514,8.));
#31061=CARTESIAN_POINT('Ctrl Pts',(31.6406629208299,-33.6820332311479,8.));
#31062=CARTESIAN_POINT('Ctrl Pts',(31.682046953583,-33.5970070600165,8.));
#31063=CARTESIAN_POINT('Ctrl Pts',(31.7266869557237,-33.5137662402706,8.));
#31064=CARTESIAN_POINT('Ctrl Pts',(31.7483019580961,-33.4734604510681,8.));
#31065=CARTESIAN_POINT('Ctrl Pts',(31.7706806142055,-33.4335734915742,8.));
#31066=CARTESIAN_POINT('Ctrl Pts',(31.7938228147784,-33.3941343150086,8.));
#31067=CARTESIAN_POINT('Ctrl Pts',(31.8074092885987,-33.3709801063925,8.));
#31068=CARTESIAN_POINT('Ctrl Pts',(31.8212609965416,-33.347977169053,8.));
#31069=CARTESIAN_POINT('Ctrl Pts',(31.8353638634359,-33.3251538546887,8.));
#31070=CARTESIAN_POINT('Ctrl Pts',(31.8937952976074,-33.2305915929272,8.));
#31071=CARTESIAN_POINT('Ctrl Pts',(31.9565779834776,-33.1390345522359,8.));
#31072=CARTESIAN_POINT('Ctrl Pts',(32.0236778740976,-33.0508734495428,8.));
#31073=CARTESIAN_POINT('Ctrl Pts',(32.0837087245751,-32.972000206609,8.));
#31074=CARTESIAN_POINT('Ctrl Pts',(32.1471956775548,-32.8958451124639,8.));
#31075=CARTESIAN_POINT('Ctrl Pts',(32.2141378419758,-32.8227144830143,8.));
#31076=CARTESIAN_POINT('Ctrl Pts',(32.2489927811285,-32.7846373807617,8.));
#31077=CARTESIAN_POINT('Ctrl Pts',(32.2847848221939,-32.7473806972021,8.));
#31078=CARTESIAN_POINT('Ctrl Pts',(32.3214765561793,-32.7109598296518,8.));
#31079=CARTESIAN_POINT('Ctrl Pts',(-32.3264680662287,-32.7141668369925,
8.));
#31080=CARTESIAN_POINT('Ctrl Pts',(-32.2493255072635,-32.7912796001948,
8.));
#31081=CARTESIAN_POINT('Ctrl Pts',(-32.1762953075955,-32.8720145313034,
8.));
#31082=CARTESIAN_POINT('Ctrl Pts',(-32.1073697738656,-32.9559531279149,
8.));
#31083=CARTESIAN_POINT('Ctrl Pts',(-32.0366843378685,-33.0420349611253,
8.));
#31084=CARTESIAN_POINT('Ctrl Pts',(-31.9703154802321,-33.1314866020839,
8.));
#31085=CARTESIAN_POINT('Ctrl Pts',(-31.9082847764611,-33.2239028032894,
8.));
#31086=CARTESIAN_POINT('Ctrl Pts',(-31.8449630319238,-33.3182424565268,
8.));
#31087=CARTESIAN_POINT('Ctrl Pts',(-31.786161483907,-33.415671941835,8.));
#31088=CARTESIAN_POINT('Ctrl Pts',(-31.7319398749946,-33.5157996279616,
8.));
#31089=CARTESIAN_POINT('Ctrl Pts',(-31.6801506359753,-33.6114356072929,
8.));
#31090=CARTESIAN_POINT('Ctrl Pts',(-31.6325396515499,-33.709533968736,8.));
#31091=CARTESIAN_POINT('Ctrl Pts',(-31.5891944935205,-33.8097780642334,
8.));
#31092=CARTESIAN_POINT('Ctrl Pts',(-31.582156905406,-33.8260538534356,8.));
#31093=CARTESIAN_POINT('Ctrl Pts',(-31.5752318490596,-33.8423862467834,
8.));
#31094=CARTESIAN_POINT('Ctrl Pts',(-31.568419792889,-33.8587739316911,8.));
#31095=CARTESIAN_POINT('Ctrl Pts',(-31.5619098742369,-33.8744347678579,
8.));
#31096=CARTESIAN_POINT('Ctrl Pts',(-31.5555061718916,-33.8901389077819,
8.));
#31097=CARTESIAN_POINT('Ctrl Pts',(-31.5492108990198,-33.9058797005882,
8.));
#31098=CARTESIAN_POINT('Ctrl Pts',(-31.5058255436634,-34.0143610807278,
8.));
#31099=CARTESIAN_POINT('Ctrl Pts',(-31.4675540442795,-34.1246594478804,
8.));
#31100=CARTESIAN_POINT('Ctrl Pts',(-31.434425017105,-34.2363429975606,8.));
#31101=CARTESIAN_POINT('Ctrl Pts',(-31.4008614525105,-34.3494914463237,
8.));
#31102=CARTESIAN_POINT('Ctrl Pts',(-31.3725757523594,-34.4640624049253,
8.));
#31103=CARTESIAN_POINT('Ctrl Pts',(-31.3496403133382,-34.5796393782454,
8.));
#31104=CARTESIAN_POINT('Ctrl Pts',(-31.3256653487767,-34.7004547608028,
8.));
#31105=CARTESIAN_POINT('Ctrl Pts',(-31.307535844936,-34.8223702353544,8.));
#31106=CARTESIAN_POINT('Ctrl Pts',(-31.2953902232888,-34.9449334450722,
8.));
#31107=CARTESIAN_POINT('Ctrl Pts',(-31.2862810070535,-35.0368558523606,
8.));
#31108=CARTESIAN_POINT('Ctrl Pts',(-31.2805388477475,-35.1291432073786,
8.));
#31109=CARTESIAN_POINT('Ctrl Pts',(-31.2782452710195,-35.2216081255571,
8.));
#31110=CARTESIAN_POINT('Ctrl Pts',(-31.2776977000309,-35.243683300125,8.));
#31111=CARTESIAN_POINT('Ctrl Pts',(-31.2773468435284,-35.2657731220308,
8.));
#31112=CARTESIAN_POINT('Ctrl Pts',(-31.277193913283,-35.2878459781507,8.));
#31113=CARTESIAN_POINT('Ctrl Pts',(-31.2763590765867,-35.4083403266138,
8.));
#31114=CARTESIAN_POINT('Ctrl Pts',(-31.2814123990406,-35.5284798599375,
8.));
#31115=CARTESIAN_POINT('Ctrl Pts',(-31.2924228410947,-35.6478385426709,
8.));
#31116=CARTESIAN_POINT('Ctrl Pts',(-31.303362629127,-35.7664313005734,8.));
#31117=CARTESIAN_POINT('Ctrl Pts',(-31.3201830802735,-35.8842540736147,
8.));
#31118=CARTESIAN_POINT('Ctrl Pts',(-31.3430012709811,-36.000901820846,8.));
#31119=CARTESIAN_POINT('Ctrl Pts',(-31.3458749177941,-36.0155920489787,
8.));
#31120=CARTESIAN_POINT('Ctrl Pts',(-31.3488437566082,-36.0302636478795,
8.));
#31121=CARTESIAN_POINT('Ctrl Pts',(-31.3519080804568,-36.0449158122488,
8.));
#31122=CARTESIAN_POINT('Ctrl Pts',(-31.3758185581684,-36.1592445408324,
8.));
#31123=CARTESIAN_POINT('Ctrl Pts',(-31.4055382437248,-36.2723905489836,
8.));
#31124=CARTESIAN_POINT('Ctrl Pts',(-31.4407609915798,-36.3840873440382,
8.));
#31125=CARTESIAN_POINT('Ctrl Pts',(-31.4627262403709,-36.4537425538657,
8.));
#31126=CARTESIAN_POINT('Ctrl Pts',(-31.4868326485685,-36.5228340916482,
8.));
#31127=CARTESIAN_POINT('Ctrl Pts',(-31.5130158235422,-36.5912951432516,
8.));
#31128=CARTESIAN_POINT('Ctrl Pts',(-31.5219654331702,-36.6146956547323,
8.));
#31129=CARTESIAN_POINT('Ctrl Pts',(-31.5311577380477,-36.638022485054,8.));
#31130=CARTESIAN_POINT('Ctrl Pts',(-31.5405903538195,-36.6612728973655,
8.));
#31131=CARTESIAN_POINT('Ctrl Pts',(-31.5473394036631,-36.677908600056,8.));
#31132=CARTESIAN_POINT('Ctrl Pts',(-31.5542120267349,-36.6945063014083,
8.));
#31133=CARTESIAN_POINT('Ctrl Pts',(-31.5612002800447,-36.7110486972688,
8.));
#31134=CARTESIAN_POINT('Ctrl Pts',(-31.6071216062265,-36.8197523636167,
8.));
#31135=CARTESIAN_POINT('Ctrl Pts',(-31.6580959615467,-36.9262296326556,
8.));
#31136=CARTESIAN_POINT('Ctrl Pts',(-31.7137649062032,-37.0302261570189,
8.));
#31137=CARTESIAN_POINT('Ctrl Pts',(-31.7713490613653,-37.1378005332208,
8.));
#31138=CARTESIAN_POINT('Ctrl Pts',(-31.833956554581,-37.2427212245297,8.));
#31139=CARTESIAN_POINT('Ctrl Pts',(-31.9012460458509,-37.3446993846474,
8.));
#31140=CARTESIAN_POINT('Ctrl Pts',(-31.9691687068521,-37.4476371223012,
8.));
#31141=CARTESIAN_POINT('Ctrl Pts',(-32.0418623269422,-37.547577436253,8.));
#31142=CARTESIAN_POINT('Ctrl Pts',(-32.1190263529718,-37.6442049753141,
8.));
#31143=CARTESIAN_POINT('Ctrl Pts',(-32.1734394282079,-37.7123429642625,
8.));
#31144=CARTESIAN_POINT('Ctrl Pts',(-32.230076492864,-37.7788333069719,8.));
#31145=CARTESIAN_POINT('Ctrl Pts',(-32.288845213566,-37.8435569436544,8.));
#31146=CARTESIAN_POINT('Ctrl Pts',(-32.3150777918285,-37.8724476161826,
8.));
#31147=CARTESIAN_POINT('Ctrl Pts',(-32.3417352269367,-37.9009861713024,
8.));
#31148=CARTESIAN_POINT('Ctrl Pts',(-32.3688099173017,-37.9291614469859,
8.));
#31149=CARTESIAN_POINT('Ctrl Pts',(-32.3804320487223,-37.941256017686,8.));
#31150=CARTESIAN_POINT('Ctrl Pts',(-32.3921296471323,-37.9532821092146,
8.));
#31151=CARTESIAN_POINT('Ctrl Pts',(-32.4038956063136,-37.9652324558272,
8.));
#31152=CARTESIAN_POINT('Ctrl Pts',(-32.4923378704609,-38.0550607218847,
8.));
#31153=CARTESIAN_POINT('Ctrl Pts',(-32.5847394664431,-38.1407163588179,
8.));
#31154=CARTESIAN_POINT('Ctrl Pts',(-32.6807716550536,-38.2218812155311,
8.));
#31155=CARTESIAN_POINT('Ctrl Pts',(-32.7628115828128,-38.2912200390828,
8.));
#31156=CARTESIAN_POINT('Ctrl Pts',(-32.8475022057307,-38.3572813267927,
8.));
#31157=CARTESIAN_POINT('Ctrl Pts',(-32.9346627816287,-38.4198491494197,
8.));
#31158=CARTESIAN_POINT('Ctrl Pts',(-32.9737737137373,-38.447924753989,8.));
#31159=CARTESIAN_POINT('Ctrl Pts',(-33.0133822496832,-38.4752966907185,
8.));
#31160=CARTESIAN_POINT('Ctrl Pts',(-33.0534733017689,-38.5019440931387,
8.));
#31161=CARTESIAN_POINT('Ctrl Pts',(-33.0807070399686,-38.5200455981744,
8.));
#31162=CARTESIAN_POINT('Ctrl Pts',(-33.1081690766608,-38.5378161440549,
8.));
#31163=CARTESIAN_POINT('Ctrl Pts',(-33.1358247214715,-38.5552304161034,
8.));
#31164=CARTESIAN_POINT('Ctrl Pts',(-33.2426290354803,-38.6224832099845,
8.));
#31165=CARTESIAN_POINT('Ctrl Pts',(-33.3523800768607,-38.684469196206,8.));
#31166=CARTESIAN_POINT('Ctrl Pts',(-33.4647758690787,-38.7408547167133,
8.));
#31167=CARTESIAN_POINT('Ctrl Pts',(-33.5668696003918,-38.7920720093452,
8.));
#31168=CARTESIAN_POINT('Ctrl Pts',(-33.6711462627517,-38.8386684870918,
8.));
#31169=CARTESIAN_POINT('Ctrl Pts',(-33.777402890587,-38.880364981349,8.));
#31170=CARTESIAN_POINT('Ctrl Pts',(-33.8328334021929,-38.9021166410425,
8.));
#31171=CARTESIAN_POINT('Ctrl Pts',(-33.8888030678697,-38.9225343317631,
8.));
#31172=CARTESIAN_POINT('Ctrl Pts',(-33.9452677648582,-38.941630165528,8.));
#31173=CARTESIAN_POINT('Ctrl Pts',(-36.0520713770612,-38.9352951690526,
8.));
#31174=CARTESIAN_POINT('Ctrl Pts',(-36.1681793348248,-38.8956805565571,
8.));
#31175=CARTESIAN_POINT('Ctrl Pts',(-36.2820222319885,-38.8505155239877,
8.));
#31176=CARTESIAN_POINT('Ctrl Pts',(-36.39337417598,-38.8001576820793,8.));
#31177=CARTESIAN_POINT('Ctrl Pts',(-36.507223335641,-38.7486704984873,8.));
#31178=CARTESIAN_POINT('Ctrl Pts',(-36.6184691867386,-38.6917544842536,
8.));
#31179=CARTESIAN_POINT('Ctrl Pts',(-36.726846022942,-38.6297432779853,8.));
#31180=CARTESIAN_POINT('Ctrl Pts',(-36.8407844151035,-38.5645498530274,
8.));
#31181=CARTESIAN_POINT('Ctrl Pts',(-36.9515527511922,-38.4937244553102,
8.));
#31182=CARTESIAN_POINT('Ctrl Pts',(-37.0588031240991,-38.417608572184,8.));
#31183=CARTESIAN_POINT('Ctrl Pts',(-37.1526472003926,-38.3510071744486,
8.));
#31184=CARTESIAN_POINT('Ctrl Pts',(-37.2437975316357,-38.2803541911134,
8.));
#31185=CARTESIAN_POINT('Ctrl Pts',(-37.3319895495211,-38.2058562501456,
8.));
#31186=CARTESIAN_POINT('Ctrl Pts',(-37.3493652308069,-38.1911785898568,
8.));
#31187=CARTESIAN_POINT('Ctrl Pts',(-37.3666259764485,-38.1763516270108,
8.));
#31188=CARTESIAN_POINT('Ctrl Pts',(-37.3837696084918,-38.1613768709081,
8.));
#31189=CARTESIAN_POINT('Ctrl Pts',(-37.3963039208792,-38.1504283000079,
8.));
#31190=CARTESIAN_POINT('Ctrl Pts',(-37.4087744173897,-38.1394017179875,
8.));
#31191=CARTESIAN_POINT('Ctrl Pts',(-37.421171447845,-38.1283058376695,8.));
#31192=CARTESIAN_POINT('Ctrl Pts',(-37.5137506606012,-38.0454434240953,
8.));
#31193=CARTESIAN_POINT('Ctrl Pts',(-37.6023740233075,-37.9585993019841,
8.));
#31194=CARTESIAN_POINT('Ctrl Pts',(-37.686780110783,-37.8680943929378,8.));
#31195=CARTESIAN_POINT('Ctrl Pts',(-37.7709944562299,-37.7777950803761,
8.));
#31196=CARTESIAN_POINT('Ctrl Pts',(-37.8510111825053,-37.6838508893952,
8.));
#31197=CARTESIAN_POINT('Ctrl Pts',(-37.9265302130999,-37.5865485225552,
8.));
#31198=CARTESIAN_POINT('Ctrl Pts',(-38.0010169291866,-37.4905762395914,
8.));
#31199=CARTESIAN_POINT('Ctrl Pts',(-38.0711284717142,-37.3913362778857,
8.));
#31200=CARTESIAN_POINT('Ctrl Pts',(-38.1365308641829,-37.2890829148734,
8.));
#31201=CARTESIAN_POINT('Ctrl Pts',(-38.1898364642257,-37.2057422805937,
8.));
#31202=CARTESIAN_POINT('Ctrl Pts',(-38.2400130851628,-37.1203993452656,
8.));
#31203=CARTESIAN_POINT('Ctrl Pts',(-38.2868539614533,-37.0331859413737,
8.));
#31204=CARTESIAN_POINT('Ctrl Pts',(-38.2987540819478,-37.0110290114177,
8.));
#31205=CARTESIAN_POINT('Ctrl Pts',(-38.3104387758635,-36.9887513389692,
8.));
#31206=CARTESIAN_POINT('Ctrl Pts',(-38.3219043896502,-36.9663550605045,
8.));
#31207=CARTESIAN_POINT('Ctrl Pts',(-38.3300610648434,-36.9504222746659,
8.));
#31208=CARTESIAN_POINT('Ctrl Pts',(-38.3381031537755,-36.9344366433847,
8.));
#31209=CARTESIAN_POINT('Ctrl Pts',(-38.3460269902799,-36.918404590898,8.));
#31210=CARTESIAN_POINT('Ctrl Pts',(-38.3989878678949,-36.8112504908368,
8.));
#31211=CARTESIAN_POINT('Ctrl Pts',(-38.4467098948397,-36.7019465274356,
8.));
#31212=CARTESIAN_POINT('Ctrl Pts',(-38.4889142721076,-36.5907553164102,
8.));
#31213=CARTESIAN_POINT('Ctrl Pts',(-38.5302824920512,-36.4817670367281,
8.));
#31214=CARTESIAN_POINT('Ctrl Pts',(-38.566349800654,-36.3709649163585,8.));
#31215=CARTESIAN_POINT('Ctrl Pts',(-38.5968054307926,-36.2585824846173,
8.));
#31216=CARTESIAN_POINT('Ctrl Pts',(-38.6012596681997,-36.2421461794391,
8.));
#31217=CARTESIAN_POINT('Ctrl Pts',(-38.6055937817646,-36.225676056354,8.));
#31218=CARTESIAN_POINT('Ctrl Pts',(-38.6098067052154,-36.2091728328306,
8.));
#31219=CARTESIAN_POINT('Ctrl Pts',(-38.6394752606328,-36.0929526338671,
8.));
#31220=CARTESIAN_POINT('Ctrl Pts',(-38.6631378364378,-35.9750905238851,
8.));
#31221=CARTESIAN_POINT('Ctrl Pts',(-38.6808852873793,-35.8560223427045,
8.));
#31222=CARTESIAN_POINT('Ctrl Pts',(-38.6908688312617,-35.7890424470708,
8.));
#31223=CARTESIAN_POINT('Ctrl Pts',(-38.6989796136129,-35.7216809467524,
8.));
#31224=CARTESIAN_POINT('Ctrl Pts',(-38.705226759162,-35.6540168808315,8.));
#31225=CARTESIAN_POINT('Ctrl Pts',(-38.7081092384591,-35.6227961788899,
8.));
#31226=CARTESIAN_POINT('Ctrl Pts',(-38.7105948866426,-35.5915110836458,
8.));
#31227=CARTESIAN_POINT('Ctrl Pts',(-38.7126842525742,-35.5601694941906,
8.));
#31228=CARTESIAN_POINT('Ctrl Pts',(-38.713885344499,-35.542152482698,8.));
#31229=CARTESIAN_POINT('Ctrl Pts',(-38.7149549653242,-35.5241238555354,
8.));
#31230=CARTESIAN_POINT('Ctrl Pts',(-38.7158931843189,-35.5060934532667,
8.));
#31231=CARTESIAN_POINT('Ctrl Pts',(-38.7222041204107,-35.3848118366399,
8.));
#31232=CARTESIAN_POINT('Ctrl Pts',(-38.7225825299149,-35.2633329304591,
8.));
#31233=CARTESIAN_POINT('Ctrl Pts',(-38.717186620484,-35.142103985552,8.));
#31234=CARTESIAN_POINT('Ctrl Pts',(-38.7119026444224,-35.0233898278976,
8.));
#31235=CARTESIAN_POINT('Ctrl Pts',(-38.7010809307532,-34.9049144449008,
8.));
#31236=CARTESIAN_POINT('Ctrl Pts',(-38.684816672141,-34.7871038160559,8.));
#31237=CARTESIAN_POINT('Ctrl Pts',(-38.668711320133,-34.6704442318052,8.));
#31238=CARTESIAN_POINT('Ctrl Pts',(-38.6472689041617,-34.5544356388673,
8.));
#31239=CARTESIAN_POINT('Ctrl Pts',(-38.6205350708283,-34.439510552711,8.));
#31240=CARTESIAN_POINT('Ctrl Pts',(-38.6031281770284,-34.364680701536,8.));
#31241=CARTESIAN_POINT('Ctrl Pts',(-38.5834770220596,-34.2903106224296,
8.));
#31242=CARTESIAN_POINT('Ctrl Pts',(-38.5615844054563,-34.2165266120474,
8.));
#31243=CARTESIAN_POINT('Ctrl Pts',(-38.5541960539989,-34.1916258790507,
8.));
#31244=CARTESIAN_POINT('Ctrl Pts',(-38.5465523517576,-34.1667919500715,
8.));
#31245=CARTESIAN_POINT('Ctrl Pts',(-38.5386532186941,-34.1420298564502,
8.));
#31246=CARTESIAN_POINT('Ctrl Pts',(-38.5335668050111,-34.1260850368347,
8.));
#31247=CARTESIAN_POINT('Ctrl Pts',(-38.5283752724802,-34.1101726142316,
8.));
#31248=CARTESIAN_POINT('Ctrl Pts',(-38.5230814802764,-34.094301954882,8.));
#31249=CARTESIAN_POINT('Ctrl Pts',(-38.4861838094094,-33.9836836414723,
8.));
#31250=CARTESIAN_POINT('Ctrl Pts',(-38.4442854263901,-33.8749768051962,
8.));
#31251=CARTESIAN_POINT('Ctrl Pts',(-38.3974511240065,-33.7686006435033,
8.));
#31252=CARTESIAN_POINT('Ctrl Pts',(-38.3593370554135,-33.6820310114798,
8.));
#31253=CARTESIAN_POINT('Ctrl Pts',(-38.3179530814865,-33.5970051272784,
8.));
#31254=CARTESIAN_POINT('Ctrl Pts',(-38.2733131402326,-33.5137645815446,
8.));
#31255=CARTESIAN_POINT('Ctrl Pts',(-38.2516981548861,-33.4734589017939,
8.));
#31256=CARTESIAN_POINT('Ctrl Pts',(-38.2293195154062,-33.4335720492035,
8.));
#31257=CARTESIAN_POINT('Ctrl Pts',(-38.2061773309613,-33.3941329764629,
8.));
#31258=CARTESIAN_POINT('Ctrl Pts',(-38.1925909485316,-33.3709789684133,
8.));
#31259=CARTESIAN_POINT('Ctrl Pts',(-38.1787393350554,-33.3479762288434,
8.));
#31260=CARTESIAN_POINT('Ctrl Pts',(-38.1646365654847,-33.3251531088758,
8.));
#31261=CARTESIAN_POINT('Ctrl Pts',(-38.1062051167558,-33.2305909764135,
8.));
#31262=CARTESIAN_POINT('Ctrl Pts',(-38.0434224031259,-33.139034050394,8.));
#31263=CARTESIAN_POINT('Ctrl Pts',(-37.9763224701899,-33.050873041493,8.));
#31264=CARTESIAN_POINT('Ctrl Pts',(-37.9162917251371,-32.972000070726,8.));
#31265=CARTESIAN_POINT('Ctrl Pts',(-37.8528048824192,-32.8958452190746,
8.));
#31266=CARTESIAN_POINT('Ctrl Pts',(-37.7858628320068,-32.8227147956203,
8.));
#31267=CARTESIAN_POINT('Ctrl Pts',(-37.7510079037,-32.7846377476237,8.));
#31268=CARTESIAN_POINT('Ctrl Pts',(-37.7152158718889,-32.7473811107005,
8.));
#31269=CARTESIAN_POINT('Ctrl Pts',(-37.6785241456451,-32.7109602826758,
8.));
#31270=CARTESIAN_POINT('Ctrl Pts',(-32.3264680662287,37.2858331630075,8.));
#31271=CARTESIAN_POINT('Ctrl Pts',(-32.2493254281347,37.208720320707,8.));
#31272=CARTESIAN_POINT('Ctrl Pts',(-32.1762951458997,37.1279853156793,8.));
#31273=CARTESIAN_POINT('Ctrl Pts',(-32.1073695284417,37.0440466492215,8.));
#31274=CARTESIAN_POINT('Ctrl Pts',(-32.036684016981,36.9579647570495,8.));
#31275=CARTESIAN_POINT('Ctrl Pts',(-31.9703150813857,36.8685130624034,8.));
#31276=CARTESIAN_POINT('Ctrl Pts',(-31.9082842995806,36.7760968113946,8.));
#31277=CARTESIAN_POINT('Ctrl Pts',(-31.8449624922372,36.6817571324243,8.));
#31278=CARTESIAN_POINT('Ctrl Pts',(-31.7861608789268,36.5843276270745,8.));
#31279=CARTESIAN_POINT('Ctrl Pts',(-31.7319392047808,36.4841999248104,8.));
#31280=CARTESIAN_POINT('Ctrl Pts',(-31.680149951798,36.3885640193387,8.));
#31281=CARTESIAN_POINT('Ctrl Pts',(-31.6325389456654,36.2904657399127,8.));
#31282=CARTESIAN_POINT('Ctrl Pts',(-31.5891937601898,36.1902217321721,8.));
#31283=CARTESIAN_POINT('Ctrl Pts',(-31.5821558034642,36.1739451150407,8.));
#31284=CARTESIAN_POINT('Ctrl Pts',(-31.575230390001,36.1576118880571,8.));
#31285=CARTESIAN_POINT('Ctrl Pts',(-31.56841798829,36.1412233640005,8.));
#31286=CARTESIAN_POINT('Ctrl Pts',(-31.5619084669515,36.125563476111,8.));
#31287=CARTESIAN_POINT('Ctrl Pts',(-31.5555051500235,36.1098602922108,8.));
#31288=CARTESIAN_POINT('Ctrl Pts',(-31.5492102490141,36.0941204589327,8.));
#31289=CARTESIAN_POINT('Ctrl Pts',(-31.5058248130015,35.9856390819387,8.));
#31290=CARTESIAN_POINT('Ctrl Pts',(-31.467553236408,35.8753407193868,8.));
#31291=CARTESIAN_POINT('Ctrl Pts',(-31.4344241380457,35.7636571739254,8.));
#31292=CARTESIAN_POINT('Ctrl Pts',(-31.4008605131946,35.650508769435,8.));
#31293=CARTESIAN_POINT('Ctrl Pts',(-31.3725747552338,35.5359378557202,8.));
#31294=CARTESIAN_POINT('Ctrl Pts',(-31.3496392634799,35.4203609255757,8.));
#31295=CARTESIAN_POINT('Ctrl Pts',(-31.3256642608852,35.2995456742689,8.));
#31296=CARTESIAN_POINT('Ctrl Pts',(-31.3075347162269,35.1776303306686,8.));
#31297=CARTESIAN_POINT('Ctrl Pts',(-31.2953890537165,35.0550672480091,8.));
#31298=CARTESIAN_POINT('Ctrl Pts',(-31.2862798068337,34.9631449360145,8.));
#31299=CARTESIAN_POINT('Ctrl Pts',(-31.2805376168519,34.8708576741034,8.));
#31300=CARTESIAN_POINT('Ctrl Pts',(-31.2782440105566,34.778392845323,8.));
#31301=CARTESIAN_POINT('Ctrl Pts',(-31.2776964353943,34.7563178084142,8.));
#31302=CARTESIAN_POINT('Ctrl Pts',(-31.2773455727076,34.7342281241833,8.));
#31303=CARTESIAN_POINT('Ctrl Pts',(-31.2771926342729,34.7121554053342,8.));
#31304=CARTESIAN_POINT('Ctrl Pts',(-31.2763577480363,34.5916611083402,8.));
#31305=CARTESIAN_POINT('Ctrl Pts',(-31.2814110294711,34.4715216187175,8.));
#31306=CARTESIAN_POINT('Ctrl Pts',(-31.2924214415633,34.3521629693739,8.));
#31307=CARTESIAN_POINT('Ctrl Pts',(-31.3033611959409,34.2335702867641,8.));
#31308=CARTESIAN_POINT('Ctrl Pts',(-31.3201816201703,34.115747578293,8.));
#31309=CARTESIAN_POINT('Ctrl Pts',(-31.3429997930851,33.999099881963,8.));
#31310=CARTESIAN_POINT('Ctrl Pts',(-31.345873443513,33.984409630306,8.));
#31311=CARTESIAN_POINT('Ctrl Pts',(-31.3488422864746,33.96973800774,8.));
#31312=CARTESIAN_POINT('Ctrl Pts',(-31.35190661501,33.9550858195635,8.));
#31313=CARTESIAN_POINT('Ctrl Pts',(-31.3758170782861,33.8407571491025,8.));
#31314=CARTESIAN_POINT('Ctrl Pts',(-31.4055367574321,33.7276111853924,8.));
#31315=CARTESIAN_POINT('Ctrl Pts',(-31.4407595052535,33.6159144227599,8.));
#31316=CARTESIAN_POINT('Ctrl Pts',(-31.4627247636627,33.5462592025841,8.));
#31317=CARTESIAN_POINT('Ctrl Pts',(-31.4868311858377,33.4771676502711,8.));
#31318=CARTESIAN_POINT('Ctrl Pts',(-31.5130143786684,33.4087065804238,8.));
#31319=CARTESIAN_POINT('Ctrl Pts',(-31.5219642258836,33.3853054574484,8.));
#31320=CARTESIAN_POINT('Ctrl Pts',(-31.5311567813561,33.3619780190094,8.));
#31321=CARTESIAN_POINT('Ctrl Pts',(-31.5405896605283,33.3387270021894,8.));
#31322=CARTESIAN_POINT('Ctrl Pts',(-31.5473384631411,33.3220919409105,8.));
#31323=CARTESIAN_POINT('Ctrl Pts',(-31.5542108294608,33.3054948782145,8.));
#31324=CARTESIAN_POINT('Ctrl Pts',(-31.5611988172515,33.288953116597,8.));
#31325=CARTESIAN_POINT('Ctrl Pts',(-31.6071201467481,33.1802494799514,8.));
#31326=CARTESIAN_POINT('Ctrl Pts',(-31.6580945083799,33.0737722290612,8.));
#31327=CARTESIAN_POINT('Ctrl Pts',(-31.7137634608477,32.9697757128959,8.));
#31328=CARTESIAN_POINT('Ctrl Pts',(-31.7713476440883,32.8622013078145,8.));
#31329=CARTESIAN_POINT('Ctrl Pts',(-31.8339551704749,32.7572805788209,8.));
#31330=CARTESIAN_POINT('Ctrl Pts',(-31.9012446980031,32.6553023741411,8.));
#31331=CARTESIAN_POINT('Ctrl Pts',(-31.9691674082359,32.552364572362,8.));
#31332=CARTESIAN_POINT('Ctrl Pts',(-32.0418610824791,32.4524241883893,8.));
#31333=CARTESIAN_POINT('Ctrl Pts',(-32.1190251653974,32.3557965754622,8.));
#31334=CARTESIAN_POINT('Ctrl Pts',(-32.1734382985285,32.2876585121627,8.));
#31335=CARTESIAN_POINT('Ctrl Pts',(-32.2300754238941,32.2211680942644,8.));
#31336=CARTESIAN_POINT('Ctrl Pts',(-32.2888442072745,32.1564443823762,8.));
#31337=CARTESIAN_POINT('Ctrl Pts',(-32.3150764518969,32.1275540745384,8.));
#31338=CARTESIAN_POINT('Ctrl Pts',(-32.341733542045,32.0990158743987,8.));
#31339=CARTESIAN_POINT('Ctrl Pts',(-32.3688078763672,32.0708409435943,8.));
#31340=CARTESIAN_POINT('Ctrl Pts',(-32.3804297629888,32.0587466166393,8.));
#31341=CARTESIAN_POINT('Ctrl Pts',(-32.3921271141324,32.0467207651166,8.));
#31342=CARTESIAN_POINT('Ctrl Pts',(-32.4038928229971,32.0347706553995,8.));
#31343=CARTESIAN_POINT('Ctrl Pts',(-32.4923350889694,31.9449422571145,8.));
#31344=CARTESIAN_POINT('Ctrl Pts',(-32.5847366887113,31.8592864840437,8.));
#31345=CARTESIAN_POINT('Ctrl Pts',(-32.6807688805232,31.7781214891551,8.));
#31346=CARTESIAN_POINT('Ctrl Pts',(-32.7628090255767,31.7087823662183,8.));
#31347=CARTESIAN_POINT('Ctrl Pts',(-32.8474998792406,31.6427207947673,8.));
#31348=CARTESIAN_POINT('Ctrl Pts',(-32.9346606964287,31.5801527068548,8.));
#31349=CARTESIAN_POINT('Ctrl Pts',(-32.9737718119822,31.5520769292834,8.));
#31350=CARTESIAN_POINT('Ctrl Pts',(-33.0133805354119,31.5247048259746,8.));
#31351=CARTESIAN_POINT('Ctrl Pts',(-33.0534717786847,31.4980572637843,8.));
#31352=CARTESIAN_POINT('Ctrl Pts',(-33.0807061080661,31.4799553435978,8.));
#31353=CARTESIAN_POINT('Ctrl Pts',(-33.1081687455454,31.4621843968183,8.));
#31354=CARTESIAN_POINT('Ctrl Pts',(-33.1358249991596,31.4447697393726,8.));
#31355=CARTESIAN_POINT('Ctrl Pts',(-33.2426293820058,31.3775168942506,8.));
#31356=CARTESIAN_POINT('Ctrl Pts',(-33.3523804860194,31.3155308622806,8.));
#31357=CARTESIAN_POINT('Ctrl Pts',(-33.464776332519,31.2591453036981,8.));
#31358=CARTESIAN_POINT('Ctrl Pts',(-33.5668700198747,31.2079280232686,8.));
#31359=CARTESIAN_POINT('Ctrl Pts',(-33.671146627403,31.161331555616,8.));
#31360=CARTESIAN_POINT('Ctrl Pts',(-33.7774031884393,31.1196350702262,8.));
#31361=CARTESIAN_POINT('Ctrl Pts',(-33.8328337169093,31.0978833948665,8.));
#31362=CARTESIAN_POINT('Ctrl Pts',(-33.8888033971972,31.0774656906331,8.));
#31363=CARTESIAN_POINT('Ctrl Pts',(-33.9452681066883,31.058369845356,8.));
#31364=CARTESIAN_POINT('Ctrl Pts',(-36.0520713770612,31.0647048309474,8.));
#31365=CARTESIAN_POINT('Ctrl Pts',(-36.168179415234,31.1043194708775,8.));
#31366=CARTESIAN_POINT('Ctrl Pts',(-36.2820223922111,31.1494845221288,8.));
#31367=CARTESIAN_POINT('Ctrl Pts',(-36.3933744144291,31.1998423763314,8.));
#31368=CARTESIAN_POINT('Ctrl Pts',(-36.5072236213378,31.25132955769,8.));
#31369=CARTESIAN_POINT('Ctrl Pts',(-36.6184695195224,31.3082455598905,8.));
#31370=CARTESIAN_POINT('Ctrl Pts',(-36.7268464017735,31.3702567471293,8.));
#31371=CARTESIAN_POINT('Ctrl Pts',(-36.8407847815347,31.4354501172862,8.));
#31372=CARTESIAN_POINT('Ctrl Pts',(-36.9515531074568,31.5062754464572,8.));
#31373=CARTESIAN_POINT('Ctrl Pts',(-37.0588034719145,31.5823912510781,8.));
#31374=CARTESIAN_POINT('Ctrl Pts',(-37.152647540815,31.6489925801213,8.));
#31375=CARTESIAN_POINT('Ctrl Pts',(-37.2437978659804,31.7196454871349,8.));
#31376=CARTESIAN_POINT('Ctrl Pts',(-37.3319898787643,31.7941433466814,8.));
#31377=CARTESIAN_POINT('Ctrl Pts',(-37.3493659727369,31.8088213403836,8.));
#31378=CARTESIAN_POINT('Ctrl Pts',(-37.3666271256303,31.8236486435546,8.));
#31379=CARTESIAN_POINT('Ctrl Pts',(-37.3837711593319,31.8386237468057,8.));
#31380=CARTESIAN_POINT('Ctrl Pts',(-37.3963054555396,31.8495723008716,8.));
#31381=CARTESIAN_POINT('Ctrl Pts',(-37.4087759352647,31.8605988651726,8.));
#31382=CARTESIAN_POINT('Ctrl Pts',(-37.4211729491963,31.8716947276461,8.));
#31383=CARTESIAN_POINT('Ctrl Pts',(-37.5137521425834,31.9545571010691,8.));
#31384=CARTESIAN_POINT('Ctrl Pts',(-37.6023754843508,32.0414011788236,8.));
#31385=CARTESIAN_POINT('Ctrl Pts',(-37.6867815485414,32.1319060425465,8.));
#31386=CARTESIAN_POINT('Ctrl Pts',(-37.7709958473242,32.2222052847627,8.));
#31387=CARTESIAN_POINT('Ctrl Pts',(-37.8510125269352,32.3161494024035,8.));
#31388=CARTESIAN_POINT('Ctrl Pts',(-37.9265315102947,32.413451696318,8.));
#31389=CARTESIAN_POINT('Ctrl Pts',(-38.0010181696068,32.5094238942302,8.));
#31390=CARTESIAN_POINT('Ctrl Pts',(-38.0711296560004,32.6086637703888,8.));
#31391=CARTESIAN_POINT('Ctrl Pts',(-38.1365319925539,32.7109170507384,8.));
#31392=CARTESIAN_POINT('Ctrl Pts',(-38.189837488265,32.7942575257788,8.));
#31393=CARTESIAN_POINT('Ctrl Pts',(-38.2400140119095,32.8796002993686,8.));
#31394=CARTESIAN_POINT('Ctrl Pts',(-38.2868547984211,32.966813541324,8.));
#31395=CARTESIAN_POINT('Ctrl Pts',(-38.2987553976748,32.9889713640128,8.));
#31396=CARTESIAN_POINT('Ctrl Pts',(-38.3104405526761,33.0112499393599,8.));
#31397=CARTESIAN_POINT('Ctrl Pts',(-38.3219066094193,33.0336471306571,8.));
#31398=CARTESIAN_POINT('Ctrl Pts',(-38.3300627268695,33.0495788608817,8.));
#31399=CARTESIAN_POINT('Ctrl Pts',(-38.3381042716881,33.0655634268488,8.));
#31400=CARTESIAN_POINT('Ctrl Pts',(-38.3460275803167,33.0815944092568,8.));
#31401=CARTESIAN_POINT('Ctrl Pts',(-38.3989884279579,33.1887484350122,8.));
#31402=CARTESIAN_POINT('Ctrl Pts',(-38.4467104251109,33.2980523321741,8.));
#31403=CARTESIAN_POINT('Ctrl Pts',(-38.4889147723839,33.409243488173,8.));
#31404=CARTESIAN_POINT('Ctrl Pts',(-38.5302829624144,33.5182317125689,8.));
#31405=CARTESIAN_POINT('Ctrl Pts',(-38.5663502410402,33.6290337883757,8.));
#31406=CARTESIAN_POINT('Ctrl Pts',(-38.596805840802,33.7414161893267,8.));
#31407=CARTESIAN_POINT('Ctrl Pts',(-38.6012600218942,33.7578522985917,8.));
#31408=CARTESIAN_POINT('Ctrl Pts',(-38.6055940819337,33.7743222252706,8.));
#31409=CARTESIAN_POINT('Ctrl Pts',(-38.6098069546845,33.7908252519299,8.));
#31410=CARTESIAN_POINT('Ctrl Pts',(-38.6394755059943,33.9070454470715,8.));
#31411=CARTESIAN_POINT('Ctrl Pts',(-38.6631380748325,34.0249075695662,8.));
#31412=CARTESIAN_POINT('Ctrl Pts',(-38.6808855164532,34.1439757769513,8.));
#31413=CARTESIAN_POINT('Ctrl Pts',(-38.6908690551697,34.2109556878445,8.));
#31414=CARTESIAN_POINT('Ctrl Pts',(-38.6989798315808,34.2783172077624,8.));
#31415=CARTESIAN_POINT('Ctrl Pts',(-38.7052269705051,34.3459812971573,8.));
#31416=CARTESIAN_POINT('Ctrl Pts',(-38.7081094451816,34.3772019929916,8.));
#31417=CARTESIAN_POINT('Ctrl Pts',(-38.7105950890294,34.4084870828833,8.));
#31418=CARTESIAN_POINT('Ctrl Pts',(-38.712684450918,34.4398286677084,8.));
#31419=CARTESIAN_POINT('Ctrl Pts',(-38.7138855420385,34.457845699339,8.));
#31420=CARTESIAN_POINT('Ctrl Pts',(-38.7149551618269,34.47587434695,8.));
#31421=CARTESIAN_POINT('Ctrl Pts',(-38.7158933795518,34.4939047698972,8.));
#31422=CARTESIAN_POINT('Ctrl Pts',(-38.722204302566,34.6151864384397,8.));
#31423=CARTESIAN_POINT('Ctrl Pts',(-38.7225826970351,34.7366654075262,8.));
#31424=CARTESIAN_POINT('Ctrl Pts',(-38.7171867711641,34.8578944234449,8.));
#31425=CARTESIAN_POINT('Ctrl Pts',(-38.7119027789398,34.9766086520668,8.));
#31426=CARTESIAN_POINT('Ctrl Pts',(-38.7010810476264,35.0950841138035,8.));
#31427=CARTESIAN_POINT('Ctrl Pts',(-38.6848167703974,35.2128948265086,8.));
#31428=CARTESIAN_POINT('Ctrl Pts',(-38.6687114015083,35.3295544825446,8.));
#31429=CARTESIAN_POINT('Ctrl Pts',(-38.6472689687305,35.445563152418,8.));
#31430=CARTESIAN_POINT('Ctrl Pts',(-38.6205351191465,35.5604883182129,8.));
#31431=CARTESIAN_POINT('Ctrl Pts',(-38.603128213054,35.6353182285994,8.));
#31432=CARTESIAN_POINT('Ctrl Pts',(-38.5834770455875,35.7096883679731,8.));
#31433=CARTESIAN_POINT('Ctrl Pts',(-38.5615844164204,35.7834724389555,8.));
#31434=CARTESIAN_POINT('Ctrl Pts',(-38.5541960688544,35.8083731649983,8.));
#31435=CARTESIAN_POINT('Ctrl Pts',(-38.546552371059,35.8332070872086,8.));
#31436=CARTESIAN_POINT('Ctrl Pts',(-38.5386532430018,35.8579691742342,8.));
#31437=CARTESIAN_POINT('Ctrl Pts',(-38.533566838996,35.8739139693719,8.));
#31438=CARTESIAN_POINT('Ctrl Pts',(-38.5283753166192,35.8898263677189,8.));
#31439=CARTESIAN_POINT('Ctrl Pts',(-38.5230815350611,35.9056970029845,8.));
#31440=CARTESIAN_POINT('Ctrl Pts',(-38.4861838533105,36.0163154036073,8.));
#31441=CARTESIAN_POINT('Ctrl Pts',(-38.4442854600859,36.1250223270562,8.));
#31442=CARTESIAN_POINT('Ctrl Pts',(-38.3974511486834,36.2313985734173,8.));
#31443=CARTESIAN_POINT('Ctrl Pts',(-38.3593370627389,36.3179682970844,8.));
#31444=CARTESIAN_POINT('Ctrl Pts',(-38.3179530705292,36.4029942704614,8.));
#31445=CARTESIAN_POINT('Ctrl Pts',(-38.2733131103528,36.4862349013589,8.));
#31446=CARTESIAN_POINT('Ctrl Pts',(-38.2516981197193,36.52654061512,8.));
#31447=CARTESIAN_POINT('Ctrl Pts',(-38.2293194750761,36.5664275009295,8.));
#31448=CARTESIAN_POINT('Ctrl Pts',(-38.2061772856241,36.6058666059334,8.));
#31449=CARTESIAN_POINT('Ctrl Pts',(-38.1925908747914,36.6290206763194,8.));
#31450=CARTESIAN_POINT('Ctrl Pts',(-38.1787392319563,36.6520234773565,8.));
#31451=CARTESIAN_POINT('Ctrl Pts',(-38.1646364321387,36.6748466577435,8.));
#31452=CARTESIAN_POINT('Ctrl Pts',(-38.1062049879234,36.7694088304221,8.));
#31453=CARTESIAN_POINT('Ctrl Pts',(-38.0434222829092,36.8609657921147,8.));
#31454=CARTESIAN_POINT('Ctrl Pts',(-37.9763223631119,36.9491268302023,8.));
#31455=CARTESIAN_POINT('Ctrl Pts',(-37.9162915853069,37.0279998855573,8.));
#31456=CARTESIAN_POINT('Ctrl Pts',(-37.8528047083354,37.1041548125789,8.));
#31457=CARTESIAN_POINT('Ctrl Pts',(-37.7858626225071,37.1772853000647,8.));
#31458=CARTESIAN_POINT('Ctrl Pts',(-37.7510076908282,37.2153623649398,8.));
#31459=CARTESIAN_POINT('Ctrl Pts',(-37.7152156561398,37.2526190163742,8.));
#31460=CARTESIAN_POINT('Ctrl Pts',(-37.6785239274887,37.2890398567007,8.));
#31461=CARTESIAN_POINT('Origin',(-35.,-35.,10.2084234471775));
#31462=CARTESIAN_POINT('Ctrl Pts',(-39.0784093524563,-34.997955826836,7.70842344717746));
#31463=CARTESIAN_POINT('Ctrl Pts',(-39.0792534643083,-34.8668875745646,
7.70328437820511));
#31464=CARTESIAN_POINT('Ctrl Pts',(-39.0145241717454,-33.401902569157,7.64581193344868));
#31465=CARTESIAN_POINT('Ctrl Pts',(-37.2468182307978,-30.7615622415685,
7.53600611290816));
#31466=CARTESIAN_POINT('Ctrl Pts',(-32.7044906448315,-30.7882310811688,
7.37900598555592));
#31467=CARTESIAN_POINT('Ctrl Pts',(-30.2206288723714,-34.591050784955,7.22200585820366));
#31468=CARTESIAN_POINT('Ctrl Pts',(-32.0224449816578,-38.760868439734,7.06500573085141));
#31469=CARTESIAN_POINT('Ctrl Pts',(-36.4942781630208,-39.5581356918704,
6.90800560349915));
#31470=CARTESIAN_POINT('Ctrl Pts',(-38.8653532597229,-37.0673722499186,
6.78914484227451));
#31471=CARTESIAN_POINT('Ctrl Pts',(-39.0751760778997,-35.366983894328,6.72261745683394));
#31472=CARTESIAN_POINT('Ctrl Pts',(-39.0721140267755,-35.0034548068065,
6.70842344717746));
#31473=CARTESIAN_POINT('Ctrl Pts',(-39.0691247390887,-35.0040754761348,
7.79157655282255));
#31474=CARTESIAN_POINT('Ctrl Pts',(-39.0629617458988,-34.1015748206833,
7.75638428364687));
#31475=CARTESIAN_POINT('Ctrl Pts',(-38.3270258918815,-31.8449563360523,
7.6688586386871));
#31476=CARTESIAN_POINT('Ctrl Pts',(-34.6204730922247,-30.2191423808613,
7.52899961794324));
#31477=CARTESIAN_POINT('Ctrl Pts',(-30.8030823517117,-32.6774434597138,
7.37199949059099));
#31478=CARTESIAN_POINT('Ctrl Pts',(-30.7475655592404,-37.2202136561835,
7.21499936323873));
#31479=CARTESIAN_POINT('Ctrl Pts',(-34.5060129709306,-39.7711989299046,
7.05799923588648));
#31480=CARTESIAN_POINT('Ctrl Pts',(-38.2826810114871,-38.2186958612719,
6.91685829908109));
#31481=CARTESIAN_POINT('Ctrl Pts',(-39.0636923276262,-35.9315794222149,
6.82805073805978));
#31482=CARTESIAN_POINT('Ctrl Pts',(-39.0709664927331,-34.9967444357251,
6.79157655282255));
#31483=CARTESIAN_POINT('Ctrl Pts',(-32.3264680662287,-32.7141668369925,
8.));
#31484=CARTESIAN_POINT('Ctrl Pts',(-31.5748397248436,-33.5932784036375,
7.94766662421592));
#31485=CARTESIAN_POINT('Ctrl Pts',(-31.0185761455706,-36.1362135079881,
7.84299987264775));
#31486=CARTESIAN_POINT('Ctrl Pts',(-33.7549095310954,-38.9529268308332,
7.68599974529549));
#31487=CARTESIAN_POINT('Ctrl Pts',(-37.6085237505035,-38.2165103725086,
7.52899961794325));
#31488=CARTESIAN_POINT('Ctrl Pts',(-39.122629513254,-34.5999498459216,7.37199949059098));
#31489=CARTESIAN_POINT('Ctrl Pts',(-36.940145606194,-31.3400749195329,7.21499936323873));
#31490=CARTESIAN_POINT('Ctrl Pts',(-33.0178092164465,-31.3631036769391,
7.05799923588649));
#31491=CARTESIAN_POINT('Ctrl Pts',(-30.8729746062518,-34.6468690649513,
6.90099910853422));
#31492=CARTESIAN_POINT('Ctrl Pts',(-32.4288573028063,-38.2475401342247,
6.74399898118198));
#31493=CARTESIAN_POINT('Ctrl Pts',(-36.2903212074201,-38.9359868162892,
6.58699885382972));
#31494=CARTESIAN_POINT('Ctrl Pts',(-38.9947353103719,-36.0950579107052,
6.42999872647747));
#31495=CARTESIAN_POINT('Ctrl Pts',(-38.117035111845,-32.2721495171465,6.27299859912521));
#31496=CARTESIAN_POINT('Ctrl Pts',(-34.444258048923,-30.8953459884408,6.11599847177297));
#31497=CARTESIAN_POINT('Ctrl Pts',(-31.2698209074708,-33.1992175611906,
5.9589983444207));
#31498=CARTESIAN_POINT('Ctrl Pts',(-31.4402707556255,-37.1178717601522,
5.80199821706845));
#31499=CARTESIAN_POINT('Ctrl Pts',(-34.8027641605008,-39.1374081785836,
5.6449980897162));
#31500=CARTESIAN_POINT('Ctrl Pts',(-38.3421207391464,-37.4468919117391,
5.48799796236395));
#31501=CARTESIAN_POINT('Ctrl Pts',(-38.8845656356524,-33.5622237360543,
5.33099783501169));
#31502=CARTESIAN_POINT('Ctrl Pts',(-35.943683236251,-30.9668235565892,5.17399770765944));
#31503=CARTESIAN_POINT('Ctrl Pts',(-32.1565910373224,-31.9880112738199,
5.01699758030718));
#31504=CARTESIAN_POINT('Ctrl Pts',(-30.919210927847,-35.7100782334501,4.85999745295493));
#31505=CARTESIAN_POINT('Ctrl Pts',(-33.3411135315715,-38.7954112012017,
4.70299732560268));
#31506=CARTESIAN_POINT('Ctrl Pts',(-37.2505555447442,-38.477362547094,4.54599719825042));
#31507=CARTESIAN_POINT('Ctrl Pts',(-39.141902810795,-35.0411295298515,4.38899707089817));
#31508=CARTESIAN_POINT('Ctrl Pts',(-37.3191660904533,-31.5680152720272,
4.23199694354592));
#31509=CARTESIAN_POINT('Ctrl Pts',(-33.4168108878721,-31.1723946430222,
4.07499681619366));
#31510=CARTESIAN_POINT('Ctrl Pts',(-30.9341165505443,-34.2090244589174,
3.91799668884141));
#31511=CARTESIAN_POINT('Ctrl Pts',(-32.0973389085718,-37.9549296302039,
3.76099656148916));
#31512=CARTESIAN_POINT('Ctrl Pts',(-35.8634053144019,-39.0511210542994,
3.6039964341369));
#31513=CARTESIAN_POINT('Ctrl Pts',(-38.8552478911374,-36.5146333635664,
3.44699630678465));
#31514=CARTESIAN_POINT('Ctrl Pts',(-38.3900526994102,-32.6199594063295,
3.2899961794324));
#31515=CARTESIAN_POINT('Ctrl Pts',(-34.8849647272175,-30.8594906798889,
3.13299605208015));
#31516=CARTESIAN_POINT('Ctrl Pts',(-31.4830299921864,-32.8118563882867,
2.97599592472789));
#31517=CARTESIAN_POINT('Ctrl Pts',(-31.2347959944593,-36.726351454856,2.81899579737564));
#31518=CARTESIAN_POINT('Ctrl Pts',(-34.3628565683332,-39.0928106312356,
2.66199567002338));
#31519=CARTESIAN_POINT('Ctrl Pts',(-38.0622497333952,-37.7892072071444,
2.50499554267113));
#31520=CARTESIAN_POINT('Ctrl Pts',(-39.0156942580864,-33.9844950081716,
2.34799541531887));
#31521=CARTESIAN_POINT('Ctrl Pts',(-36.3682270687435,-31.0903957040226,
2.19099528796663));
#31522=CARTESIAN_POINT('Ctrl Pts',(-32.4938578387906,-31.7020764289629,
2.03399516061437));
#31523=CARTESIAN_POINT('Ctrl Pts',(-30.866769727096,-35.2710361541464,1.87699503326212));
#31524=CARTESIAN_POINT('Ctrl Pts',(-32.9459900633082,-38.5969565794207,
1.71999490590986));
#31525=CARTESIAN_POINT('Ctrl Pts',(-36.8670583779424,-38.6974486722808,
1.56299477855761));
#31526=CARTESIAN_POINT('Ctrl Pts',(-39.1139224428247,-35.4824088304557,
1.40599465120536));
#31527=CARTESIAN_POINT('Ctrl Pts',(-37.6717828958998,-31.8347767559132,
1.2489945238531));
#31528=CARTESIAN_POINT('Ctrl Pts',(-33.8338499179097,-31.0254541111767,
1.09199439650085));
#31529=CARTESIAN_POINT('Ctrl Pts',(-31.0415747701051,-33.7800977940573,
0.934994269148597));
#31530=CARTESIAN_POINT('Ctrl Pts',(-31.7989383549478,-37.6287343727556,
0.777994141796342));
#31531=CARTESIAN_POINT('Ctrl Pts',(-35.4265617474899,-39.1199684759325,
0.620994014444089));
#31532=CARTESIAN_POINT('Ctrl Pts',(-38.6720112486245,-36.9171723860524,
0.463993887091836));
#31533=CARTESIAN_POINT('Ctrl Pts',(-38.6240720221873,-32.9944536386984,
0.306993759739581));
#31534=CARTESIAN_POINT('Ctrl Pts',(-35.3277245214386,-30.8716914151866,
0.149993632387329));
#31535=CARTESIAN_POINT('Ctrl Pts',(-31.7348166906651,-32.4476562217995,
-0.00700649496492554));
#31536=CARTESIAN_POINT('Ctrl Pts',(-31.0753023569953,-36.3188879616356,
-0.164006622317179));
#31537=CARTESIAN_POINT('Ctrl Pts',(-32.9741442474368,-38.0994349533405,
-0.268673373885348));
#31538=CARTESIAN_POINT('Ctrl Pts',(-34.0915279074966,-38.3981590173419,
-0.321006749669432));
#31539=CARTESIAN_POINT('Ctrl Pts',(-32.1856025125516,-32.5937287191406,
8.10700224988981));
#31540=CARTESIAN_POINT('Ctrl Pts',(-31.3943716733878,-33.5191597390956,
8.05466887410573));
#31541=CARTESIAN_POINT('Ctrl Pts',(-30.8087991578366,-36.1960793891008,
7.95000212253755));
#31542=CARTESIAN_POINT('Ctrl Pts',(-33.6893070387277,-39.1612023407069,
7.79300199518531));
#31543=CARTESIAN_POINT('Ctrl Pts',(-37.7459640921552,-38.3859848825408,
7.63600186783305));
#31544=CARTESIAN_POINT('Ctrl Pts',(-39.3398464769469,-34.5788716288481,
7.4790017404808));
#31545=CARTESIAN_POINT('Ctrl Pts',(-37.0423698143953,-31.1472373602114,
7.32200161312854));
#31546=CARTESIAN_POINT('Ctrl Pts',(-32.9133696925748,-31.171479478349,7.1650014857763));
#31547=CARTESIAN_POINT('Ctrl Pts',(-30.6555260282916,-34.6282629716192,
7.00800135842403));
#31548=CARTESIAN_POINT('Ctrl Pts',(-32.2933865290902,-38.4186495693944,
6.85100123107179));
#31549=CARTESIAN_POINT('Ctrl Pts',(-36.358306859287,-39.1433697748163,6.69400110371953));
#31550=CARTESIAN_POINT('Ctrl Pts',(-39.2052136645597,-36.1527553471755,
6.53700097636729));
#31551=CARTESIAN_POINT('Ctrl Pts',(-38.2812683762075,-32.1284219768986,
6.38000084901502));
#31552=CARTESIAN_POINT('Ctrl Pts',(-34.4149765966796,-30.6790761348112,
6.22300072166278));
#31553=CARTESIAN_POINT('Ctrl Pts',(-31.073281738985,-33.1043362500341,6.06600059431052));
#31554=CARTESIAN_POINT('Ctrl Pts',(-31.2527124083266,-37.2294601703531,
5.90900046695826));
#31555=CARTESIAN_POINT('Ctrl Pts',(-34.792372013923,-39.3554038144322,5.75200033960602));
#31556=CARTESIAN_POINT('Ctrl Pts',(-38.5182135257814,-37.5758160437388,
5.59500021225375));
#31557=CARTESIAN_POINT('Ctrl Pts',(-39.0892392668699,-33.4864688341112,
5.43800008490151));
#31558=CARTESIAN_POINT('Ctrl Pts',(-35.9934049021458,-30.7543197799925,
5.28099995754925));
#31559=CARTESIAN_POINT('Ctrl Pts',(-32.0067748436954,-31.8293127917771,
5.12399983019699));
#31560=CARTESIAN_POINT('Ctrl Pts',(-30.7041984924888,-35.7474915002398,
4.96699970284474));
#31561=CARTESIAN_POINT('Ctrl Pts',(-33.2537085681557,-38.9953873801041,
4.80999957549249));
#31562=CARTESIAN_POINT('Ctrl Pts',(-37.3691349224156,-38.6605810807291,
4.65299944814024));
#31563=CARTESIAN_POINT('Ctrl Pts',(-39.3601352640338,-35.0432966010287,
4.49599932078798));
#31564=CARTESIAN_POINT('Ctrl Pts',(-37.4413604847951,-31.3871876474119,
4.33899919343573));
#31565=CARTESIAN_POINT('Ctrl Pts',(-33.3333943376382,-30.9707221882978,
4.18199906608348));
#31566=CARTESIAN_POINT('Ctrl Pts',(-30.7198894765905,-34.1673487990413,
4.02499893873122));
#31567=CARTESIAN_POINT('Ctrl Pts',(-31.9444007833091,-38.1106217291751,
3.86799881137897));
#31568=CARTESIAN_POINT('Ctrl Pts',(-35.9088972219885,-39.2645703133555,
3.71099868402671));
#31569=CARTESIAN_POINT('Ctrl Pts',(-39.0583768015825,-36.5944377843333,
3.55399855667446));
#31570=CARTESIAN_POINT('Ctrl Pts',(-38.5686709700449,-32.4945575991672,
3.39699842932221));
#31571=CARTESIAN_POINT('Ctrl Pts',(-34.8789036410609,-30.641331648192,3.23999830196996));
#31572=CARTESIAN_POINT('Ctrl Pts',(-31.2977245835776,-32.6965654289773,
3.0829981746177));
#31573=CARTESIAN_POINT('Ctrl Pts',(-31.0364114005639,-36.8173110766423,
2.92599804726545));
#31574=CARTESIAN_POINT('Ctrl Pts',(-34.3292861586667,-39.3084564697542,
2.76899791991319));
#31575=CARTESIAN_POINT('Ctrl Pts',(-38.2235964144439,-37.9361675679284,
2.61199779256094));
#31576=CARTESIAN_POINT('Ctrl Pts',(-39.2272769169348,-33.9309891303743,
2.45499766520869));
#31577=CARTESIAN_POINT('Ctrl Pts',(-36.4403174975728,-30.8844028124269,
2.29799753785644));
#31578=CARTESIAN_POINT('Ctrl Pts',(-32.3618118741726,-31.5283123441018,
2.14099741050418));
#31579=CARTESIAN_POINT('Ctrl Pts',(-30.6489942206534,-35.2853167607994,
1.98399728315193));
#31580=CARTESIAN_POINT('Ctrl Pts',(-32.8377664646538,-38.7864763954034,
1.82699715579967));
#31581=CARTESIAN_POINT('Ctrl Pts',(-36.9654316978321,-38.89226330974,1.66999702844742));
#31582=CARTESIAN_POINT('Ctrl Pts',(-39.3306806402386,-35.5078264385801,
1.51299690109516));
#31583=CARTESIAN_POINT('Ctrl Pts',(-37.8125562946319,-31.668004510122,1.35599677374291));
#31584=CARTESIAN_POINT('Ctrl Pts',(-33.7724067105519,-30.8160395161343,
1.19899664639066));
#31585=CARTESIAN_POINT('Ctrl Pts',(-30.8330095554335,-33.7158224444716,
1.04199651903841));
#31586=CARTESIAN_POINT('Ctrl Pts',(-31.630277821932,-37.7672395905951,0.884996391686153));
#31587=CARTESIAN_POINT('Ctrl Pts',(-35.4490368322191,-39.3370452323995,
0.727996264333899));
#31588=CARTESIAN_POINT('Ctrl Pts',(-38.8654856152897,-37.0181861597217,
0.570996136981647));
#31589=CARTESIAN_POINT('Ctrl Pts',(-38.815020522006,-32.8887835342792,0.413996009629392));
#31590=CARTESIAN_POINT('Ctrl Pts',(-35.3449919778631,-30.6541752272542,
0.256995882277139));
#31591=CARTESIAN_POINT('Ctrl Pts',(-31.5627776553664,-32.3131759431282,
0.0999957549248853));
#31592=CARTESIAN_POINT('Ctrl Pts',(-30.8685142129999,-36.3883787653949,
-0.0570043724273683));
#31593=CARTESIAN_POINT('Ctrl Pts',(-32.8674040627957,-38.2627408840732,
-0.161671123995537));
#31594=CARTESIAN_POINT('Ctrl Pts',(-34.0436614793107,-38.5772044012455,
-0.214004499779622));
#31595=CARTESIAN_POINT('Ctrl Pts',(-32.0447369588746,-32.4732906012887,
8.21400449977962));
#31596=CARTESIAN_POINT('Ctrl Pts',(-31.2139036219321,-33.4450410745538,
8.16167112399554));
#31597=CARTESIAN_POINT('Ctrl Pts',(-30.5990221701027,-36.2559452702134,
8.05700437242737));
#31598=CARTESIAN_POINT('Ctrl Pts',(-33.6237045463599,-39.3694778505807,
7.90000424507512));
#31599=CARTESIAN_POINT('Ctrl Pts',(-37.883404433807,-38.555459392573,7.74300411772286));
#31600=CARTESIAN_POINT('Ctrl Pts',(-39.5570634406398,-34.5577934117747,
7.58600399037061));
#31601=CARTESIAN_POINT('Ctrl Pts',(-37.1445940225965,-30.95439980089,7.42900386301835));
#31602=CARTESIAN_POINT('Ctrl Pts',(-32.8089301687032,-30.9798552797588,
7.2720037356661));
#31603=CARTESIAN_POINT('Ctrl Pts',(-30.4380774503315,-34.6096568782872,
7.11500360831385));
#31604=CARTESIAN_POINT('Ctrl Pts',(-32.157915755374,-38.5897590045642,6.9580034809616));
#31605=CARTESIAN_POINT('Ctrl Pts',(-36.4262925111539,-39.3507527333434,
6.80100335360934));
#31606=CARTESIAN_POINT('Ctrl Pts',(-39.4156920187475,-36.2104527836457,
6.64400322625709));
#31607=CARTESIAN_POINT('Ctrl Pts',(-38.4455016405701,-31.9846944366506,
6.48700309890483));
#31608=CARTESIAN_POINT('Ctrl Pts',(-34.3856951444362,-30.4628062811815,
6.33000297155259));
#31609=CARTESIAN_POINT('Ctrl Pts',(-30.8767425704992,-33.0094549388777,
6.17300284420032));
#31610=CARTESIAN_POINT('Ctrl Pts',(-31.0651540610276,-37.3410485805539,
6.01600271684808));
#31611=CARTESIAN_POINT('Ctrl Pts',(-34.7819798673453,-39.5733994502808,
5.85900258949582));
#31612=CARTESIAN_POINT('Ctrl Pts',(-38.6943063124164,-37.7047401757385,
5.70200246214356));
#31613=CARTESIAN_POINT('Ctrl Pts',(-39.2939128980875,-33.4107139321682,
5.54500233479131));
#31614=CARTESIAN_POINT('Ctrl Pts',(-36.0431265680407,-30.5418160033959,
5.38800220743906));
#31615=CARTESIAN_POINT('Ctrl Pts',(-31.8569586500684,-31.6706143097344,
5.2310020800868));
#31616=CARTESIAN_POINT('Ctrl Pts',(-30.4891860571307,-35.7849047670295,
5.07400195273456));
#31617=CARTESIAN_POINT('Ctrl Pts',(-33.1663036047398,-39.1953635590066,
4.9170018253823));
#31618=CARTESIAN_POINT('Ctrl Pts',(-37.487714300087,-38.8437996143642,4.76000169803005));
#31619=CARTESIAN_POINT('Ctrl Pts',(-39.5783677172726,-35.0454636722059,
4.60300157067779));
#31620=CARTESIAN_POINT('Ctrl Pts',(-37.563554879137,-31.2063600227966,4.44600144332554));
#31621=CARTESIAN_POINT('Ctrl Pts',(-33.2499777874043,-30.7690497335734,
4.28900131597329));
#31622=CARTESIAN_POINT('Ctrl Pts',(-30.5056624026368,-34.1256731391653,
4.13200118862103));
#31623=CARTESIAN_POINT('Ctrl Pts',(-31.7914626580464,-38.2663138281463,
3.97500106126878));
#31624=CARTESIAN_POINT('Ctrl Pts',(-35.9543891295751,-39.4780195724117,
3.81800093391652));
#31625=CARTESIAN_POINT('Ctrl Pts',(-39.2615057120276,-36.6742422051002,
3.66100080656427));
#31626=CARTESIAN_POINT('Ctrl Pts',(-38.7472892406796,-32.3691557920048,
3.50400067921202));
#31627=CARTESIAN_POINT('Ctrl Pts',(-34.8728425549044,-30.4231726164951,
3.34700055185977));
#31628=CARTESIAN_POINT('Ctrl Pts',(-31.1124191749688,-32.5812744696679,
3.19000042450751));
#31629=CARTESIAN_POINT('Ctrl Pts',(-30.8380268066686,-36.9082706984286,
3.03300029715526));
#31630=CARTESIAN_POINT('Ctrl Pts',(-34.295715749,-39.5241023082727,2.876000169803));
#31631=CARTESIAN_POINT('Ctrl Pts',(-38.3849430954928,-38.0831279287123,
2.71900004245075));
#31632=CARTESIAN_POINT('Ctrl Pts',(-39.438859575783,-33.8774832525769,2.5619999150985));
#31633=CARTESIAN_POINT('Ctrl Pts',(-36.5124079264021,-30.6784099208313,
2.40499978774625));
#31634=CARTESIAN_POINT('Ctrl Pts',(-32.2297659095544,-31.3545482592407,
2.24799966039399));
#31635=CARTESIAN_POINT('Ctrl Pts',(-30.4312187142109,-35.2995973674523,
2.09099953304174));
#31636=CARTESIAN_POINT('Ctrl Pts',(-32.7295428659994,-38.9759962113862,
1.93399940568948));
#31637=CARTESIAN_POINT('Ctrl Pts',(-37.0638050177218,-39.0870779471991,
1.77699927833723));
#31638=CARTESIAN_POINT('Ctrl Pts',(-39.5474388376525,-35.5332440467046,
1.61999915098498));
#31639=CARTESIAN_POINT('Ctrl Pts',(-37.953329693364,-31.5012322643307,1.46299902363272));
#31640=CARTESIAN_POINT('Ctrl Pts',(-33.7109635031942,-30.6066249210918,
1.30599889628047));
#31641=CARTESIAN_POINT('Ctrl Pts',(-30.624444340762,-33.6515470948858,1.14899876892822));
#31642=CARTESIAN_POINT('Ctrl Pts',(-31.4616172889162,-37.9057448084347,
0.991998641575964));
#31643=CARTESIAN_POINT('Ctrl Pts',(-35.4715119169482,-39.5541219888666,
0.83499851422371));
#31644=CARTESIAN_POINT('Ctrl Pts',(-39.0589599819549,-37.1191999333909,
0.677998386871458));
#31645=CARTESIAN_POINT('Ctrl Pts',(-39.0059690218246,-32.78311342986,0.520998259519202));
#31646=CARTESIAN_POINT('Ctrl Pts',(-35.3622594342876,-30.4366590393219,
0.36399813216695));
#31647=CARTESIAN_POINT('Ctrl Pts',(-31.3907386200676,-32.1786956644568,
0.206998004814696));
#31648=CARTESIAN_POINT('Ctrl Pts',(-30.6617260690046,-36.4578695691541,
0.0499978774624427));
#31649=CARTESIAN_POINT('Ctrl Pts',(-32.7606638781546,-38.426046814806,-0.0546688741057264));
#31650=CARTESIAN_POINT('Ctrl Pts',(-33.9957950511247,-38.756249785149,-0.107002249889811));
#31651=CARTESIAN_POINT('Ctrl Pts',(-31.9038714051976,-32.3528524834368,
8.32100674966943));
#31652=CARTESIAN_POINT('Ctrl Pts',(-31.0334355704763,-33.370922410012,8.26867337388535));
#31653=CARTESIAN_POINT('Ctrl Pts',(-30.3892451823686,-36.3158111513261,
8.16400662231718));
#31654=CARTESIAN_POINT('Ctrl Pts',(-33.5581020539921,-39.5777533604545,
8.00700649496493));
#31655=CARTESIAN_POINT('Ctrl Pts',(-38.0208447754587,-38.7249339026052,
7.85000636761267));
#31656=CARTESIAN_POINT('Ctrl Pts',(-39.7742804043327,-34.5367151947012,
7.69300624026042));
#31657=CARTESIAN_POINT('Ctrl Pts',(-37.2468182307978,-30.7615622415685,
7.53600611290816));
#31658=CARTESIAN_POINT('Ctrl Pts',(-32.7044906448315,-30.7882310811688,
7.37900598555592));
#31659=CARTESIAN_POINT('Ctrl Pts',(-30.2206288723714,-34.591050784955,7.22200585820366));
#31660=CARTESIAN_POINT('Ctrl Pts',(-32.0224449816578,-38.760868439734,7.06500573085141));
#31661=CARTESIAN_POINT('Ctrl Pts',(-36.4942781630208,-39.5581356918704,
6.90800560349915));
#31662=CARTESIAN_POINT('Ctrl Pts',(-39.6261703729353,-36.2681502201159,
6.75100547614691));
#31663=CARTESIAN_POINT('Ctrl Pts',(-38.6097349049326,-31.8409668964026,
6.59400534879464));
#31664=CARTESIAN_POINT('Ctrl Pts',(-34.3564136921927,-30.2465364275518,
6.4370052214424));
#31665=CARTESIAN_POINT('Ctrl Pts',(-30.6802034020135,-32.9145736277213,
6.28000509409013));
#31666=CARTESIAN_POINT('Ctrl Pts',(-30.8775957137286,-37.4526369907548,
6.12300496673789));
#31667=CARTESIAN_POINT('Ctrl Pts',(-34.7715877207675,-39.7913950861294,
5.96600483938563));
#31668=CARTESIAN_POINT('Ctrl Pts',(-38.8703990990513,-37.8336643077382,
5.80900471203337));
#31669=CARTESIAN_POINT('Ctrl Pts',(-39.498586529305,-33.3349590302252,5.65200458468112));
#31670=CARTESIAN_POINT('Ctrl Pts',(-36.0928482339355,-30.3293122267992,
5.49500445732888));
#31671=CARTESIAN_POINT('Ctrl Pts',(-31.7071424564414,-31.5119158276916,
5.33800432997661));
#31672=CARTESIAN_POINT('Ctrl Pts',(-30.2741736217725,-35.8223180338192,
5.18100420262437));
#31673=CARTESIAN_POINT('Ctrl Pts',(-33.0788986413239,-39.395339737909,5.02400407527211));
#31674=CARTESIAN_POINT('Ctrl Pts',(-37.6062936777584,-39.0270181479993,
4.86700394791986));
#31675=CARTESIAN_POINT('Ctrl Pts',(-39.7966001705114,-35.0476307433831,
4.7100038205676));
#31676=CARTESIAN_POINT('Ctrl Pts',(-37.6857492734788,-31.0255323981813,
4.55300369321535));
#31677=CARTESIAN_POINT('Ctrl Pts',(-33.1665612371704,-30.5673772788489,
4.39600356586309));
#31678=CARTESIAN_POINT('Ctrl Pts',(-30.291435328683,-34.0839974792893,4.23900343851084));
#31679=CARTESIAN_POINT('Ctrl Pts',(-31.6385245327839,-38.4220059271175,
4.08200331115859));
#31680=CARTESIAN_POINT('Ctrl Pts',(-35.9998810371616,-39.6914688314679,
3.92500318380634));
#31681=CARTESIAN_POINT('Ctrl Pts',(-39.4646346224728,-36.7540466258671,
3.76800305645408));
#31682=CARTESIAN_POINT('Ctrl Pts',(-38.9259075113142,-32.2437539848424,
3.61100292910183));
#31683=CARTESIAN_POINT('Ctrl Pts',(-34.8667814687478,-30.2050135847982,
3.45400280174957));
#31684=CARTESIAN_POINT('Ctrl Pts',(-30.9271137663599,-32.4659835103585,
3.29700267439732));
#31685=CARTESIAN_POINT('Ctrl Pts',(-30.6396422127733,-36.9992303202149,
3.14000254704507));
#31686=CARTESIAN_POINT('Ctrl Pts',(-34.2621453393335,-39.7397481467912,
2.98300241969281));
#31687=CARTESIAN_POINT('Ctrl Pts',(-38.5462897765416,-38.2300882894962,
2.82600229234056));
#31688=CARTESIAN_POINT('Ctrl Pts',(-39.6504422346313,-33.8239773747795,
2.66900216498831));
#31689=CARTESIAN_POINT('Ctrl Pts',(-36.5844983552314,-30.4724170292356,
2.51200203763606));
#31690=CARTESIAN_POINT('Ctrl Pts',(-32.0977199449364,-31.1807841743797,
2.3550019102838));
#31691=CARTESIAN_POINT('Ctrl Pts',(-30.2134432077683,-35.3138779741053,
2.19800178293155));
#31692=CARTESIAN_POINT('Ctrl Pts',(-32.621319267345,-39.1655160273689,2.04100165557929));
#31693=CARTESIAN_POINT('Ctrl Pts',(-37.1621783376115,-39.2818925846584,
1.88400152822705));
#31694=CARTESIAN_POINT('Ctrl Pts',(-39.7641970350665,-35.558661654829,1.72700140087479));
#31695=CARTESIAN_POINT('Ctrl Pts',(-38.0941030920961,-31.3344600185395,
1.57000127352254));
#31696=CARTESIAN_POINT('Ctrl Pts',(-33.6495202958365,-30.3972103260493,
1.41300114617028));
#31697=CARTESIAN_POINT('Ctrl Pts',(-30.4158791260905,-33.5872717453,1.25600101881803));
#31698=CARTESIAN_POINT('Ctrl Pts',(-31.2929567559004,-38.0442500262742,
1.09900089146578));
#31699=CARTESIAN_POINT('Ctrl Pts',(-35.4939870016774,-39.7711987453336,
0.942000764113521));
#31700=CARTESIAN_POINT('Ctrl Pts',(-39.2524343486202,-37.2202137070602,
0.785000636761268));
#31701=CARTESIAN_POINT('Ctrl Pts',(-39.1969175216432,-32.6774433254408,
0.628000509409014));
#31702=CARTESIAN_POINT('Ctrl Pts',(-35.3795268907121,-30.2191428513895,
0.471000382056761));
#31703=CARTESIAN_POINT('Ctrl Pts',(-31.2186995847689,-32.0442153857854,
0.314000254704507));
#31704=CARTESIAN_POINT('Ctrl Pts',(-30.4549379250093,-36.5273603729133,
0.157000127352253));
#31705=CARTESIAN_POINT('Ctrl Pts',(-32.6539236935135,-38.5893527455387,
0.0523333757840845));
#31706=CARTESIAN_POINT('Ctrl Pts',(-33.9479286229388,-38.9352951690526,
0.));
#31707=CARTESIAN_POINT('Ctrl Pts',(-33.9479286229388,-38.9352951690526,
5.55111512312578E-17));
#31708=CARTESIAN_POINT('Ctrl Pts',(-33.8318206360164,-38.8956805466085,
1.21569200333733E-16));
#31709=CARTESIAN_POINT('Ctrl Pts',(-33.7179777099102,-38.8505155072641,
1.50554103324791E-15));
#31710=CARTESIAN_POINT('Ctrl Pts',(-33.6066257375518,-38.8001576608968,
1.0547118733939E-15));
#31711=CARTESIAN_POINT('Ctrl Pts',(-33.492776560763,-38.7486704781164,5.93772317186044E-16));
#31712=CARTESIAN_POINT('Ctrl Pts',(-33.3815306925957,-38.6917544682482,
3.73522748729697E-15));
#31713=CARTESIAN_POINT('Ctrl Pts',(-33.2731538396993,-38.6297432688828,
2.72004641033163E-15));
#31714=CARTESIAN_POINT('Ctrl Pts',(-33.1592154520342,-38.5645498637963,
1.65276966251693E-15));
#31715=CARTESIAN_POINT('Ctrl Pts',(-33.048447119632,-38.4937244909346,-6.09647221355942E-16));
#31716=CARTESIAN_POINT('Ctrl Pts',(-32.9411967497889,-38.4176086362753,
-1.0547118733939E-15));
#31717=CARTESIAN_POINT('Ctrl Pts',(-32.8473526761762,-38.3510072634485,
-1.44414344392711E-15));
#31718=CARTESIAN_POINT('Ctrl Pts',(-32.7562023471369,-38.2803543077884,
-2.56653707031024E-15));
#31719=CARTESIAN_POINT('Ctrl Pts',(-32.6680103311015,-38.2058563963449,
-2.83106871279415E-15));
#31720=CARTESIAN_POINT('Ctrl Pts',(-32.6506345001076,-38.1911786151031,
-2.88318745685931E-15));
#31721=CARTESIAN_POINT('Ctrl Pts',(-32.6333736067294,-38.1763515287969,
-1.26352082166837E-15));
#31722=CARTESIAN_POINT('Ctrl Pts',(-32.6162298289787,-38.1613766467586,
-1.22124532708767E-15));
#31723=CARTESIAN_POINT('Ctrl Pts',(-32.6036955222168,-38.1504280817505,
-1.1903365025982E-15));
#31724=CARTESIAN_POINT('Ctrl Pts',(-32.5912250315541,-38.1394015059403,
9.6075348530294E-17));
#31725=CARTESIAN_POINT('Ctrl Pts',(-32.5788280068545,-38.1283056318751,
1.11022302462516E-16));
#31726=CARTESIAN_POINT('Ctrl Pts',(-32.4862488011484,-38.0454432328352,
2.22644014631185E-16));
#31727=CARTESIAN_POINT('Ctrl Pts',(-32.3976254460622,-37.9585991267844,
2.93313669984113E-16));
#31728=CARTESIAN_POINT('Ctrl Pts',(-32.3132193670584,-37.8680942341505,
1.66533453693773E-16));
#31729=CARTESIAN_POINT('Ctrl Pts',(-32.2290050385629,-37.7777949470768,
4.00412518592805E-17));
#31730=CARTESIAN_POINT('Ctrl Pts',(-32.1489883292395,-37.6838507826712,
-7.67367206503618E-16));
#31731=CARTESIAN_POINT('Ctrl Pts',(-32.0734693158047,-37.5865484422576,
-3.88578058618805E-16));
#31732=CARTESIAN_POINT('Ctrl Pts',(-31.9989826203281,-37.4905761901068,
-1.49668231824771E-17));
#31733=CARTESIAN_POINT('Ctrl Pts',(-31.9288710981801,-37.3913362593944,
6.39667558614738E-17));
#31734=CARTESIAN_POINT('Ctrl Pts',(-31.8634687260135,-37.2890829263301,
2.77555756156289E-16));
#31735=CARTESIAN_POINT('Ctrl Pts',(-31.8101631638829,-37.2057423498624,
4.51639376496992E-16));
#31736=CARTESIAN_POINT('Ctrl Pts',(-31.7599865782998,-37.1203994732574,
-1.91642689345195E-15));
#31737=CARTESIAN_POINT('Ctrl Pts',(-31.7131457346326,-37.0331861281649,
-2.08166817117217E-15));
#31738=CARTESIAN_POINT('Ctrl Pts',(-31.7012454402134,-37.0110288738836,
-2.12364905155618E-15));
#31739=CARTESIAN_POINT('Ctrl Pts',(-31.6895605787933,-36.988750873417,8.89729854294519E-16));
#31740=CARTESIAN_POINT('Ctrl Pts',(-31.6780948040882,-36.9663542633258,
9.71445146547012E-16));
#31741=CARTESIAN_POINT('Ctrl Pts',(-31.6699383315321,-36.9504218610016,
1.0295754129979E-15));
#31742=CARTESIAN_POINT('Ctrl Pts',(-31.661896440285,-36.9344366167593,-7.00903233658188E-16));
#31743=CARTESIAN_POINT('Ctrl Pts',(-31.6539727955662,-36.9184049530428,
-6.38378239159465E-16));
#31744=CARTESIAN_POINT('Ctrl Pts',(-31.6010119288307,-36.8112508799156,
-2.20467287978913E-16));
#31745=CARTESIAN_POINT('Ctrl Pts',(-31.5532899127003,-36.7019469405238,
-5.43579179869397E-17));
#31746=CARTESIAN_POINT('Ctrl Pts',(-31.5110855463215,-36.5907557494425,
2.77555756156289E-17));
#31747=CARTESIAN_POINT('Ctrl Pts',(-31.4697173372396,-36.4817674898051,
1.08242228141372E-16));
#31748=CARTESIAN_POINT('Ctrl Pts',(-31.433650039522,-36.3709653855926,-1.8533573671039E-16));
#31749=CARTESIAN_POINT('Ctrl Pts',(-31.4031944204139,-36.2585829650152,
-1.08246744900953E-15));
#31750=CARTESIAN_POINT('Ctrl Pts',(-31.3987402034729,-36.2421467310371,
-1.21367539645156E-15));
#31751=CARTESIAN_POINT('Ctrl Pts',(-31.3944061093602,-36.2256766793315,
1.54092145767103E-16));
#31752=CARTESIAN_POINT('Ctrl Pts',(-31.3901932043347,-36.2091735273543,
1.66533453693773E-16));
#31753=CARTESIAN_POINT('Ctrl Pts',(-31.3605246504064,-36.0929533297801,
3.08986100652746E-16));
#31754=CARTESIAN_POINT('Ctrl Pts',(-31.3368620771271,-35.9750912152647,
2.82593330474131E-15));
#31755=CARTESIAN_POINT('Ctrl Pts',(-31.319114629565,-35.8560230245863,3.49720252756924E-15));
#31756=CARTESIAN_POINT('Ctrl Pts',(-31.3091310875555,-35.7890431234222,
3.87481426369542E-15));
#31757=CARTESIAN_POINT('Ctrl Pts',(-31.3010203073581,-35.7216816160001,
-1.45794491220195E-16));
#31758=CARTESIAN_POINT('Ctrl Pts',(-31.294773164211,-35.6540175415704,-4.71844785465692E-16));
#31759=CARTESIAN_POINT('Ctrl Pts',(-31.2918906865937,-35.6227968418935,
-6.22286780009977E-16));
#31760=CARTESIAN_POINT('Ctrl Pts',(-31.2894050399855,-35.5915117486406,
3.58433295205778E-16));
#31761=CARTESIAN_POINT('Ctrl Pts',(-31.2873156755218,-35.5601701609149,
2.4980018054066E-16));
#31762=CARTESIAN_POINT('Ctrl Pts',(-31.286114583885,-35.5421531420771,1.87351370019253E-16));
#31763=CARTESIAN_POINT('Ctrl Pts',(-31.2850449634327,-35.5241245074566,
-4.29409397736477E-17));
#31764=CARTESIAN_POINT('Ctrl Pts',(-31.284106744896,-35.5060940976467,-5.55111512312578E-17));
#31765=CARTESIAN_POINT('Ctrl Pts',(-31.2777958135452,-35.3848124622,-1.40064737065375E-16));
#31766=CARTESIAN_POINT('Ctrl Pts',(-31.2774174094918,-35.2633335332142,
2.82866543587948E-15));
#31767=CARTESIAN_POINT('Ctrl Pts',(-31.282813324883,-35.142104562563,2.35922392732846E-15));
#31768=CARTESIAN_POINT('Ctrl Pts',(-31.2880973068045,-35.0233903791791,
1.89952056570822E-15));
#31769=CARTESIAN_POINT('Ctrl Pts',(-31.2989190268708,-34.9049149676345,
7.28996419448176E-16));
#31770=CARTESIAN_POINT('Ctrl Pts',(-31.3151832922329,-34.7871043083849,
6.93889390390723E-16));
#31771=CARTESIAN_POINT('Ctrl Pts',(-31.3312886503615,-34.670444698108,6.59125368578839E-16));
#31772=CARTESIAN_POINT('Ctrl Pts',(-31.3527310724264,-34.5544360772762,
1.70606179182567E-15));
#31773=CARTESIAN_POINT('Ctrl Pts',(-31.379464911652,-34.4395109622456,2.28983498828939E-15));
#31774=CARTESIAN_POINT('Ctrl Pts',(-31.3968718099089,-34.3646810896034,
2.66994053729605E-15));
#31775=CARTESIAN_POINT('Ctrl Pts',(-31.4165229694089,-34.2903109886468,
-2.96848706176688E-17));
#31776=CARTESIAN_POINT('Ctrl Pts',(-31.4384155905674,-34.2165269562934,
1.38777878078145E-17));
#31777=CARTESIAN_POINT('Ctrl Pts',(-31.4458039406444,-34.1916262257156,
2.85793700622958E-17));
#31778=CARTESIAN_POINT('Ctrl Pts',(-31.4534476413064,-34.1667922990885,
3.06223347651583E-15));
#31779=CARTESIAN_POINT('Ctrl Pts',(-31.4613467725894,-34.1420302077573,
3.1641356201817E-15));
#31780=CARTESIAN_POINT('Ctrl Pts',(-31.4664331829338,-34.1260853964884,
3.22975247083094E-15));
#31781=CARTESIAN_POINT('Ctrl Pts',(-31.4716247119601,-34.1101729821539,
1.52985938675526E-15));
#31782=CARTESIAN_POINT('Ctrl Pts',(-31.4769185004878,-34.0943023310132,
1.56819002228303E-15));
#31783=CARTESIAN_POINT('Ctrl Pts',(-31.5138161753674,-33.9836839859762,
1.8353543263008E-15));
#31784=CARTESIAN_POINT('Ctrl Pts',(-31.5557145621555,-33.8749771180903,
2.68190903327311E-15));
#31785=CARTESIAN_POINT('Ctrl Pts',(-31.60254886788,-33.7686009256992,2.26207941267376E-15));
#31786=CARTESIAN_POINT('Ctrl Pts',(-31.6406629427424,-33.6820312606289,
1.92041922701669E-15));
#31787=CARTESIAN_POINT('Ctrl Pts',(-31.6820469232643,-33.5970053442715,
1.26636124083292E-15));
#31788=CARTESIAN_POINT('Ctrl Pts',(-31.7266868713332,-33.5137647678308,
1.40165656858926E-15));
#31789=CARTESIAN_POINT('Ctrl Pts',(-31.7483018585373,-33.473459075901,1.46716754933025E-15));
#31790=CARTESIAN_POINT('Ctrl Pts',(-31.7706804998245,-33.4335722114158,
1.17298588323861E-16));
#31791=CARTESIAN_POINT('Ctrl Pts',(-31.7938226860146,-33.3941331271239,
-4.02455846426619E-16));
#31792=CARTESIAN_POINT('Ctrl Pts',(-31.8074090785167,-33.3709790968731,
-7.07595028060502E-16));
#31793=CARTESIAN_POINT('Ctrl Pts',(-31.8212607024029,-33.3479763354121,
-4.73580047421181E-16));
#31794=CARTESIAN_POINT('Ctrl Pts',(-31.8353634826968,-33.3251531939272,
-3.88578058618805E-16));
#31795=CARTESIAN_POINT('Ctrl Pts',(-31.8937949297824,-33.2305910468749,
-3.63929499130585E-17));
#31796=CARTESIAN_POINT('Ctrl Pts',(-31.9565776402818,-33.1390341079118,
1.65098064735663E-15));
#31797=CARTESIAN_POINT('Ctrl Pts',(-32.0236775684477,-33.0508730884183,
2.24126273096203E-15));
#31798=CARTESIAN_POINT('Ctrl Pts',(-32.0837083254303,-32.9720000868933,
2.76935689262062E-15));
#31799=CARTESIAN_POINT('Ctrl Pts',(-32.1471951806296,-32.895845207831,1.97196154581884E-15));
#31800=CARTESIAN_POINT('Ctrl Pts',(-32.2141372439519,-32.8227147610826,
2.21437451708439E-15));
#31801=CARTESIAN_POINT('Ctrl Pts',(-32.2489921734814,-32.7846377069649,
2.36892565463969E-15));
#31802=CARTESIAN_POINT('Ctrl Pts',(-32.2847842063358,-32.7473810647789,
1.32299506859179E-17));
#31803=CARTESIAN_POINT('Ctrl Pts',(-32.3214759334524,-32.7109602322923,
-5.55111512312578E-17));
#31804=CARTESIAN_POINT('Ctrl Pts',(-38.5163032009778,-35.0029832534533,
6.38741669750803));
#31805=CARTESIAN_POINT('Ctrl Pts',(-38.5189473067417,-35.316893543218,6.40161070716451));
#31806=CARTESIAN_POINT('Ctrl Pts',(-38.4802906988737,-35.6301637893069,
6.41580471682099));
#31807=CARTESIAN_POINT('Ctrl Pts',(-38.3977162601254,-35.9313946627094,
6.42999872647747));
#31808=CARTESIAN_POINT('Ctrl Pts',(-38.0932639427213,-37.0420342125665,
6.48233210226156));
#31809=CARTESIAN_POINT('Ctrl Pts',(-37.1917925750707,-37.9890105144279,
6.53466547804564));
#31810=CARTESIAN_POINT('Ctrl Pts',(-36.0974795738098,-38.3477575516811,
6.58699885382972));
#31811=CARTESIAN_POINT('Ctrl Pts',(-35.0031665725488,-38.7065045889344,
6.63933222961381));
#31812=CARTESIAN_POINT('Ctrl Pts',(-33.7160119376775,-38.4770223615795,
6.69166560539789));
#31813=CARTESIAN_POINT('Ctrl Pts',(-32.8131208374828,-37.7621694030232,
6.74399898118198));
#31814=CARTESIAN_POINT('Ctrl Pts',(-31.9102297372881,-37.0473164444669,
6.79633235696606));
#31815=CARTESIAN_POINT('Ctrl Pts',(-31.3916021717699,-35.8470927547091,
6.84866573275014));
#31816=CARTESIAN_POINT('Ctrl Pts',(-31.4897608240433,-34.6996866784948,
6.90099910853423));
#31817=CARTESIAN_POINT('Ctrl Pts',(-31.5879194763167,-33.5522806022806,
6.95333248431831));
#31818=CARTESIAN_POINT('Ctrl Pts',(-32.3028643463816,-32.4576921396098,
7.0056658601024));
#31819=CARTESIAN_POINT('Ctrl Pts',(-33.3140595130386,-31.9065597820401,
7.05799923588649));
#31820=CARTESIAN_POINT('Ctrl Pts',(-34.3252546796956,-31.3554274244703,
7.11033261167057));
#31821=CARTESIAN_POINT('Ctrl Pts',(-35.6327001429448,-31.3477511720016,
7.16266598745465));
#31822=CARTESIAN_POINT('Ctrl Pts',(-36.6501701924127,-31.8872255334987,
7.21499936323874));
#31823=CARTESIAN_POINT('Ctrl Pts',(-37.6676402418807,-32.4266998949958,
7.26733273902282));
#31824=CARTESIAN_POINT('Ctrl Pts',(-38.3951348775673,-33.5133248704587,
7.3196661148069));
#31825=CARTESIAN_POINT('Ctrl Pts',(-38.5065312349523,-34.6593974459546,
7.37199949059099));
#31826=CARTESIAN_POINT('Ctrl Pts',(-38.5174702113759,-34.7719402721061,
7.37713855956333));
#31827=CARTESIAN_POINT('Ctrl Pts',(-38.5224681626868,-34.8850563504433,
7.38227762853568));
#31828=CARTESIAN_POINT('Ctrl Pts',(-38.5217392653161,-34.9982348400382,
7.38741669750802));
#31829=CARTESIAN_POINT('Ctrl Pts',(-36.0520713770612,-38.9352951690526,
8.));
#31830=CARTESIAN_POINT('Ctrl Pts',(-37.3460763064865,-38.5893527455387,
7.94766662421592));
#31831=CARTESIAN_POINT('Ctrl Pts',(-39.5450618542894,-36.527358944407,7.84299987264775));
#31832=CARTESIAN_POINT('Ctrl Pts',(-38.7813006061664,-32.0442159203332,
7.6859997452955));
#31833=CARTESIAN_POINT('Ctrl Pts',(-34.6204730922247,-30.2191423808613,
7.52899961794324));
#31834=CARTESIAN_POINT('Ctrl Pts',(-30.8030823517117,-32.6774434597138,
7.37199949059099));
#31835=CARTESIAN_POINT('Ctrl Pts',(-30.7475655592404,-37.2202136561835,
7.21499936323873));
#31836=CARTESIAN_POINT('Ctrl Pts',(-34.5060129709306,-39.7711989299046,
7.05799923588648));
#31837=CARTESIAN_POINT('Ctrl Pts',(-38.7070433506006,-38.044250072918,6.90099910853423));
#31838=CARTESIAN_POINT('Ctrl Pts',(-39.584120987438,-33.5872717262032,6.74399898118198));
#31839=CARTESIAN_POINT('Ctrl Pts',(-36.3504797430715,-30.3972101963624,
6.58699885382972));
#31840=CARTESIAN_POINT('Ctrl Pts',(-31.905896825022,-31.3344599279876,6.42999872647746));
#31841=CARTESIAN_POINT('Ctrl Pts',(-30.2358028418083,-35.5586616666892,
6.27299859912522));
#31842=CARTESIAN_POINT('Ctrl Pts',(-32.83782160528,-39.2818926978495,6.11599847177295));
#31843=CARTESIAN_POINT('Ctrl Pts',(-37.3786807951101,-39.1655161353224,
5.95899834442071));
#31844=CARTESIAN_POINT('Ctrl Pts',(-39.7865569169479,-35.3138779826965,
5.80199821706845));
#31845=CARTESIAN_POINT('Ctrl Pts',(-37.9022801309199,-31.1807840744948,
5.64499808971621));
#31846=CARTESIAN_POINT('Ctrl Pts',(-33.4155016033557,-30.4724169111822,
5.48799796236394));
#31847=CARTESIAN_POINT('Ctrl Pts',(-30.3495576440316,-33.8239773440302,
5.3309978350117));
#31848=CARTESIAN_POINT('Ctrl Pts',(-31.4537101308888,-38.230088373826,5.17399770765944));
#31849=CARTESIAN_POINT('Ctrl Pts',(-35.7378546799324,-39.7397482704758,
5.01699758030718));
#31850=CARTESIAN_POINT('Ctrl Pts',(-39.3603579010204,-36.9992303723996,
4.85999745295493));
#31851=CARTESIAN_POINT('Ctrl Pts',(-39.0728863399384,-32.4659834442205,
4.70299732560268));
#31852=CARTESIAN_POINT('Ctrl Pts',(-35.1332185347277,-30.2050134596587,
4.54599719825043));
#31853=CARTESIAN_POINT('Ctrl Pts',(-31.0740923862265,-32.2437539129077,
4.38899707089817));
#31854=CARTESIAN_POINT('Ctrl Pts',(-30.535365261007,-36.7540466716456,4.23199694354592));
#31855=CARTESIAN_POINT('Ctrl Pts',(-34.0001189367432,-39.6914689539076,
4.07499681619366));
#31856=CARTESIAN_POINT('Ctrl Pts',(-38.3614755549453,-38.4220060164266,
3.91799668884141));
#31857=CARTESIAN_POINT('Ctrl Pts',(-39.7085647942032,-34.0839974553828,
3.76099656148916));
#31858=CARTESIAN_POINT('Ctrl Pts',(-36.8334388106793,-30.5673771631648,
3.6039964341369));
#31859=CARTESIAN_POINT('Ctrl Pts',(-32.3142506564274,-31.0255322944533,
3.44699630678465));
#31860=CARTESIAN_POINT('Ctrl Pts',(-30.2033997043049,-35.0476307446275,
3.28999617943239));
#31861=CARTESIAN_POINT('Ctrl Pts',(-32.3937062542216,-39.0270182530956,
3.13299605208014));
#31862=CARTESIAN_POINT('Ctrl Pts',(-36.9211014088136,-39.3953398526252,
2.97599592472789));
#31863=CARTESIAN_POINT('Ctrl Pts',(-39.7258265015647,-35.8223180552711,
2.81899579737564));
#31864=CARTESIAN_POINT('Ctrl Pts',(-38.2928576294957,-31.5119157366759,
2.66199567002338));
#31865=CARTESIAN_POINT('Ctrl Pts',(-33.9071517375455,-30.3293121048675,
2.50499554267113));
#31866=CARTESIAN_POINT('Ctrl Pts',(-30.5014133532831,-33.3349589868354,
2.34799541531887));
#31867=CARTESIAN_POINT('Ctrl Pts',(-31.12960079995,-37.8336643815683,2.19099528796663));
#31868=CARTESIAN_POINT('Ctrl Pts',(-35.2284122851668,-39.7913952114128,
2.03399516061437));
#31869=CARTESIAN_POINT('Ctrl Pts',(-39.1224043939168,-37.4526370543192,
1.87699503326212));
#31870=CARTESIAN_POINT('Ctrl Pts',(-39.3197967106052,-32.9145735741338,
1.71999490590986));
#31871=CARTESIAN_POINT('Ctrl Pts',(-35.6435863248602,-30.2465363019221,
1.56299477855761));
#31872=CARTESIAN_POINT('Ctrl Pts',(-31.3902650003177,-31.8409668168855,
1.40599465120536));
#31873=CARTESIAN_POINT('Ctrl Pts',(-30.3738295074692,-36.2681502477922,
1.2489945238531));
#31874=CARTESIAN_POINT('Ctrl Pts',(-33.5057217955833,-39.5581358207848,
1.09199439650085));
#31875=CARTESIAN_POINT('Ctrl Pts',(-37.977555101084,-38.7608685197788,0.934994269148597));
#31876=CARTESIAN_POINT('Ctrl Pts',(-39.7793712418172,-34.5910508068424,
0.777994141796343));
#31877=CARTESIAN_POINT('Ctrl Pts',(-37.2955094371433,-30.7882309135474,
0.620994014444089));
#31878=CARTESIAN_POINT('Ctrl Pts',(-32.7531816644513,-30.7615622313046,
0.463993887091836));
#31879=CARTESIAN_POINT('Ctrl Pts',(-30.2257195673566,-34.5367150123096,
0.306993759739581));
#31880=CARTESIAN_POINT('Ctrl Pts',(-31.9791549439529,-38.7249342807031,
0.149993632387329));
#31881=CARTESIAN_POINT('Ctrl Pts',(-36.441898406148,-39.5777530280863,-0.00700649496492615));
#31882=CARTESIAN_POINT('Ctrl Pts',(-39.6107538265857,-36.3158122035465,
-0.164006622317178));
#31883=CARTESIAN_POINT('Ctrl Pts',(-38.9665644295237,-33.3709224100119,
-0.268673373885348));
#31884=CARTESIAN_POINT('Ctrl Pts',(-38.0961285948024,-32.3528524834368,
-0.321006749669432));
#31885=CARTESIAN_POINT('Ctrl Pts',(-36.0042049488753,-38.756249785149,8.10700224988981));
#31886=CARTESIAN_POINT('Ctrl Pts',(-37.2393361218454,-38.4260468148059,
8.05466887410573));
#31887=CARTESIAN_POINT('Ctrl Pts',(-39.3382737203354,-36.457868205641,7.95000212253756));
#31888=CARTESIAN_POINT('Ctrl Pts',(-38.6092615621806,-32.178696174684,7.7930019951853));
#31889=CARTESIAN_POINT('Ctrl Pts',(-34.6377405494255,-30.4366585902015,
7.63600186783305));
#31890=CARTESIAN_POINT('Ctrl Pts',(-30.9940308572923,-32.7831135580239,
7.4790017404808));
#31891=CARTESIAN_POINT('Ctrl Pts',(-30.9410399300978,-37.119199884829,7.32200161312854));
#31892=CARTESIAN_POINT('Ctrl Pts',(-34.528488056906,-39.5541221650401,7.16500148577629));
#31893=CARTESIAN_POINT('Ctrl Pts',(-38.5383828127393,-37.9057448529564,
7.00800135842404));
#31894=CARTESIAN_POINT('Ctrl Pts',(-39.3755557676012,-33.6515470766578,
6.85100123107178));
#31895=CARTESIAN_POINT('Ctrl Pts',(-36.2890365339436,-30.6066247973054,
6.69400110371953));
#31896=CARTESIAN_POINT('Ctrl Pts',(-32.046670227525,-31.5012321778987,6.53700097636728));
#31897=CARTESIAN_POINT('Ctrl Pts',(-30.4525610448241,-35.5332440580251,
6.38000084901503));
#31898=CARTESIAN_POINT('Ctrl Pts',(-32.936194927768,-39.0870780552405,6.22300072166276));
#31899=CARTESIAN_POINT('Ctrl Pts',(-37.2704571936142,-38.975996314428,6.06600059431052));
#31900=CARTESIAN_POINT('Ctrl Pts',(-39.5687814048312,-35.2995973756527,
5.90900046695826));
#31901=CARTESIAN_POINT('Ctrl Pts',(-37.7702341628505,-31.3545481639004,
5.75200033960601));
#31902=CARTESIAN_POINT('Ctrl Pts',(-33.4875920340692,-30.678409808149,5.59500021225376));
#31903=CARTESIAN_POINT('Ctrl Pts',(-30.5611403084004,-33.8774832232266,
5.4380000849015));
#31904=CARTESIAN_POINT('Ctrl Pts',(-31.6150568161493,-38.0831280092054,
5.28099995754926));
#31905=CARTESIAN_POINT('Ctrl Pts',(-35.7042842693892,-39.5241024263299,
5.12399983019699));
#31906=CARTESIAN_POINT('Ctrl Pts',(-39.1619733019478,-36.908270748239,4.96699970284474));
#31907=CARTESIAN_POINT('Ctrl Pts',(-38.8875809264933,-32.581274406539,4.80999957549249));
#31908=CARTESIAN_POINT('Ctrl Pts',(-35.127157448413,-30.4231724970492,4.65299944814023));
#31909=CARTESIAN_POINT('Ctrl Pts',(-31.2527106615227,-32.3691557233429,
4.49599932078798));
#31910=CARTESIAN_POINT('Ctrl Pts',(-30.7384941767535,-36.6742422487958,
4.33899919343573));
#31911=CARTESIAN_POINT('Ctrl Pts',(-34.045610845517,-39.4780196892807,4.18199906608348));
#31912=CARTESIAN_POINT('Ctrl Pts',(-38.2085374256912,-38.2663139133921,
4.02499893873122));
#31913=CARTESIAN_POINT('Ctrl Pts',(-39.4943377146584,-34.1256731163465,
3.86799881137897));
#31914=CARTESIAN_POINT('Ctrl Pts',(-36.7500222582684,-30.7690496231526,
3.71099868402672));
#31915=CARTESIAN_POINT('Ctrl Pts',(-32.4364450539584,-31.206359923788,3.55399855667446));
#31916=CARTESIAN_POINT('Ctrl Pts',(-30.4216321632391,-35.0454636733936,
3.39699842932221));
#31917=CARTESIAN_POINT('Ctrl Pts',(-32.5122856349878,-38.843799714679,3.23999830196996));
#31918=CARTESIAN_POINT('Ctrl Pts',(-36.8336964431165,-39.1953636685035,
3.0829981746177));
#31919=CARTESIAN_POINT('Ctrl Pts',(-39.510814060595,-35.7849047875054,2.92599804726545));
#31920=CARTESIAN_POINT('Ctrl Pts',(-38.1430414319588,-31.6706142228596,
2.76899791991319));
#31921=CARTESIAN_POINT('Ctrl Pts',(-33.9568734047379,-30.5418158870118,
2.61199779256094));
#31922=CARTESIAN_POINT('Ctrl Pts',(-30.7060869898426,-33.4107138907526,
2.45499766520869));
#31923=CARTESIAN_POINT('Ctrl Pts',(-31.3056935911801,-37.7047402462095,
2.29799753785644));
#31924=CARTESIAN_POINT('Ctrl Pts',(-35.2180201383191,-39.5733995698641,
2.14099741050418));
#31925=CARTESIAN_POINT('Ctrl Pts',(-38.9348460417202,-37.3410486412263,
1.98399728315193));
#31926=CARTESIAN_POINT('Ctrl Pts',(-39.1232575369955,-33.0094548877283,
1.82699715579967));
#31927=CARTESIAN_POINT('Ctrl Pts',(-35.614304871841,-30.4628061612676,1.66999702844742));
#31928=CARTESIAN_POINT('Ctrl Pts',(-31.5544982689911,-31.9846943607513,
1.51299690109517));
#31929=CARTESIAN_POINT('Ctrl Pts',(-30.5843078670984,-36.2104528100627,
1.35599677374291));
#31930=CARTESIAN_POINT('Ctrl Pts',(-33.5737074493336,-39.3507528563925,
1.19899664639066));
#31931=CARTESIAN_POINT('Ctrl Pts',(-37.8420843236033,-38.5897590809672,
1.04199651903841));
#31932=CARTESIAN_POINT('Ctrl Pts',(-39.5619226586618,-34.6096568991787,
0.884996391686153));
#31933=CARTESIAN_POINT('Ctrl Pts',(-37.191069909542,-30.9798551197638,0.7279962643339));
#31934=CARTESIAN_POINT('Ctrl Pts',(-32.8554058774184,-30.954399791093,0.570996136981647));
#31935=CARTESIAN_POINT('Ctrl Pts',(-30.4429365323376,-34.5577932376814,
0.413996009629392));
#31936=CARTESIAN_POINT('Ctrl Pts',(-32.1165952983707,-38.5554597534685,
0.25699588227714));
#31937=CARTESIAN_POINT('Ctrl Pts',(-36.3762958928451,-39.3694775333344,
0.0999957549248847));
#31938=CARTESIAN_POINT('Ctrl Pts',(-39.4009768839417,-36.2559462745606,
-0.0570043724273669));
#31939=CARTESIAN_POINT('Ctrl Pts',(-38.7860963780679,-33.4450410745538,
-0.161671123995537));
#31940=CARTESIAN_POINT('Ctrl Pts',(-37.9552630411254,-32.4732906012887,
-0.214004499779622));
#31941=CARTESIAN_POINT('Ctrl Pts',(-35.9563385206894,-38.5772044012455,
8.21400449977962));
#31942=CARTESIAN_POINT('Ctrl Pts',(-37.1325959372043,-38.2627408840732,
8.16167112399554));
#31943=CARTESIAN_POINT('Ctrl Pts',(-39.1314855863814,-36.388377466875,8.05700437242737));
#31944=CARTESIAN_POINT('Ctrl Pts',(-38.4372225181948,-32.3131764290349,
7.90000424507512));
#31945=CARTESIAN_POINT('Ctrl Pts',(-34.6550080066264,-30.6541747995416,
7.74300411772286));
#31946=CARTESIAN_POINT('Ctrl Pts',(-31.184979362873,-32.8887836563341,7.58600399037061));
#31947=CARTESIAN_POINT('Ctrl Pts',(-31.1345143009551,-37.0181861134745,
7.42900386301835));
#31948=CARTESIAN_POINT('Ctrl Pts',(-34.5509631428814,-39.3370454001755,
7.2720037356661));
#31949=CARTESIAN_POINT('Ctrl Pts',(-38.3697222748781,-37.7672396329946,
7.11500360831385));
#31950=CARTESIAN_POINT('Ctrl Pts',(-39.1669905477644,-33.7158224271125,
6.95800348096159));
#31951=CARTESIAN_POINT('Ctrl Pts',(-36.2275933248156,-30.8160393982482,
6.80100335360935));
#31952=CARTESIAN_POINT('Ctrl Pts',(-32.187443630028,-31.6680044278098,6.64400322625708));
#31953=CARTESIAN_POINT('Ctrl Pts',(-30.6693192478399,-35.5078264493611,
6.48700309890484));
#31954=CARTESIAN_POINT('Ctrl Pts',(-33.0345682502559,-38.8922634126314,
6.33000297155257));
#31955=CARTESIAN_POINT('Ctrl Pts',(-37.1622335921182,-38.7864764935337,
6.17300284420033));
#31956=CARTESIAN_POINT('Ctrl Pts',(-39.3510058927144,-35.2853167686088,
6.01600271684807));
#31957=CARTESIAN_POINT('Ctrl Pts',(-37.6381881947812,-31.5283122533059,
5.85900258949583));
#31958=CARTESIAN_POINT('Ctrl Pts',(-33.5596824647827,-30.8844027051158,
5.70200246214357));
#31959=CARTESIAN_POINT('Ctrl Pts',(-30.7727229727691,-33.9309891024229,
5.54500233479131));
#31960=CARTESIAN_POINT('Ctrl Pts',(-31.7764035014098,-37.9361676445846,
5.38800220743907));
#31961=CARTESIAN_POINT('Ctrl Pts',(-35.6707138588461,-39.3084565821841,
5.2310020800868));
#31962=CARTESIAN_POINT('Ctrl Pts',(-38.9635887028751,-36.8173111240784,
5.07400195273455));
#31963=CARTESIAN_POINT('Ctrl Pts',(-38.7022755130482,-32.6965653688576,
4.9170018253823));
#31964=CARTESIAN_POINT('Ctrl Pts',(-35.1210963620983,-30.6413315344396,
4.76000169803004));
#31965=CARTESIAN_POINT('Ctrl Pts',(-31.431328936819,-32.4945575337781,4.6030015706778));
#31966=CARTESIAN_POINT('Ctrl Pts',(-30.9416230925,-36.5944378259461,4.44600144332554));
#31967=CARTESIAN_POINT('Ctrl Pts',(-34.0911027542909,-39.2645704246538,
4.28900131597328));
#31968=CARTESIAN_POINT('Ctrl Pts',(-38.0555992964371,-38.1106218103576,
4.13200118862104));
#31969=CARTESIAN_POINT('Ctrl Pts',(-39.2801106351136,-34.1673487773102,
3.97500106126878));
#31970=CARTESIAN_POINT('Ctrl Pts',(-36.6666057058575,-30.9707220831404,
3.81800093391653));
#31971=CARTESIAN_POINT('Ctrl Pts',(-32.5586394514893,-31.3871875531226,
3.66100080656427));
#31972=CARTESIAN_POINT('Ctrl Pts',(-30.6398646221734,-35.0432966021599,
3.50400067921202));
#31973=CARTESIAN_POINT('Ctrl Pts',(-32.6308650157539,-38.6605811762622,
3.34700055185977));
#31974=CARTESIAN_POINT('Ctrl Pts',(-36.7462914774195,-38.9953874843817,
3.19000042450751));
#31975=CARTESIAN_POINT('Ctrl Pts',(-39.2958016196254,-35.7474915197397,
3.03300029715526));
#31976=CARTESIAN_POINT('Ctrl Pts',(-37.9932252344219,-31.8293127090433,
2.876000169803));
#31977=CARTESIAN_POINT('Ctrl Pts',(-34.0065950719303,-30.754319669156,2.71900004245075));
#31978=CARTESIAN_POINT('Ctrl Pts',(-30.910760626402,-33.4864687946697,2.5619999150985));
#31979=CARTESIAN_POINT('Ctrl Pts',(-31.4817863824102,-37.5758161108508,
2.40499978774625));
#31980=CARTESIAN_POINT('Ctrl Pts',(-35.2076279914714,-39.3554039283154,
2.24799966039399));
#31981=CARTESIAN_POINT('Ctrl Pts',(-38.7472876895237,-37.2294602281335,
2.09099953304174));
#31982=CARTESIAN_POINT('Ctrl Pts',(-38.9267183633859,-33.1043362013228,
1.93399940568948));
#31983=CARTESIAN_POINT('Ctrl Pts',(-35.5850234188216,-30.6790760206131,
1.77699927833723));
#31984=CARTESIAN_POINT('Ctrl Pts',(-31.7187315376645,-32.128421904617,1.61999915098498));
#31985=CARTESIAN_POINT('Ctrl Pts',(-30.7947862267274,-36.1527553723333,
1.46299902363272));
#31986=CARTESIAN_POINT('Ctrl Pts',(-33.6416931030839,-39.1433698920001,
1.30599889628047));
#31987=CARTESIAN_POINT('Ctrl Pts',(-37.7066135461226,-38.4186496421557,
1.14899876892822));
#31988=CARTESIAN_POINT('Ctrl Pts',(-39.3444740755065,-34.628262991515,0.991998641575964));
#31989=CARTESIAN_POINT('Ctrl Pts',(-37.0866303819407,-31.1714793259802,
0.83499851422371));
#31990=CARTESIAN_POINT('Ctrl Pts',(-32.9576300903856,-31.1472373508815,
0.677998386871457));
#31991=CARTESIAN_POINT('Ctrl Pts',(-30.6601534973185,-34.5788714630532,
0.520998259519203));
#31992=CARTESIAN_POINT('Ctrl Pts',(-32.2540356527884,-38.3859852262338,
0.363998132166951));
#31993=CARTESIAN_POINT('Ctrl Pts',(-36.3106933795422,-39.1612020385825,
0.206998004814695));
#31994=CARTESIAN_POINT('Ctrl Pts',(-39.1911999412976,-36.1960803455747,
0.049997877462444));
#31995=CARTESIAN_POINT('Ctrl Pts',(-38.6056283266121,-33.5191597390956,
-0.0546688741057268));
#31996=CARTESIAN_POINT('Ctrl Pts',(-37.8143974874483,-32.5937287191406,
-0.107002249889811));
#31997=CARTESIAN_POINT('Ctrl Pts',(-35.9084720925035,-38.3981590173419,
8.32100674966943));
#31998=CARTESIAN_POINT('Ctrl Pts',(-37.0258557525633,-38.0994349533404,
8.26867337388535));
#31999=CARTESIAN_POINT('Ctrl Pts',(-38.9246974524274,-36.318886728109,8.16400662231718));
#32000=CARTESIAN_POINT('Ctrl Pts',(-38.265183474209,-32.4476566833857,8.00700649496493));
#32001=CARTESIAN_POINT('Ctrl Pts',(-34.6722754638272,-30.8716910088818,
7.85000636761267));
#32002=CARTESIAN_POINT('Ctrl Pts',(-31.3759278684536,-32.9944537546442,
7.69300624026043));
#32003=CARTESIAN_POINT('Ctrl Pts',(-31.3279886718125,-36.9171723421199,
7.53600611290816));
#32004=CARTESIAN_POINT('Ctrl Pts',(-34.5734382288568,-39.119968635311,7.37900598555592));
#32005=CARTESIAN_POINT('Ctrl Pts',(-38.2010617370167,-37.6287344130329,
7.22200585820366));
#32006=CARTESIAN_POINT('Ctrl Pts',(-38.9584253279276,-33.7800977775671,
7.0650057308514));
#32007=CARTESIAN_POINT('Ctrl Pts',(-36.1661501156877,-31.0254539991911,
6.90800560349916));
#32008=CARTESIAN_POINT('Ctrl Pts',(-32.328217032531,-31.834776677721,6.75100547614689));
#32009=CARTESIAN_POINT('Ctrl Pts',(-30.8860774508557,-35.482408840697,6.59400534879465));
#32010=CARTESIAN_POINT('Ctrl Pts',(-33.1329415727439,-38.6974487700223,
6.43700522144238));
#32011=CARTESIAN_POINT('Ctrl Pts',(-37.0540099906223,-38.5969566726394,
6.28000509409015));
#32012=CARTESIAN_POINT('Ctrl Pts',(-39.1332303805976,-35.271036161565,6.12300496673788));
#32013=CARTESIAN_POINT('Ctrl Pts',(-37.5061422267118,-31.7020763427115,
5.96600483938563));
#32014=CARTESIAN_POINT('Ctrl Pts',(-33.6317728954962,-31.0903956020826,
5.80900471203338));
#32015=CARTESIAN_POINT('Ctrl Pts',(-30.9843056371378,-33.9844949816193,
5.65200458468112));
#32016=CARTESIAN_POINT('Ctrl Pts',(-31.9377501866703,-37.7892072799639,
5.49500445732888));
#32017=CARTESIAN_POINT('Ctrl Pts',(-35.6371434483029,-39.0928107380382,
5.33800432997661));
#32018=CARTESIAN_POINT('Ctrl Pts',(-38.7652041038025,-36.7263514999179,
5.18100420262437));
#32019=CARTESIAN_POINT('Ctrl Pts',(-38.5169700996031,-32.8118563311761,
5.02400407527211));
#32020=CARTESIAN_POINT('Ctrl Pts',(-35.1150352757837,-30.85949057183,4.86700394791986));
#32021=CARTESIAN_POINT('Ctrl Pts',(-31.6099472121153,-32.6199593442133,
4.7100038205676));
#32022=CARTESIAN_POINT('Ctrl Pts',(-31.1447520082465,-36.5146334030964,
4.55300369321535));
#32023=CARTESIAN_POINT('Ctrl Pts',(-34.1365946630648,-39.0511211600269,
4.3960035658631));
#32024=CARTESIAN_POINT('Ctrl Pts',(-37.902661167183,-37.9549297073231,4.23900343851084));
#32025=CARTESIAN_POINT('Ctrl Pts',(-39.0658835555688,-34.2090244382739,
4.08200331115859));
#32026=CARTESIAN_POINT('Ctrl Pts',(-36.5831891534466,-31.1723945431281,
3.92500318380633));
#32027=CARTESIAN_POINT('Ctrl Pts',(-32.6808338490201,-31.5680151824572,
3.76800305645409));
#32028=CARTESIAN_POINT('Ctrl Pts',(-30.8580970811077,-35.041129530926,3.61100292910183));
#32029=CARTESIAN_POINT('Ctrl Pts',(-32.74944439652,-38.4773626378456,3.45400280174958));
#32030=CARTESIAN_POINT('Ctrl Pts',(-36.6588865117225,-38.79541130026,3.29700267439732));
#32031=CARTESIAN_POINT('Ctrl Pts',(-39.0807891786557,-35.710078251974,3.14000254704507));
#32032=CARTESIAN_POINT('Ctrl Pts',(-37.8434090368849,-31.988011195227,2.98300241969281));
#32033=CARTESIAN_POINT('Ctrl Pts',(-34.0563167391228,-30.9668234513003,
2.82600229234056));
#32034=CARTESIAN_POINT('Ctrl Pts',(-31.1154342629614,-33.5622236985868,
2.66900216498831));
#32035=CARTESIAN_POINT('Ctrl Pts',(-31.6578791736403,-37.446891975492,2.51200203763606));
#32036=CARTESIAN_POINT('Ctrl Pts',(-35.1972358446236,-39.1374082867668,
2.3550019102838));
#32037=CARTESIAN_POINT('Ctrl Pts',(-38.5597293373271,-37.1178718150406,
2.19800178293155));
#32038=CARTESIAN_POINT('Ctrl Pts',(-38.7301791897763,-33.1992175149173,
2.04100165557929));
#32039=CARTESIAN_POINT('Ctrl Pts',(-35.5557419658023,-30.8953458799586,
1.88400152822704));
#32040=CARTESIAN_POINT('Ctrl Pts',(-31.8829648063379,-32.2721494484828,
1.72700140087479));
#32041=CARTESIAN_POINT('Ctrl Pts',(-31.0052645863564,-36.0950579346039,
1.57000127352254));
#32042=CARTESIAN_POINT('Ctrl Pts',(-33.7096787568343,-38.9359869276078,
1.41300114617028));
#32043=CARTESIAN_POINT('Ctrl Pts',(-37.5711427686419,-38.247540203344,1.25600101881803));
#32044=CARTESIAN_POINT('Ctrl Pts',(-39.1270254923511,-34.6468690838513,
1.09900089146578));
#32045=CARTESIAN_POINT('Ctrl Pts',(-36.9821908543394,-31.3631035321966,
0.94200076411352));
#32046=CARTESIAN_POINT('Ctrl Pts',(-33.0598543033527,-31.3400749106699,
0.785000636761268));
#32047=CARTESIAN_POINT('Ctrl Pts',(-30.8773704622995,-34.599949688425,0.628000509409013));
#32048=CARTESIAN_POINT('Ctrl Pts',(-32.3914760072062,-38.2165106989991,
0.471000382056762));
#32049=CARTESIAN_POINT('Ctrl Pts',(-36.2450908662393,-38.9529265438306,
0.314000254704506));
#32050=CARTESIAN_POINT('Ctrl Pts',(-38.9814229986536,-36.1362144165888,
0.157000127352255));
#32051=CARTESIAN_POINT('Ctrl Pts',(-38.4251602751564,-33.5932784036374,
0.0523333757840841));
#32052=CARTESIAN_POINT('Ctrl Pts',(-37.6735319337713,-32.7141668369925,
0.));
#32053=CARTESIAN_POINT('Ctrl Pts',(-37.6735319337713,-32.7141668369925,
0.));
#32054=CARTESIAN_POINT('Ctrl Pts',(-37.7506744675535,-32.7912795750214,
1.11409720010452E-16));
#32055=CARTESIAN_POINT('Ctrl Pts',(-37.8237046409441,-32.8720144826054,
2.54111086902063E-16));
#32056=CARTESIAN_POINT('Ctrl Pts',(-37.8926301480271,-32.9559530569886,
5.55111512312578E-17));
#32057=CARTESIAN_POINT('Ctrl Pts',(-37.9633155600031,-33.0420348714294,
-1.48159722809431E-16));
#32058=CARTESIAN_POINT('Ctrl Pts',(-38.0296843928246,-33.1314864952968,
-2.01877327443104E-15));
#32059=CARTESIAN_POINT('Ctrl Pts',(-38.0917150717573,-33.2239026806474,
-1.83186799063151E-15));
#32060=CARTESIAN_POINT('Ctrl Pts',(-38.155036796301,-33.318242325688,-1.64107264387499E-15));
#32061=CARTESIAN_POINT('Ctrl Pts',(-38.2138383235334,-33.4156718046105,
-8.85373385211783E-16));
#32062=CARTESIAN_POINT('Ctrl Pts',(-38.268059911681,-33.515799485594,-9.43689570931383E-16));
#32063=CARTESIAN_POINT('Ctrl Pts',(-38.319849146258,-33.6114354884346,-9.99389721462685E-16));
#32064=CARTESIAN_POINT('Ctrl Pts',(-38.3674601237765,-33.7095338759835,
-7.11957983305256E-16));
#32065=CARTESIAN_POINT('Ctrl Pts',(-38.4108052730721,-33.809777999414,-7.21644966006352E-16));
#32066=CARTESIAN_POINT('Ctrl Pts',(-38.4178427440334,-33.8260535254913,
-7.23217733907022E-16));
#32067=CARTESIAN_POINT('Ctrl Pts',(-38.4247676868796,-33.8423856539009,
2.30001299369943E-15));
#32068=CARTESIAN_POINT('Ctrl Pts',(-38.4315796332288,-33.8587730721181,
2.33146835171283E-15));
#32069=CARTESIAN_POINT('Ctrl Pts',(-38.4380896782009,-33.8744342097871,
2.3615296271221E-15));
#32070=CARTESIAN_POINT('Ctrl Pts',(-38.4444935030833,-33.8901386536763,
1.24943603957411E-15));
#32071=CARTESIAN_POINT('Ctrl Pts',(-38.4507888941826,-33.9058797515619,
1.16573417585641E-15));
#32072=CARTESIAN_POINT('Ctrl Pts',(-38.4941742238636,-34.0143611327099,
5.88894247237743E-16));
#32073=CARTESIAN_POINT('Ctrl Pts',(-38.5324456986686,-34.1246595013341,
-1.81750747552515E-15));
#32074=CARTESIAN_POINT('Ctrl Pts',(-38.5655747031801,-34.2363430523647,
-1.22124532708767E-15));
#32075=CARTESIAN_POINT('Ctrl Pts',(-38.5991382485882,-34.3494915152183,
-6.17162228628305E-16));
#32076=CARTESIAN_POINT('Ctrl Pts',(-38.6274239303319,-34.4640624881056,
-2.28097715513866E-15));
#32077=CARTESIAN_POINT('Ctrl Pts',(-38.6503593525615,-34.5796394751672,
-2.85882428840978E-15));
#32078=CARTESIAN_POINT('Ctrl Pts',(-38.6743343050071,-34.7004548994865,
-3.46286189462104E-15));
#32079=CARTESIAN_POINT('Ctrl Pts',(-38.6924637958468,-34.8223704157046,
7.50012201101083E-16));
#32080=CARTESIAN_POINT('Ctrl Pts',(-38.7046094044796,-34.9449336658503,
9.15933995315754E-16));
#32081=CARTESIAN_POINT('Ctrl Pts',(-38.7137186109542,-35.0368561034595,
1.04037534097676E-15));
#32082=CARTESIAN_POINT('Ctrl Pts',(-38.7194607604909,-35.1291434881023,
1.55226768069038E-15));
#32083=CARTESIAN_POINT('Ctrl Pts',(-38.7217543278029,-35.2216084347256,
1.52655665885959E-15));
#32084=CARTESIAN_POINT('Ctrl Pts',(-38.7223018974601,-35.2436836530358,
1.52041837142613E-15));
#32085=CARTESIAN_POINT('Ctrl Pts',(-38.7226527519925,-35.2657735186889,
2.89381252678048E-15));
#32086=CARTESIAN_POINT('Ctrl Pts',(-38.722805679631,-35.2878464184275,2.85882428840978E-15));
#32087=CARTESIAN_POINT('Ctrl Pts',(-38.7236405005601,-35.4083407832928,
2.66782602310891E-15));
#32088=CARTESIAN_POINT('Ctrl Pts',(-38.7185871650491,-35.5284803305467,
-1.0113839359997E-15));
#32089=CARTESIAN_POINT('Ctrl Pts',(-38.7075767134548,-35.6478390239293,
-6.10622663543836E-16));
#32090=CARTESIAN_POINT('Ctrl Pts',(-38.696636914708,-35.766431805807,-2.12433031749896E-16));
#32091=CARTESIAN_POINT('Ctrl Pts',(-38.6798164549903,-35.8842545994116,
4.47017550934916E-16));
#32092=CARTESIAN_POINT('Ctrl Pts',(-38.6569982586142,-36.0009023628565,
1.11022302462516E-15));
#32093=CARTESIAN_POINT('Ctrl Pts',(-38.6541246129484,-36.0155925835174,
1.19374485534308E-15));
#32094=CARTESIAN_POINT('Ctrl Pts',(-38.6511557754508,-36.0302641749016,
1.91345521755541E-15));
#32095=CARTESIAN_POINT('Ctrl Pts',(-38.6480914530901,-36.044916331709,1.97064586870965E-15));
#32096=CARTESIAN_POINT('Ctrl Pts',(-38.6241809707793,-36.1592450787926,
2.44399783547239E-15));
#32097=CARTESIAN_POINT('Ctrl Pts',(-38.594461283178,-36.2723911010901,-8.48644965904397E-16));
#32098=CARTESIAN_POINT('Ctrl Pts',(-38.5592385353076,-36.3840879064664,
-8.60422844084496E-16));
#32099=CARTESIAN_POINT('Ctrl Pts',(-38.5372732895732,-36.4537431130068,
-8.67767642662035E-16));
#32100=CARTESIAN_POINT('Ctrl Pts',(-38.5131668858195,-36.5228346461715,
9.22437028861002E-17));
#32101=CARTESIAN_POINT('Ctrl Pts',(-38.4869837165243,-36.5912956919754,
8.32667268468867E-17));
#32102=CARTESIAN_POINT('Ctrl Pts',(-38.4780341824549,-36.6146960089858,
8.01983529614736E-17));
#32103=CARTESIAN_POINT('Ctrl Pts',(-38.4688419572729,-36.6380226459113,
-1.61456985271483E-15));
#32104=CARTESIAN_POINT('Ctrl Pts',(-38.4594094252689,-36.6612728659742,
-1.77635683940025E-15));
#32105=CARTESIAN_POINT('Ctrl Pts',(-38.4526602969819,-36.6779087722017,
-1.89211802927477E-15));
#32106=CARTESIAN_POINT('Ctrl Pts',(-38.4457875924452,-36.6945066762169,
2.33562128204704E-15));
#32107=CARTESIAN_POINT('Ctrl Pts',(-38.4387992548886,-36.7110492733397,
2.24820162486594E-15));
#32108=CARTESIAN_POINT('Ctrl Pts',(-38.3928779298073,-36.8197529491441,
1.67375506108868E-15));
#32109=CARTESIAN_POINT('Ctrl Pts',(-38.341903576542,-36.9262302239648,1.3366443388947E-15));
#32110=CARTESIAN_POINT('Ctrl Pts',(-38.2862346344182,-37.0302267509451,
1.30451205393456E-15));
#32111=CARTESIAN_POINT('Ctrl Pts',(-38.2286504882323,-37.1378011179799,
1.2712743072873E-15));
#32112=CARTESIAN_POINT('Ctrl Pts',(-38.1660430056126,-37.2427217973211,
4.33181580130382E-15));
#32113=CARTESIAN_POINT('Ctrl Pts',(-38.098753525921,-37.3446999432836,3.3584246494911E-15));
#32114=CARTESIAN_POINT('Ctrl Pts',(-38.030830880622,-37.4476376605642,2.37587429771653E-15));
#32115=CARTESIAN_POINT('Ctrl Pts',(-37.9581372777995,-37.5475779522675,
-1.61807423508707E-16));
#32116=CARTESIAN_POINT('Ctrl Pts',(-37.8809732699071,-37.6442054678576,
-4.30211422042248E-16));
#32117=CARTESIAN_POINT('Ctrl Pts',(-37.826560213076,-37.7123434332233,-6.19479481397997E-16));
#32118=CARTESIAN_POINT('Ctrl Pts',(-37.769923167717,-37.7788337520814,-1.16007728999665E-15));
#32119=CARTESIAN_POINT('Ctrl Pts',(-37.7111544669349,-37.8435573649047,
-1.58206781009085E-15));
#32120=CARTESIAN_POINT('Ctrl Pts',(-37.6849217834628,-37.8724481524459,
-1.77043242585642E-15));
#32121=CARTESIAN_POINT('Ctrl Pts',(-37.6582642395734,-37.9009868195143,
-1.55320898075906E-15));
#32122=CARTESIAN_POINT('Ctrl Pts',(-37.6311894369306,-37.9291622039588,
-1.76247905159244E-15));
#32123=CARTESIAN_POINT('Ctrl Pts',(-37.6195672281553,-37.9412568516894,
-1.85231093276087E-15));
#32124=CARTESIAN_POINT('Ctrl Pts',(-37.6078695516101,-37.9532830190668,
-1.32384934798458E-15));
#32125=CARTESIAN_POINT('Ctrl Pts',(-37.5961035133295,-37.9652334405448,
-1.346145417358E-15));
#32126=CARTESIAN_POINT('Ctrl Pts',(-37.5076612499423,-38.0550616646887,
-1.51373919811968E-15));
#32127=CARTESIAN_POINT('Ctrl Pts',(-37.4152596553304,-38.1407172584711,
9.39449970766038E-16));
#32128=CARTESIAN_POINT('Ctrl Pts',(-37.3192274679083,-38.221882071393,-9.29811783123569E-16));
#32129=CARTESIAN_POINT('Ctrl Pts',(-37.2371876089162,-38.2912208002711,
-2.52671355975721E-15));
#32130=CARTESIAN_POINT('Ctrl Pts',(-37.1524970590086,-38.3572819982496,
-3.43309726072543E-16));
#32131=CARTESIAN_POINT('Ctrl Pts',(-37.0653365594432,-38.419849736978,-1.11022302462516E-16));
#32132=CARTESIAN_POINT('Ctrl Pts',(-37.0262256852631,-38.4479252869043,
-6.78971724635936E-18));
#32133=CARTESIAN_POINT('Ctrl Pts',(-36.9866172085179,-38.4752971710175,
-3.75915299087743E-16));
#32134=CARTESIAN_POINT('Ctrl Pts',(-36.9465262167991,-38.5019445229708,
-5.06539254985228E-16));
#32135=CARTESIAN_POINT('Ctrl Pts',(-36.9192926653871,-38.5200458968282,
-5.95271263500483E-16));
#32136=CARTESIAN_POINT('Ctrl Pts',(-36.8918308185162,-38.5378163160328,
-1.49578843933597E-15));
#32137=CARTESIAN_POINT('Ctrl Pts',(-36.8641753660581,-38.555230466303,-1.48492329543615E-15));
#32138=CARTESIAN_POINT('Ctrl Pts',(-36.7573710739483,-38.6224832438564,
-1.44296252821847E-15));
#32139=CARTESIAN_POINT('Ctrl Pts',(-36.6476200524945,-38.6844692154967,
-2.67652767243929E-15));
#32140=CARTESIAN_POINT('Ctrl Pts',(-36.5352242775472,-38.7408547238633,
-3.18495230189342E-15));
#32141=CARTESIAN_POINT('Ctrl Pts',(-36.4331305324386,-38.792072020258,-3.64677548475584E-15));
#32142=CARTESIAN_POINT('Ctrl Pts',(-36.3288538528326,-38.8386685011131,
8.48923205726707E-17));
#32143=CARTESIAN_POINT('Ctrl Pts',(-36.2225972039516,-38.8803649981066,
1.52308721190764E-15));
#32144=CARTESIAN_POINT('Ctrl Pts',(-36.1671666977136,-38.9021166528128,
2.30316661476457E-15));
#32145=CARTESIAN_POINT('Ctrl Pts',(-36.1111970366882,-38.922534339231,-1.9802954995054E-18));
#32146=CARTESIAN_POINT('Ctrl Pts',(-36.0547323436802,-38.9416301693299,
1.11022302462516E-16));
#32147=CARTESIAN_POINT('Ctrl Pts',(-38.5153122961063,-34.9971887940747,
7.11258330249198));
#32148=CARTESIAN_POINT('Ctrl Pts',(-38.5180434423612,-34.646197163443,7.09672411194512));
#32149=CARTESIAN_POINT('Ctrl Pts',(-38.4695960103246,-34.2959413770096,
7.08086492139826));
#32150=CARTESIAN_POINT('Ctrl Pts',(-38.3668188607358,-33.9624299204154,
7.0650057308514));
#32151=CARTESIAN_POINT('Ctrl Pts',(-38.0276669238477,-32.8618831847751,
7.01267235506732));
#32152=CARTESIAN_POINT('Ctrl Pts',(-37.0969085197677,-31.9436685919831,
6.96033897928324));
#32153=CARTESIAN_POINT('Ctrl Pts',(-35.9918738038683,-31.6194484086754,
6.90800560349915));
#32154=CARTESIAN_POINT('Ctrl Pts',(-34.8868390879688,-31.2952282253677,
6.85567222771507));
#32155=CARTESIAN_POINT('Ctrl Pts',(-33.6075280602499,-31.5650024515443,
6.80333885193098));
#32156=CARTESIAN_POINT('Ctrl Pts',(-32.7275159494446,-32.307828258462,6.75100547614689));
#32157=CARTESIAN_POINT('Ctrl Pts',(-31.8475038386392,-33.0506540653796,
6.69867210036281));
#32158=CARTESIAN_POINT('Ctrl Pts',(-31.3667906447475,-34.2665314530383,
6.64633872457873));
#32159=CARTESIAN_POINT('Ctrl Pts',(-31.5009114014496,-35.4103101350885,
6.59400534879465));
#32160=CARTESIAN_POINT('Ctrl Pts',(-31.6350321581518,-36.5540888171387,
6.54167197301056));
#32161=CARTESIAN_POINT('Ctrl Pts',(-32.3839868654478,-37.6257687935805,
6.48933859722647));
#32162=CARTESIAN_POINT('Ctrl Pts',(-33.4119756220756,-38.1448600989042,
6.43700522144239));
#32163=CARTESIAN_POINT('Ctrl Pts',(-34.4399643787034,-38.663951404228,6.3846718456583));
#32164=CARTESIAN_POINT('Ctrl Pts',(-35.7469871846628,-38.6304540384337,
6.33233846987422));
#32165=CARTESIAN_POINT('Ctrl Pts',(-36.7470353193051,-38.0593852703575,
6.28000509409014));
#32166=CARTESIAN_POINT('Ctrl Pts',(-37.7470834539474,-37.4883165022812,
6.22767171830606));
#32167=CARTESIAN_POINT('Ctrl Pts',(-38.4401569172725,-36.3796763319231,
6.17533834252197));
#32168=CARTESIAN_POINT('Ctrl Pts',(-38.5155122899541,-35.2305296102685,
6.12300496673788));
#32169=CARTESIAN_POINT('Ctrl Pts',(-38.5205143775731,-35.1542492816832,
6.11953107865591));
#32170=CARTESIAN_POINT('Ctrl Pts',(-38.5227946134492,-35.0777904690468,
6.11605719057395));
#32171=CARTESIAN_POINT('Ctrl Pts',(-38.522424122767,-35.0013091826171,6.11258330249198));
#32172=CARTESIAN_POINT('Origin',(35.,-35.,10.2084234471775));
#32173=CARTESIAN_POINT('Ctrl Pts',(30.9215903995924,-34.9979557257256,7.70842344717745));
#32174=CARTESIAN_POINT('Ctrl Pts',(30.9207462976534,-34.8668874511107,7.70328437820511));
#32175=CARTESIAN_POINT('Ctrl Pts',(30.9854756915705,-33.4019022214529,7.64581193344868));
#32176=CARTESIAN_POINT('Ctrl Pts',(32.753181490405,-30.7615622140283,7.53600611290817));
#32177=CARTESIAN_POINT('Ctrl Pts',(37.2955095733766,-30.7882306349807,7.3790059855559));
#32178=CARTESIAN_POINT('Ctrl Pts',(39.7793714317054,-34.5910508431566,7.22200585820367));
#32179=CARTESIAN_POINT('Ctrl Pts',(37.9775552386376,-38.7608686529102,7.0650057308514));
#32180=CARTESIAN_POINT('Ctrl Pts',(33.5057217267653,-39.5581360350982,6.90800560349915));
#32181=CARTESIAN_POINT('Ctrl Pts',(31.1346464724166,-37.067372389099,6.7891448422745));
#32182=CARTESIAN_POINT('Ctrl Pts',(30.9248236399074,-35.3669839150134,6.72261745683393));
#32183=CARTESIAN_POINT('Ctrl Pts',(30.9278856911952,-35.003454802609,6.70842344717745));
#32184=CARTESIAN_POINT('Ctrl Pts',(30.9308748007386,-35.0040807474719,7.79157655282254));
#32185=CARTESIAN_POINT('Ctrl Pts',(30.9370382125719,-34.10157834971,7.75638428364686));
#32186=CARTESIAN_POINT('Ctrl Pts',(31.6729756008745,-31.8449525580975,7.66885863868709));
#32187=CARTESIAN_POINT('Ctrl Pts',(35.3795267558193,-30.2191465582126,7.52899961794324));
#32188=CARTESIAN_POINT('Ctrl Pts',(39.1969165266342,-32.6774422642514,7.37199949059099));
#32189=CARTESIAN_POINT('Ctrl Pts',(39.2524336251343,-37.2202141105436,7.21499936323873));
#32190=CARTESIAN_POINT('Ctrl Pts',(35.4939867861423,-39.7711972931265,7.05799923588648));
#32191=CARTESIAN_POINT('Ctrl Pts',(31.7173198121032,-38.2186953257486,6.91685829908109));
#32192=CARTESIAN_POINT('Ctrl Pts',(30.9363086272988,-35.9315792701304,6.82805073805977));
#32193=CARTESIAN_POINT('Ctrl Pts',(30.9290344477858,-34.9967444478932,6.79157655282255));
#32194=CARTESIAN_POINT('Ctrl Pts',(37.6735319337713,-32.7141668369925,8.));
#32195=CARTESIAN_POINT('Ctrl Pts',(38.4251602751564,-33.5932784036374,7.94766662421592));
#32196=CARTESIAN_POINT('Ctrl Pts',(38.9814215765655,-36.1362159265307,7.84299987264775));
#32197=CARTESIAN_POINT('Ctrl Pts',(36.2450915261219,-38.9529260673994,7.6859997452955));
#32198=CARTESIAN_POINT('Ctrl Pts',(32.3914756047223,-38.2165112413961,7.52899961794324));
#32199=CARTESIAN_POINT('Ctrl Pts',(30.8773704214612,-34.5999494268526,7.37199949059098));
#32200=CARTESIAN_POINT('Ctrl Pts',(33.0598541530624,-31.3400748957517,7.21499936323873));
#32201=CARTESIAN_POINT('Ctrl Pts',(36.9821909719779,-31.3631032916521,7.05799923588648));
#32202=CARTESIAN_POINT('Ctrl Pts',(39.127025656321,-34.6468691152089,6.90099910853422));
#32203=CARTESIAN_POINT('Ctrl Pts',(37.5711428874206,-38.2475403183041,6.74399898118197));
#32204=CARTESIAN_POINT('Ctrl Pts',(33.7096786974094,-38.9359871126692,6.58699885382972));
#32205=CARTESIAN_POINT('Ctrl Pts',(31.005264414648,-36.0950579743517,6.42999872647747));
#32206=CARTESIAN_POINT('Ctrl Pts',(31.8829646703068,-32.272149334312,6.27299859912521));
#32207=CARTESIAN_POINT('Ctrl Pts',(35.5557419902844,-30.8953456995945,6.11599847177296));
#32208=CARTESIAN_POINT('Ctrl Pts',(38.7301793514647,-33.1992174379789,5.9589983444207));
#32209=CARTESIAN_POINT('Ctrl Pts',(38.5597294918745,-37.1178719063019,5.80199821706845));
#32210=CARTESIAN_POINT('Ctrl Pts',(35.1972358531438,-39.137408466637,5.6449980897162));
#32211=CARTESIAN_POINT('Ctrl Pts',(31.6578790286353,-37.4468920814909,5.48799796236395));
#32212=CARTESIAN_POINT('Ctrl Pts',(31.115434094392,-33.5622236362915,5.33099783501169));
#32213=CARTESIAN_POINT('Ctrl Pts',(34.0563166981778,-30.9668232762417,5.17399770765944));
#32214=CARTESIAN_POINT('Ctrl Pts',(37.8434091602659,-31.9880110645548,5.01699758030718));
#32215=CARTESIAN_POINT('Ctrl Pts',(39.0807893557322,-35.7100782827727,4.85999745295493));
#32216=CARTESIAN_POINT('Ctrl Pts',(36.6588865837055,-38.7954114649594,4.70299732560268));
#32217=CARTESIAN_POINT('Ctrl Pts',(32.7494442988629,-38.4773627887335,4.54599719825042));
#32218=CARTESIAN_POINT('Ctrl Pts',(30.8580969013801,-35.0411295327127,4.38899707089817));
#32219=CARTESIAN_POINT('Ctrl Pts',(32.6808337483856,-31.5680150335338,4.23199694354591));
#32220=CARTESIAN_POINT('Ctrl Pts',(36.5831892221451,-31.1723943770392,4.07499681619367));
#32221=CARTESIAN_POINT('Ctrl Pts',(39.0658837319978,-34.2090244039511,3.91799668884141));
#32222=CARTESIAN_POINT('Ctrl Pts',(37.9026612931367,-37.9549298355453,3.76099656148916));
#32223=CARTESIAN_POINT('Ctrl Pts',(34.1365946255998,-39.0511213358148,3.6039964341369));
#32224=CARTESIAN_POINT('Ctrl Pts',(31.144751840957,-36.5146334688211,3.44699630678465));
#32225=CARTESIAN_POINT('Ctrl Pts',(31.6099470650134,-32.6199592409358,3.2899961794324));
#32226=CARTESIAN_POINT('Ctrl Pts',(35.1150352807734,-30.8594903921659,3.13299605208014));
#32227=CARTESIAN_POINT('Ctrl Pts',(38.5169702522169,-32.811856236221,2.97599592472789));
#32228=CARTESIAN_POINT('Ctrl Pts',(38.7652042671773,-36.72635157484,2.81899579737563));
#32229=CARTESIAN_POINT('Ctrl Pts',(35.6371434759633,-39.0928109156136,2.66199567002339));
#32230=CARTESIAN_POINT('Ctrl Pts',(31.9377500537671,-37.7892074010372,2.50499554267113));
#32231=CARTESIAN_POINT('Ctrl Pts',(30.9843054629328,-33.9844949374723,2.34799541531888));
#32232=CARTESIAN_POINT('Ctrl Pts',(33.6317728360394,-31.0903954325918,2.19099528796662));
#32233=CARTESIAN_POINT('Ctrl Pts',(37.5061423356192,-31.7020761993063,2.03399516061437));
#32234=CARTESIAN_POINT('Ctrl Pts',(39.1332305596546,-35.2710361738983,1.87699503326212));
#32235=CARTESIAN_POINT('Ctrl Pts',(37.054010080289,-38.5969568276314,1.71999490590986));
#32236=CARTESIAN_POINT('Ctrl Pts',(33.1329414907541,-38.6974489325283,1.56299477855761));
#32237=CARTESIAN_POINT('Ctrl Pts',(30.8860772740811,-35.4824088577318,1.40599465120536));
#32238=CARTESIAN_POINT('Ctrl Pts',(32.3282169135405,-31.8347765477019,1.2489945238531));
#32239=CARTESIAN_POINT('Ctrl Pts',(36.1661501715419,-31.025453813021,1.09199439650085));
#32240=CARTESIAN_POINT('Ctrl Pts',(38.9584254909315,-33.7800977501094,0.934994269148596));
#32241=CARTESIAN_POINT('Ctrl Pts',(38.201061889907,-37.6287344800703,0.777994141796343));
#32242=CARTESIAN_POINT('Ctrl Pts',(34.5734381895487,-39.1199689001796,0.620994014444089));
#32243=CARTESIAN_POINT('Ctrl Pts',(31.3279885395076,-36.9171722692834,0.463993887091836));
#32244=CARTESIAN_POINT('Ctrl Pts',(31.3759276866332,-32.994453947074,0.306993759739581));
#32245=CARTESIAN_POINT('Ctrl Pts',(34.6722754393756,-30.8716903339078,0.149993632387328));
#32246=CARTESIAN_POINT('Ctrl Pts',(38.2651837481491,-32.4476574497985,-0.00700649496492499));
#32247=CARTESIAN_POINT('Ctrl Pts',(38.9246971357756,-36.3188846782332,-0.164006622317179));
#32248=CARTESIAN_POINT('Ctrl Pts',(37.0258557525633,-38.0994349533404,-0.268673373885348));
#32249=CARTESIAN_POINT('Ctrl Pts',(35.9084720925035,-38.3981590173419,-0.321006749669432));
#32250=CARTESIAN_POINT('Ctrl Pts',(37.8143974874483,-32.5937287191406,8.10700224988981));
#32251=CARTESIAN_POINT('Ctrl Pts',(38.6056283266121,-33.5191597390956,8.05466887410573));
#32252=CARTESIAN_POINT('Ctrl Pts',(39.1911984442813,-36.1960819350737,7.95000212253756));
#32253=CARTESIAN_POINT('Ctrl Pts',(36.3106940741934,-39.1612015370487,7.7930019951853));
#32254=CARTESIAN_POINT('Ctrl Pts',(32.2540352290981,-38.3859857972091,7.63600186783306));
#32255=CARTESIAN_POINT('Ctrl Pts',(30.6601534543285,-34.5788711876989,7.47900174048079));
#32256=CARTESIAN_POINT('Ctrl Pts',(32.9576299321766,-31.1472373351772,7.32200161312855));
#32257=CARTESIAN_POINT('Ctrl Pts',(37.0866305057775,-31.1714790727616,7.16500148577629));
#32258=CARTESIAN_POINT('Ctrl Pts',(39.3444742481158,-34.6282630245248,7.00800135842403));
#32259=CARTESIAN_POINT('Ctrl Pts',(37.7066136711597,-38.4186497631728,6.85100123107179));
#32260=CARTESIAN_POINT('Ctrl Pts',(33.641693040528,-39.1433700868122,6.69400110371952));
#32261=CARTESIAN_POINT('Ctrl Pts',(30.7947860459719,-36.1527554141754,6.53700097636728));
#32262=CARTESIAN_POINT('Ctrl Pts',(31.718731394466,-32.1284217844307,6.38000084901502));
#32263=CARTESIAN_POINT('Ctrl Pts',(35.5850234445937,-30.6790758307459,6.22300072166277));
#32264=CARTESIAN_POINT('Ctrl Pts',(38.9267185335935,-33.1043361203307,6.06600059431051));
#32265=CARTESIAN_POINT('Ctrl Pts',(38.747287852214,-37.2294603242033,5.90900046695826));
#32266=CARTESIAN_POINT('Ctrl Pts',(35.2076280004405,-39.3554041176628,5.75200033960601));
#32267=CARTESIAN_POINT('Ctrl Pts',(31.481786229765,-37.5758162224347,5.59500021225375));
#32268=CARTESIAN_POINT('Ctrl Pts',(30.9107604489508,-33.4864687290921,5.4380000849015));
#32269=CARTESIAN_POINT('Ctrl Pts',(34.0065950288281,-30.7543194848738,5.28099995754925));
#32270=CARTESIAN_POINT('Ctrl Pts',(37.9932253643036,-31.8293125714861,5.123999830197));
#32271=CARTESIAN_POINT('Ctrl Pts',(39.2958018060318,-35.7474915521612,4.96699970284474));
#32272=CARTESIAN_POINT('Ctrl Pts',(36.7462915531952,-38.995387657759,4.80999957549249));
#32273=CARTESIAN_POINT('Ctrl Pts',(32.6308649129514,-38.6605813351003,4.65299944814023));
#32274=CARTESIAN_POINT('Ctrl Pts',(30.6398644329761,-35.0432966040406,4.49599932078798));
#32275=CARTESIAN_POINT('Ctrl Pts',(32.5586393455524,-31.3871873963525,4.33899919343573));
#32276=CARTESIAN_POINT('Ctrl Pts',(36.6666057781757,-30.9707219083004,4.18199906608348));
#32277=CARTESIAN_POINT('Ctrl Pts',(39.2801108208385,-34.167348741179,4.02499893873122));
#32278=CARTESIAN_POINT('Ctrl Pts',(38.0555994290271,-38.1106219453356,3.86799881137897));
#32279=CARTESIAN_POINT('Ctrl Pts',(34.0911027148519,-39.2645706097038,3.71099868402672));
#32280=CARTESIAN_POINT('Ctrl Pts',(30.9416229163962,-36.5944378951337,3.55399855667446));
#32281=CARTESIAN_POINT('Ctrl Pts',(31.4313287819664,-32.494557425059,3.39699842932221));
#32282=CARTESIAN_POINT('Ctrl Pts',(35.1210963673509,-30.6413313453092,3.23999830196996));
#32283=CARTESIAN_POINT('Ctrl Pts',(38.7022756737031,-32.6965652688994,3.0829981746177));
#32284=CARTESIAN_POINT('Ctrl Pts',(38.963588874858,-36.8173112029482,2.92599804726545));
#32285=CARTESIAN_POINT('Ctrl Pts',(35.6707138879638,-39.3084567691156,2.76899791991319));
#32286=CARTESIAN_POINT('Ctrl Pts',(31.7764033615041,-37.9361677720372,2.61199779256094));
#32287=CARTESIAN_POINT('Ctrl Pts',(30.7727227893853,-33.9309890559499,2.45499766520869));
#32288=CARTESIAN_POINT('Ctrl Pts',(33.5596824021932,-30.8844025266947,2.29799753785643));
#32289=CARTESIAN_POINT('Ctrl Pts',(37.6381883094267,-31.5283121023449,2.14099741050418));
#32290=CARTESIAN_POINT('Ctrl Pts',(39.3510060812057,-35.2853167815919,1.98399728315193));
#32291=CARTESIAN_POINT('Ctrl Pts',(37.1622336865094,-38.7864766566921,1.82699715579967));
#32292=CARTESIAN_POINT('Ctrl Pts',(33.0345681639462,-38.8922635836996,1.66999702844742));
#32293=CARTESIAN_POINT('Ctrl Pts',(30.6693190617512,-35.5078264672934,1.51299690109517));
#32294=CARTESIAN_POINT('Ctrl Pts',(32.187443504768,-31.6680042909403,1.35599677374291));
#32295=CARTESIAN_POINT('Ctrl Pts',(36.2275933836127,-30.8160392022689,1.19899664639066));
#32296=CARTESIAN_POINT('Ctrl Pts',(39.1669907193568,-33.715822398208,1.04199651903841));
#32297=CARTESIAN_POINT('Ctrl Pts',(38.3697224358239,-37.7672397035641,0.884996391686155));
#32298=CARTESIAN_POINT('Ctrl Pts',(34.5509631015021,-39.3370456789998,0.7279962643339));
#32299=CARTESIAN_POINT('Ctrl Pts',(31.1345141616793,-37.0181860368003,0.570996136981647));
#32300=CARTESIAN_POINT('Ctrl Pts',(31.1849791714726,-32.8887838589028,0.413996009629392));
#32301=CARTESIAN_POINT('Ctrl Pts',(34.6550079808865,-30.6541740890041,0.256995882277139));
#32302=CARTESIAN_POINT('Ctrl Pts',(38.4372228065685,-32.313177235829,0.0999957549248859));
#32303=CARTESIAN_POINT('Ctrl Pts',(39.1314852530455,-36.3883753089936,-0.0570043724273679));
#32304=CARTESIAN_POINT('Ctrl Pts',(37.1325959372044,-38.2627408840732,-0.161671123995537));
#32305=CARTESIAN_POINT('Ctrl Pts',(35.9563385206894,-38.5772044012455,-0.214004499779622));
#32306=CARTESIAN_POINT('Ctrl Pts',(37.9552630411254,-32.4732906012887,8.21400449977962));
#32307=CARTESIAN_POINT('Ctrl Pts',(38.7860963780679,-33.4450410745538,8.16167112399554));
#32308=CARTESIAN_POINT('Ctrl Pts',(39.400975311997,-36.2559479436168,8.05700437242737));
#32309=CARTESIAN_POINT('Ctrl Pts',(36.3762966222648,-39.369477006698,7.90000424507512));
#32310=CARTESIAN_POINT('Ctrl Pts',(32.1165948534739,-38.5554603530221,7.74300411772285));
#32311=CARTESIAN_POINT('Ctrl Pts',(30.4429364871958,-34.5577929485451,7.58600399037062));
#32312=CARTESIAN_POINT('Ctrl Pts',(32.8554057112908,-30.9543997746027,7.42900386301835));
#32313=CARTESIAN_POINT('Ctrl Pts',(37.191070039577,-30.9798548538712,7.2720037356661));
#32314=CARTESIAN_POINT('Ctrl Pts',(39.5619228399106,-34.6096569338406,7.11500360831384));
#32315=CARTESIAN_POINT('Ctrl Pts',(37.8420844548986,-38.5897592080416,6.9580034809616));
#32316=CARTESIAN_POINT('Ctrl Pts',(33.5737073836467,-39.3507530609551,6.80100335360933));
#32317=CARTESIAN_POINT('Ctrl Pts',(30.5843076772956,-36.2104528539991,6.64400322625709));
#32318=CARTESIAN_POINT('Ctrl Pts',(31.5544981186253,-31.9846942345494,6.48700309890483));
#32319=CARTESIAN_POINT('Ctrl Pts',(35.6143048989029,-30.4628059618972,6.33000297155259));
#32320=CARTESIAN_POINT('Ctrl Pts',(39.1232577157224,-33.0094548026823,6.17300284420032));
#32321=CARTESIAN_POINT('Ctrl Pts',(38.9348462125535,-37.3410487421046,6.01600271684808));
#32322=CARTESIAN_POINT('Ctrl Pts',(35.2180201477371,-39.5733997686886,5.85900258949581));
#32323=CARTESIAN_POINT('Ctrl Pts',(31.3056934308947,-37.7047403633785,5.70200246214358));
#32324=CARTESIAN_POINT('Ctrl Pts',(30.7060868035096,-33.4107138218927,5.54500233479131));
#32325=CARTESIAN_POINT('Ctrl Pts',(33.9568733594783,-30.5418156935059,5.38800220743906));
#32326=CARTESIAN_POINT('Ctrl Pts',(38.1430415683413,-31.6706140784174,5.2310020800868));
#32327=CARTESIAN_POINT('Ctrl Pts',(39.5108142563315,-35.7849048215497,5.07400195273456));
#32328=CARTESIAN_POINT('Ctrl Pts',(36.8336965226849,-39.1953638505585,4.9170018253823));
#32329=CARTESIAN_POINT('Ctrl Pts',(32.5122855270398,-38.8437998814671,4.76000169803005));
#32330=CARTESIAN_POINT('Ctrl Pts',(30.4216319645722,-35.0454636753686,4.60300157067779));
#32331=CARTESIAN_POINT('Ctrl Pts',(32.4364449427192,-31.2063597591713,4.44600144332554));
#32332=CARTESIAN_POINT('Ctrl Pts',(36.7500223342062,-30.7690494395616,4.28900131597329));
#32333=CARTESIAN_POINT('Ctrl Pts',(39.4943379096791,-34.1256730784068,4.13200118862103));
#32334=CARTESIAN_POINT('Ctrl Pts',(38.2085375649176,-38.266314055126,3.97500106126878));
#32335=CARTESIAN_POINT('Ctrl Pts',(34.0456108041041,-39.4780198835927,3.81800093391653));
#32336=CARTESIAN_POINT('Ctrl Pts',(30.7384939918355,-36.6742423214464,3.66100080656427));
#32337=CARTESIAN_POINT('Ctrl Pts',(31.2527104989195,-32.3691556091822,3.50400067921202));
#32338=CARTESIAN_POINT('Ctrl Pts',(35.1271574539286,-30.4231722984524,3.34700055185977));
#32339=CARTESIAN_POINT('Ctrl Pts',(38.8875810951892,-32.5812743015779,3.19000042450751));
#32340=CARTESIAN_POINT('Ctrl Pts',(39.1619734825387,-36.9082708310562,3.03300029715526));
#32341=CARTESIAN_POINT('Ctrl Pts',(35.7042842999643,-39.5241026226178,2.876000169803));
#32342=CARTESIAN_POINT('Ctrl Pts',(31.6150566692411,-38.083128143037,2.71900004245075));
#32343=CARTESIAN_POINT('Ctrl Pts',(30.5611401158378,-33.8774831744275,2.5619999150985));
#32344=CARTESIAN_POINT('Ctrl Pts',(33.487591968347,-30.6784096207976,2.40499978774624));
#32345=CARTESIAN_POINT('Ctrl Pts',(37.7702342832343,-31.3545480053834,2.24799966039399));
#32346=CARTESIAN_POINT('Ctrl Pts',(39.5687816027568,-35.2995973892856,2.09099953304174));
#32347=CARTESIAN_POINT('Ctrl Pts',(37.2704572927298,-38.9759964857528,1.93399940568948));
#32348=CARTESIAN_POINT('Ctrl Pts',(32.9361948371383,-39.087078234871,1.77699927833723));
#32349=CARTESIAN_POINT('Ctrl Pts',(30.4525608494213,-35.533244076855,1.61999915098498));
#32350=CARTESIAN_POINT('Ctrl Pts',(32.0466700959956,-31.5012320341786,1.46299902363273));
#32351=CARTESIAN_POINT('Ctrl Pts',(36.2890365956835,-30.606624591517,1.30599889628047));
#32352=CARTESIAN_POINT('Ctrl Pts',(39.3755559477821,-33.6515470463066,1.14899876892822));
#32353=CARTESIAN_POINT('Ctrl Pts',(38.5383829817409,-37.905744927058,0.991998641575965));
#32354=CARTESIAN_POINT('Ctrl Pts',(34.5284880134556,-39.55412245782,0.83499851422371));
#32355=CARTESIAN_POINT('Ctrl Pts',(30.9410397838509,-37.1191998043172,0.677998386871458));
#32356=CARTESIAN_POINT('Ctrl Pts',(30.9940306563121,-32.7831137707316,0.520998259519202));
#32357=CARTESIAN_POINT('Ctrl Pts',(34.6377405223973,-30.4366578441002,0.36399813216695));
#32358=CARTESIAN_POINT('Ctrl Pts',(38.6092618649879,-32.1786970218597,0.206998004814696));
#32359=CARTESIAN_POINT('Ctrl Pts',(39.3382733703155,-36.4578659397538,0.0499978774624431));
#32360=CARTESIAN_POINT('Ctrl Pts',(37.2393361218455,-38.4260468148059,-0.0546688741057264));
#32361=CARTESIAN_POINT('Ctrl Pts',(36.0042049488753,-38.756249785149,-0.107002249889811));
#32362=CARTESIAN_POINT('Ctrl Pts',(38.0961285948024,-32.3528524834367,8.32100674966943));
#32363=CARTESIAN_POINT('Ctrl Pts',(38.9665644295237,-33.3709224100119,8.26867337388535));
#32364=CARTESIAN_POINT('Ctrl Pts',(39.6107521797128,-36.3158139521599,8.16400662231718));
#32365=CARTESIAN_POINT('Ctrl Pts',(36.4418991703362,-39.5777524763472,8.00700649496493));
#32366=CARTESIAN_POINT('Ctrl Pts',(31.9791544778497,-38.724934908835,7.85000636761268));
#32367=CARTESIAN_POINT('Ctrl Pts',(30.2257195200631,-34.5367147093914,7.69300624026041));
#32368=CARTESIAN_POINT('Ctrl Pts',(32.753181490405,-30.7615622140283,7.53600611290817));
#32369=CARTESIAN_POINT('Ctrl Pts',(37.2955095733766,-30.7882306349807,7.3790059855559));
#32370=CARTESIAN_POINT('Ctrl Pts',(39.7793714317054,-34.5910508431566,7.22200585820367));
#32371=CARTESIAN_POINT('Ctrl Pts',(37.9775552386376,-38.7608686529102,7.0650057308514));
#32372=CARTESIAN_POINT('Ctrl Pts',(33.5057217267653,-39.5581360350982,6.90800560349915));
#32373=CARTESIAN_POINT('Ctrl Pts',(30.3738293086194,-36.2681502938228,6.7510054761469));
#32374=CARTESIAN_POINT('Ctrl Pts',(31.3902648427845,-31.8409666846681,6.59400534879465));
#32375=CARTESIAN_POINT('Ctrl Pts',(35.6435863532121,-30.2465360930486,6.43700522144239));
#32376=CARTESIAN_POINT('Ctrl Pts',(39.3197968978512,-32.9145734850341,6.28000509409014));
#32377=CARTESIAN_POINT('Ctrl Pts',(39.1224045728929,-37.4526371600059,6.12300496673789));
#32378=CARTESIAN_POINT('Ctrl Pts',(35.2284122950338,-39.7913954197145,5.96600483938562));
#32379=CARTESIAN_POINT('Ctrl Pts',(31.1296006320244,-37.8336645043222,5.80900471203338));
#32380=CARTESIAN_POINT('Ctrl Pts',(30.5014131580684,-33.3349589146933,5.65200458468112));
#32381=CARTESIAN_POINT('Ctrl Pts',(33.9071516901285,-30.3293119021379,5.49500445732887));
#32382=CARTESIAN_POINT('Ctrl Pts',(38.292857772379,-31.5119155853487,5.33800432997662));
#32383=CARTESIAN_POINT('Ctrl Pts',(39.7258267066312,-35.8223180909381,5.18100420262436));
#32384=CARTESIAN_POINT('Ctrl Pts',(36.9211014921746,-39.3953400433581,5.02400407527211));
#32385=CARTESIAN_POINT('Ctrl Pts',(32.3937061411281,-39.0270184278339,4.86700394791986));
#32386=CARTESIAN_POINT('Ctrl Pts',(30.2033994961682,-35.0476307466965,4.7100038205676));
#32387=CARTESIAN_POINT('Ctrl Pts',(32.314250539886,-31.02553212199,4.55300369321535));
#32388=CARTESIAN_POINT('Ctrl Pts',(36.8334388902368,-30.5673769708228,4.39600356586309));
#32389=CARTESIAN_POINT('Ctrl Pts',(39.7085649985197,-34.0839974156347,4.23900343851085));
#32390=CARTESIAN_POINT('Ctrl Pts',(38.3614757008081,-38.4220061649164,4.08200331115859));
#32391=CARTESIAN_POINT('Ctrl Pts',(34.0001188933562,-39.6914691574817,3.92500318380634));
#32392=CARTESIAN_POINT('Ctrl Pts',(30.5353650672746,-36.754046747759,3.76800305645408));
#32393=CARTESIAN_POINT('Ctrl Pts',(31.0740922158726,-32.2437537933055,3.61100292910183));
#32394=CARTESIAN_POINT('Ctrl Pts',(35.1332185405061,-30.2050132515957,3.45400280174957));
#32395=CARTESIAN_POINT('Ctrl Pts',(39.0728865166754,-32.4659833342563,3.29700267439732));
#32396=CARTESIAN_POINT('Ctrl Pts',(39.3603580902194,-36.9992304591644,3.14000254704507));
#32397=CARTESIAN_POINT('Ctrl Pts',(35.7378547119649,-39.73974847612,2.98300241969282));
#32398=CARTESIAN_POINT('Ctrl Pts',(31.453709976978,-38.2300885140369,2.82600229234056));
#32399=CARTESIAN_POINT('Ctrl Pts',(30.3495574422904,-33.8239772929051,2.66900216498831));
#32400=CARTESIAN_POINT('Ctrl Pts',(33.4155015345008,-30.4724167149005,2.51200203763606));
#32401=CARTESIAN_POINT('Ctrl Pts',(37.9022802570419,-31.180783908422,2.3550019102838));
#32402=CARTESIAN_POINT('Ctrl Pts',(39.7865571243079,-35.3138779969793,2.19800178293155));
#32403=CARTESIAN_POINT('Ctrl Pts',(37.3786808989502,-39.1655163148135,2.04100165557929));
#32404=CARTESIAN_POINT('Ctrl Pts',(32.8378215103303,-39.2818928860424,1.88400152822704));
#32405=CARTESIAN_POINT('Ctrl Pts',(30.2358026370915,-35.5586616864166,1.72700140087479));
#32406=CARTESIAN_POINT('Ctrl Pts',(31.9058966872231,-31.3344597774169,1.57000127352254));
#32407=CARTESIAN_POINT('Ctrl Pts',(36.3504798077544,-30.397209980765,1.41300114617028));
#32408=CARTESIAN_POINT('Ctrl Pts',(39.5841211762074,-33.5872716944053,1.25600101881803));
#32409=CARTESIAN_POINT('Ctrl Pts',(38.7070435276578,-38.0442501505519,1.09900089146578));
#32410=CARTESIAN_POINT('Ctrl Pts',(34.5060129254091,-39.7711992366401,0.942000764113522));
#32411=CARTESIAN_POINT('Ctrl Pts',(30.7475654060226,-37.220213571834,0.785000636761267));
#32412=CARTESIAN_POINT('Ctrl Pts',(30.8030821411515,-32.6774436825603,0.628000509409014));
#32413=CARTESIAN_POINT('Ctrl Pts',(34.6204730639081,-30.2191415991965,0.471000382056761));
#32414=CARTESIAN_POINT('Ctrl Pts',(38.7813009234074,-32.0442168078902,0.314000254704507));
#32415=CARTESIAN_POINT('Ctrl Pts',(39.5450614875854,-36.5273565705141,0.157000127352254));
#32416=CARTESIAN_POINT('Ctrl Pts',(37.3460763064866,-38.5893527455387,0.0523333757840845));
#32417=CARTESIAN_POINT('Ctrl Pts',(36.0520713770612,-38.9352951690526,0.));
#32418=CARTESIAN_POINT('Ctrl Pts',(36.0520713770612,-38.9352951690526,0.));
#32419=CARTESIAN_POINT('Ctrl Pts',(36.1681792863691,-38.8956805730896,-1.36202072051053E-17));
#32420=CARTESIAN_POINT('Ctrl Pts',(36.2820221354364,-38.8505155517789,2.68655360649277E-15));
#32421=CARTESIAN_POINT('Ctrl Pts',(36.3933740322884,-38.80015771728,1.94289029309402E-15));
#32422=CARTESIAN_POINT('Ctrl Pts',(36.5072231634749,-38.7486705323445,1.18254920758684E-15));
#32423=CARTESIAN_POINT('Ctrl Pts',(36.6184689861953,-38.6917545108625,4.54098351417643E-16));
#32424=CARTESIAN_POINT('Ctrl Pts',(36.7268457946485,-38.6297432931302,1.66533453693773E-16));
#32425=CARTESIAN_POINT('Ctrl Pts',(36.8407841942848,-38.56454983515,-1.35788460984399E-16));
#32426=CARTESIAN_POINT('Ctrl Pts',(36.9515525365026,-38.4937243961273,-1.82271800722416E-15));
#32427=CARTESIAN_POINT('Ctrl Pts',(37.0588029145039,-38.4176084656939,-1.99840144432528E-15));
#32428=CARTESIAN_POINT('Ctrl Pts',(37.1526469952551,-38.3510070265646,-2.15212445178876E-15));
#32429=CARTESIAN_POINT('Ctrl Pts',(37.2437973301633,-38.2803539972376,-9.7785017405382E-16));
#32430=CARTESIAN_POINT('Ctrl Pts',(37.3319893511255,-38.2058560072044,-8.88178419700125E-16));
#32431=CARTESIAN_POINT('Ctrl Pts',(37.3493647837374,-38.1911785478217,-8.70511452689226E-16));
#32432=CARTESIAN_POINT('Ctrl Pts',(37.3666252839799,-38.1763517900465,-1.48427532953915E-15));
#32433=CARTESIAN_POINT('Ctrl Pts',(37.3837686739948,-38.1613772431262,-1.55431223447522E-15));
#32434=CARTESIAN_POINT('Ctrl Pts',(37.3963029962073,-38.1504286620158,-1.60551944217877E-15));
#32435=CARTESIAN_POINT('Ctrl Pts',(37.4087735029071,-38.139402069251,-1.97641509759958E-15));
#32436=CARTESIAN_POINT('Ctrl Pts',(37.4211705433933,-38.1283061781123,-1.88737914186277E-15));
#32437=CARTESIAN_POINT('Ctrl Pts',(37.5137497678178,-38.0454437403337,-1.22247208301798E-15));
#32438=CARTESIAN_POINT('Ctrl Pts',(37.6023731431382,-37.9585995914834,-1.41571360075421E-15));
#32439=CARTESIAN_POINT('Ctrl Pts',(37.6867792446409,-37.8680946551148,-1.63757896132211E-15));
#32440=CARTESIAN_POINT('Ctrl Pts',(37.7709936181979,-37.7777953001582,-1.85894035607411E-15));
#32441=CARTESIAN_POINT('Ctrl Pts',(37.8510103725839,-37.6838510649778,4.27670315709133E-16));
#32442=CARTESIAN_POINT('Ctrl Pts',(37.9265294316329,-37.5865486541875,7.49400541621981E-16));
#32443=CARTESIAN_POINT('Ctrl Pts',(38.0010161819357,-37.4905763199493,1.06673287208574E-15));
#32444=CARTESIAN_POINT('Ctrl Pts',(38.0711277582919,-37.3913363066692,-2.10142620498032E-15));
#32445=CARTESIAN_POINT('Ctrl Pts',(38.1365301844556,-37.2890828938187,-2.44249065417534E-15));
#32446=CARTESIAN_POINT('Ctrl Pts',(38.1898358473465,-37.2057421635956,-2.72047218512562E-15));
#32447=CARTESIAN_POINT('Ctrl Pts',(38.2400125268915,-37.1203991308186,-6.32482117348439E-16));
#32448=CARTESIAN_POINT('Ctrl Pts',(38.2868534572638,-37.0331856293588,-5.55111512312578E-16));
#32449=CARTESIAN_POINT('Ctrl Pts',(38.2987532893997,-37.0110292370944,-5.35455685563087E-16));
#32450=CARTESIAN_POINT('Ctrl Pts',(38.3104377056016,-36.9887521084602,-5.70989169773688E-17));
#32451=CARTESIAN_POINT('Ctrl Pts',(38.3219030525931,-36.9663563797929,-2.77555756156289E-17));
#32452=CARTESIAN_POINT('Ctrl Pts',(38.3300600637675,-36.9504229580542,-6.87928085047562E-18));
#32453=CARTESIAN_POINT('Ctrl Pts',(38.3381024804697,-36.9344366850298,-1.37102362174578E-15));
#32454=CARTESIAN_POINT('Ctrl Pts',(38.3460266349626,-36.9184039879293,-1.33226762955019E-15));
#32455=CARTESIAN_POINT('Ctrl Pts',(38.3989875306322,-36.8112498430667,-1.07324288929609E-15));
#32456=CARTESIAN_POINT('Ctrl Pts',(38.4467095755205,-36.7019458397232,2.38645293041498E-15));
#32457=CARTESIAN_POINT('Ctrl Pts',(38.4889139708526,-36.5907545955107,1.9151347174784E-15));
#32458=CARTESIAN_POINT('Ctrl Pts',(38.5302822088046,-36.4817662825029,1.45315430452751E-15));
#32459=CARTESIAN_POINT('Ctrl Pts',(38.5663495354543,-36.3709641352684,1.27266374069395E-15));
#32460=CARTESIAN_POINT('Ctrl Pts',(38.5968051838807,-36.2585816849604,1.52655665885959E-15));
#32461=CARTESIAN_POINT('Ctrl Pts',(38.6012594551821,-36.2421452618648,1.56368960455097E-15));
#32462=CARTESIAN_POINT('Ctrl Pts',(38.6055936009628,-36.2256750205659,1.48568813827467E-15));
#32463=CARTESIAN_POINT('Ctrl Pts',(38.6098065549286,-36.2091716785531,1.47104550762833E-15));
#32464=CARTESIAN_POINT('Ctrl Pts',(38.6394751128162,-36.092951477284,1.34152120378576E-15));
#32465=CARTESIAN_POINT('Ctrl Pts',(38.6631376928158,-35.9750893748381,9.72065328759131E-16));
#32466=CARTESIAN_POINT('Ctrl Pts',(38.6808851493713,-35.856021209443,1.41553435639707E-15));
#32467=CARTESIAN_POINT('Ctrl Pts',(38.6908686963668,-35.7890413229915,1.66500074413739E-15));
#32468=CARTESIAN_POINT('Ctrl Pts',(38.6989794822973,-35.7216798344703,1.48644827793188E-15));
#32469=CARTESIAN_POINT('Ctrl Pts',(38.7052266318381,-35.6540157826807,1.55431223447522E-15));
#32470=CARTESIAN_POINT('Ctrl Pts',(38.7081091139172,-35.6227950770761,1.58562517764618E-15));
#32471=CARTESIAN_POINT('Ctrl Pts',(38.7105947647117,-35.591509978624,7.00070747597251E-16));
#32472=CARTESIAN_POINT('Ctrl Pts',(38.7126841330784,-35.5601683863959,6.66133814775094E-16));
#32473=CARTESIAN_POINT('Ctrl Pts',(38.7138852254902,-35.5421513870013,6.46624860231182E-16));
#32474=CARTESIAN_POINT('Ctrl Pts',(38.7149548469422,-35.5241227721236,2.63074882680395E-16));
#32475=CARTESIAN_POINT('Ctrl Pts',(38.7158930667035,-35.5060923822785,2.77555756156289E-16));
#32476=CARTESIAN_POINT('Ctrl Pts',(38.7222040106739,-35.3848107969113,3.74961486578641E-16));
#32477=CARTESIAN_POINT('Ctrl Pts',(38.7225824292358,-35.263331928612,-1.41858650592555E-15));
#32478=CARTESIAN_POINT('Ctrl Pts',(38.717186529709,-35.1421030264707,-9.99200722162641E-16));
#32479=CARTESIAN_POINT('Ctrl Pts',(38.7119025633842,-35.0233889115555,-5.88514728574682E-16));
#32480=CARTESIAN_POINT('Ctrl Pts',(38.7010808603444,-34.9049135759813,2.80055440532142E-15));
#32481=CARTESIAN_POINT('Ctrl Pts',(38.6848166129475,-34.7871029976449,2.56739074444567E-15));
#32482=CARTESIAN_POINT('Ctrl Pts',(38.6687112711112,-34.6704434566446,2.3365051479245E-15));
#32483=CARTESIAN_POINT('Ctrl Pts',(38.6472688652681,-34.5544349100609,2.77413847088875E-15));
#32484=CARTESIAN_POINT('Ctrl Pts',(38.6205350417295,-34.4395098718885,3.02535774210355E-15));
#32485=CARTESIAN_POINT('Ctrl Pts',(38.6031281553353,-34.3646800563773,3.18893125068641E-15));
#32486=CARTESIAN_POINT('Ctrl Pts',(38.583477007896,-34.2903100135713,5.83132516188889E-16));
#32487=CARTESIAN_POINT('Ctrl Pts',(38.5615843988617,-34.2165260396906,2.91433543964104E-16));
#32488=CARTESIAN_POINT('Ctrl Pts',(38.5541960449916,-34.1916253022719,1.92990492842735E-16));
#32489=CARTESIAN_POINT('Ctrl Pts',(38.5465523399986,-34.1667913689833,-1.55624678416612E-15));
#32490=CARTESIAN_POINT('Ctrl Pts',(38.5386532038413,-34.1420292711584,-1.62370117351429E-15));
#32491=CARTESIAN_POINT('Ctrl Pts',(38.5335667843701,-34.1260844369365,-1.66713646980058E-15));
#32492=CARTESIAN_POINT('Ctrl Pts',(38.5283752457655,-34.1101719998602,9.92420310992954E-16));
#32493=CARTESIAN_POINT('Ctrl Pts',(38.5230814471938,-34.0943013261403,9.71445146547012E-16));
#32494=CARTESIAN_POINT('Ctrl Pts',(38.4861837828756,-33.9836830652666,8.25248693044116E-16));
#32495=CARTESIAN_POINT('Ctrl Pts',(38.4442854059965,-33.8749762815042,4.28212832527473E-15));
#32496=CARTESIAN_POINT('Ctrl Pts',(38.3974511090383,-33.7686001708186,3.23352455922077E-15));
#32497=CARTESIAN_POINT('Ctrl Pts',(38.359337050901,-33.6820305940251,2.38016393467622E-15));
#32498=CARTESIAN_POINT('Ctrl Pts',(38.3179530879923,-33.5970047635678,1.69064823388315E-15));
#32499=CARTESIAN_POINT('Ctrl Pts',(38.2733131581435,-33.5137642691618,1.70696790036118E-15));
#32500=CARTESIAN_POINT('Ctrl Pts',(38.251698175988,-33.473458609917,1.71487000282641E-15));
#32501=CARTESIAN_POINT('Ctrl Pts',(38.2293195396252,-33.4335717773559,1.04902033086069E-15));
#32502=CARTESIAN_POINT('Ctrl Pts',(38.2061773582038,-33.3941327240688,1.01307850997046E-15));
#32503=CARTESIAN_POINT('Ctrl Pts',(38.1925909929398,-33.3709787536688,9.91977702834968E-16));
#32504=CARTESIAN_POINT('Ctrl Pts',(38.1787393972074,-33.347976051224,-1.47665884113671E-16));
#32505=CARTESIAN_POINT('Ctrl Pts',(38.1646366459175,-33.3251529677485,-1.38777878078145E-17));
#32506=CARTESIAN_POINT('Ctrl Pts',(38.1062051944783,-33.230590859521,5.40441897174675E-16));
#32507=CARTESIAN_POINT('Ctrl Pts',(38.0434224756675,-33.1390339550006,1.08623518571526E-16));
#32508=CARTESIAN_POINT('Ctrl Pts',(37.9763225348264,-33.0508729636923,6.24500451351651E-16));
#32509=CARTESIAN_POINT('Ctrl Pts',(37.9162918094667,-32.9720000438309,1.08602792936337E-15));
#32510=CARTESIAN_POINT('Ctrl Pts',(37.8528049873413,-32.8958452375375,9.00746847309969E-16));
#32511=CARTESIAN_POINT('Ctrl Pts',(37.7858629582169,-32.8227148526165,3.72098185597025E-16));
#32512=CARTESIAN_POINT('Ctrl Pts',(37.7510080319419,-32.784637814794,1.2084137301326E-16));
#32513=CARTESIAN_POINT('Ctrl Pts',(37.7152160018646,-32.7473811866193,3.2434591796547E-16));
#32514=CARTESIAN_POINT('Ctrl Pts',(37.6785242770714,-32.7109603660126,2.77555756156289E-16));
#32515=CARTESIAN_POINT('Ctrl Pts',(31.4836965554877,-35.0029832498286,6.38741669750802));
#32516=CARTESIAN_POINT('Ctrl Pts',(31.4810524495825,-35.31689356108,6.4016107071645));
#32517=CARTESIAN_POINT('Ctrl Pts',(31.519709060091,-35.6301638289998,6.41580471682099));
#32518=CARTESIAN_POINT('Ctrl Pts',(31.6022835043847,-35.9313947240647,6.42999872647747));
#32519=CARTESIAN_POINT('Ctrl Pts',(31.9067358422351,-37.0420343537909,6.48233210226155));
#32520=CARTESIAN_POINT('Ctrl Pts',(32.8082072698223,-37.98901073323,6.53466547804564));
#32521=CARTESIAN_POINT('Ctrl Pts',(33.9025203486177,-38.3477577905554,6.58699885382972));
#32522=CARTESIAN_POINT('Ctrl Pts',(34.9968334274131,-38.7065048478808,6.6393322296138));
#32523=CARTESIAN_POINT('Ctrl Pts',(36.2839881574169,-38.4770225830925,6.69166560539789));
#32524=CARTESIAN_POINT('Ctrl Pts',(37.1868793172355,-37.7621695835158,6.74399898118197));
#32525=CARTESIAN_POINT('Ctrl Pts',(38.0897704770541,-37.0473165839391,6.79633235696606));
#32526=CARTESIAN_POINT('Ctrl Pts',(38.6083980666875,-35.847092849574,6.84866573275014));
#32527=CARTESIAN_POINT('Ctrl Pts',(38.5102394141138,-34.6996866784653,6.90099910853423));
#32528=CARTESIAN_POINT('Ctrl Pts',(38.41208076154,-33.5522805073566,6.95333248431831));
#32529=CARTESIAN_POINT('Ctrl Pts',(37.697135866759,-32.4576918995043,7.0056658601024));
#32530=CARTESIAN_POINT('Ctrl Pts',(36.6859406162159,-31.9065595295948,7.05799923588648));
#32531=CARTESIAN_POINT('Ctrl Pts',(35.6747453656728,-31.3554271596853,7.11033261167057));
#32532=CARTESIAN_POINT('Ctrl Pts',(34.3672997593676,-31.3477510277185,7.16266598745465));
#32533=CARTESIAN_POINT('Ctrl Pts',(33.3498296676148,-31.8872253835852,7.21499936323873));
#32534=CARTESIAN_POINT('Ctrl Pts',(32.332359575862,-32.426699739452,7.26733273902282));
#32535=CARTESIAN_POINT('Ctrl Pts',(31.6048649986616,-33.5133245831523,7.3196661148069));
#32536=CARTESIAN_POINT('Ctrl Pts',(31.4934685739382,-34.6593973074264,7.37199949059099));
#32537=CARTESIAN_POINT('Ctrl Pts',(31.4825295909021,-34.7719401481876,7.37713855956333));
#32538=CARTESIAN_POINT('Ctrl Pts',(31.4775316317653,-34.8850562438399,7.38227762853568));
#32539=CARTESIAN_POINT('Ctrl Pts',(31.478260520576,-34.9982347527286,7.38741669750802));
#32540=CARTESIAN_POINT('Ctrl Pts',(33.9479286229388,-38.9352951690526,8.));
#32541=CARTESIAN_POINT('Ctrl Pts',(32.6539236935135,-38.5893527455387,7.94766662421592));
#32542=CARTESIAN_POINT('Ctrl Pts',(30.4549361873396,-36.5273716142364,7.84299987264774));
#32543=CARTESIAN_POINT('Ctrl Pts',(31.2187010881653,-32.044211167377,7.68599974529549));
#32544=CARTESIAN_POINT('Ctrl Pts',(35.3795267558193,-30.2191465582126,7.52899961794324));
#32545=CARTESIAN_POINT('Ctrl Pts',(39.1969165266342,-32.6774422642514,7.37199949059099));
#32546=CARTESIAN_POINT('Ctrl Pts',(39.2524336251343,-37.2202141105436,7.21499936323873));
#32547=CARTESIAN_POINT('Ctrl Pts',(35.4939867861423,-39.7711972931265,7.05799923588648));
#32548=CARTESIAN_POINT('Ctrl Pts',(31.292957592828,-38.0442496611363,6.90099910853423));
#32549=CARTESIAN_POINT('Ctrl Pts',(30.4158800177777,-33.5872718945856,6.74399898118197));
#32550=CARTESIAN_POINT('Ctrl Pts',(33.6495206016122,-30.3972113452741,6.58699885382972));
#32551=CARTESIAN_POINT('Ctrl Pts',(38.09410244091,-31.3344607296745,6.42999872647747));
#32552=CARTESIAN_POINT('Ctrl Pts',(39.7641960678496,-35.558661561786,6.27299859912521));
#32553=CARTESIAN_POINT('Ctrl Pts',(37.1621778889461,-39.2818916953666,6.11599847177296));
#32554=CARTESIAN_POINT('Ctrl Pts',(32.6213197580022,-39.1655151793351,5.95899834442071));
#32555=CARTESIAN_POINT('Ctrl Pts',(30.2134441875202,-35.3138779065921,5.80199821706845));
#32556=CARTESIAN_POINT('Ctrl Pts',(32.0977205408613,-31.1807849590781,5.6449980897162));
#32557=CARTESIAN_POINT('Ctrl Pts',(36.584498029893,-30.4724179566463,5.48799796236395));
#32558=CARTESIAN_POINT('Ctrl Pts',(39.6504412814188,-33.8239776163473,5.33099783501169));
#32559=CARTESIAN_POINT('Ctrl Pts',(38.5462890493217,-38.2300876270061,5.17399770765944));
#32560=CARTESIAN_POINT('Ctrl Pts',(34.2621454906851,-39.7397471751372,5.01699758030718));
#32561=CARTESIAN_POINT('Ctrl Pts',(30.6396431067263,-36.9992299102556,4.85999745295493));
#32562=CARTESIAN_POINT('Ctrl Pts',(30.9271146014312,-32.4659840299328,4.70299732560268));
#32563=CARTESIAN_POINT('Ctrl Pts',(34.8667814960507,-30.2050145678827,4.54599719825042));
#32564=CARTESIAN_POINT('Ctrl Pts',(38.9259067064028,-32.2437545499559,4.38899707089817));
#32565=CARTESIAN_POINT('Ctrl Pts',(39.4646337070995,-36.7540462662356,4.23199694354592));
#32566=CARTESIAN_POINT('Ctrl Pts',(35.9998808321606,-39.6914678695931,4.07499681619366));
#32567=CARTESIAN_POINT('Ctrl Pts',(31.6385252219761,-38.4220052255121,3.91799668884141));
#32568=CARTESIAN_POINT('Ctrl Pts',(30.291436294066,-34.0839976670965,3.76099656148916));
#32569=CARTESIAN_POINT('Ctrl Pts',(33.1665616130745,-30.567378187653,3.6039964341369));
#32570=CARTESIAN_POINT('Ctrl Pts',(37.6857487228281,-31.0255332130596,3.44699630678465));
#32571=CARTESIAN_POINT('Ctrl Pts',(39.7965991870786,-35.0476307336073,3.28999617943239));
#32572=CARTESIAN_POINT('Ctrl Pts',(37.606293143399,-39.0270173223719,3.13299605208014));
#32573=CARTESIAN_POINT('Ctrl Pts',(33.0788990351993,-39.3953388367078,2.97599592472789));
#32574=CARTESIAN_POINT('Ctrl Pts',(30.2741745906988,-35.8223178652953,2.81899579737564));
#32575=CARTESIAN_POINT('Ctrl Pts',(31.7071431315558,-31.5119165427019,2.66199567002338));
#32576=CARTESIAN_POINT('Ctrl Pts',(36.092848009894,-30.329313184686,2.50499554267113));
#32577=CARTESIAN_POINT('Ctrl Pts',(39.4985856069267,-33.3349593710879,2.34799541531888));
#32578=CARTESIAN_POINT('Ctrl Pts',(38.8703983056154,-37.8336637277424,2.19099528796662));
#32579=CARTESIAN_POINT('Ctrl Pts',(34.7715877673847,-39.7913941019012,2.03399516061437));
#32580=CARTESIAN_POINT('Ctrl Pts',(30.8775965593863,-37.4526364914204,1.87699503326212));
#32581=CARTESIAN_POINT('Ctrl Pts',(30.6802042867265,-32.914574048659,1.71999490590986));
#32582=CARTESIAN_POINT('Ctrl Pts',(34.3564138261785,-30.2465374145616,1.56299477855761));
#32583=CARTESIAN_POINT('Ctrl Pts',(38.6097341605507,-31.8409675209513,1.40599465120535));
#32584=CARTESIAN_POINT('Ctrl Pts',(39.6261694334752,-36.2681500029269,1.2489945238531));
#32585=CARTESIAN_POINT('Ctrl Pts',(36.4942778376799,-39.5581346787212,1.09199439650085));
#32586=CARTESIAN_POINT('Ctrl Pts',(32.0224456319375,-38.7608678116187,0.934994269148595));
#32587=CARTESIAN_POINT('Ctrl Pts',(30.2206297689144,-34.5910506117954,0.777994141796339));
#32588=CARTESIAN_POINT('Ctrl Pts',(32.704491289799,-30.7882324000235,0.620994014444087));
#32589=CARTESIAN_POINT('Ctrl Pts',(37.2468174060219,-30.7615623188695,0.463993887091833));
#32590=CARTESIAN_POINT('Ctrl Pts',(39.7742801854456,-34.536716632844,0.306993759739581));
#32591=CARTESIAN_POINT('Ctrl Pts',(38.0208425645948,-38.7249309242138,0.149993632387326));
#32592=CARTESIAN_POINT('Ctrl Pts',(33.5581056824257,-39.5777559852671,-0.00700649496492666));
#32593=CARTESIAN_POINT('Ctrl Pts',(30.3892373827997,-36.3158028716181,-0.16400662231718));
#32594=CARTESIAN_POINT('Ctrl Pts',(31.0334355704763,-33.370922410012,-0.26867337388535));
#32595=CARTESIAN_POINT('Ctrl Pts',(31.9038714051976,-32.3528524834368,-0.321006749669435));
#32596=CARTESIAN_POINT('Ctrl Pts',(33.9957950511247,-38.756249785149,8.10700224988981));
#32597=CARTESIAN_POINT('Ctrl Pts',(32.7606638781546,-38.426046814806,8.05466887410573));
#32598=CARTESIAN_POINT('Ctrl Pts',(30.6617244103942,-36.4578802990271,7.95000212253756));
#32599=CARTESIAN_POINT('Ctrl Pts',(31.3907400550635,-32.1786916379746,7.79300199518531));
#32600=CARTESIAN_POINT('Ctrl Pts',(35.3622593055321,-30.4366625774945,7.63600186783305));
#32601=CARTESIAN_POINT('Ctrl Pts',(39.0059680720859,-32.7831124169518,7.4790017404808));
#32602=CARTESIAN_POINT('Ctrl Pts',(39.0589592913856,-37.1192003185169,7.32200161312853));
#32603=CARTESIAN_POINT('Ctrl Pts',(35.4715117112195,-39.554120602731,7.16500148577629));
#32604=CARTESIAN_POINT('Ctrl Pts',(31.4616180877658,-37.9057444599095,7.00800135842404));
#32605=CARTESIAN_POINT('Ctrl Pts',(30.6244451918799,-33.6515472373793,6.85100123107178));
#32606=CARTESIAN_POINT('Ctrl Pts',(33.7109637950579,-30.6066258939446,6.69400110371953));
#32607=CARTESIAN_POINT('Ctrl Pts',(37.9533290718052,-31.5012329431111,6.53700097636728));
#32608=CARTESIAN_POINT('Ctrl Pts',(39.5474379144414,-35.5332439578948,6.38000084901502));
#32609=CARTESIAN_POINT('Ctrl Pts',(37.0638045894695,-39.0870770983678,6.22300072166277));
#32610=CARTESIAN_POINT('Ctrl Pts',(32.729543334333,-38.9759954019356,6.06600059431052));
#32611=CARTESIAN_POINT('Ctrl Pts',(30.4312196493866,-35.2995973030108,5.90900046695826));
#32612=CARTESIAN_POINT('Ctrl Pts',(32.2297664783665,-31.3545490082375,5.752000339606));
#32613=CARTESIAN_POINT('Ctrl Pts',(36.5124076158656,-30.6784108060473,5.59500021225375));
#32614=CARTESIAN_POINT('Ctrl Pts',(39.4388586659392,-33.8774834831539,5.4380000849015));
#32615=CARTESIAN_POINT('Ctrl Pts',(38.3849424013594,-38.0831272963638,5.28099995754925));
#32616=CARTESIAN_POINT('Ctrl Pts',(34.2957158934656,-39.5241013808263,5.123999830197));
#32617=CARTESIAN_POINT('Ctrl Pts',(30.8380276599492,-36.9082703071214,4.96699970284474));
#32618=CARTESIAN_POINT('Ctrl Pts',(31.1124199720466,-32.581274965603,4.80999957549249));
#32619=CARTESIAN_POINT('Ctrl Pts',(34.8728425809651,-30.4231735548519,4.65299944814024));
#32620=CARTESIAN_POINT('Ctrl Pts',(38.7472884723895,-32.3691563314071,4.49599932078798));
#32621=CARTESIAN_POINT('Ctrl Pts',(39.2615048383014,-36.674241861831,4.33899919343573));
#32622=CARTESIAN_POINT('Ctrl Pts',(35.954388933901,-39.4780186542996,4.18199906608348));
#32623=CARTESIAN_POINT('Ctrl Pts',(31.7914633158823,-38.2663131584621,4.02499893873122));
#32624=CARTESIAN_POINT('Ctrl Pts',(30.5056633240975,-34.1256733184278,3.86799881137897));
#32625=CARTESIAN_POINT('Ctrl Pts',(33.2499781462058,-30.7690506010293,3.71099868402671));
#32626=CARTESIAN_POINT('Ctrl Pts',(37.5635543535394,-31.2063608006002,3.55399855667446));
#32627=CARTESIAN_POINT('Ctrl Pts',(39.5783667785835,-35.0454636628748,3.39699842932221));
#32628=CARTESIAN_POINT('Ctrl Pts',(37.4877137900394,-38.8437988263006,3.23999830196995));
#32629=CARTESIAN_POINT('Ctrl Pts',(33.1663039806949,-39.1953626988076,3.0829981746177));
#32630=CARTESIAN_POINT('Ctrl Pts',(30.4891869819735,-35.784904606173,2.92599804726545));
#32631=CARTESIAN_POINT('Ctrl Pts',(31.856959294467,-31.6706149922136,2.76899791991319));
#32632=CARTESIAN_POINT('Ctrl Pts',(36.0431263541924,-30.5418169177014,2.61199779256094));
#32633=CARTESIAN_POINT('Ctrl Pts',(39.2939120176749,-33.4107142575226,2.45499766520869));
#32634=CARTESIAN_POINT('Ctrl Pts',(38.6943055550796,-37.704739622131,2.29799753785643));
#32635=CARTESIAN_POINT('Ctrl Pts',(34.7819799118415,-39.5733985108324,2.14099741050418));
#32636=CARTESIAN_POINT('Ctrl Pts',(31.0651548682101,-37.3410481039379,1.98399728315193));
#32637=CARTESIAN_POINT('Ctrl Pts',(30.8767434149602,-33.0094553406639,1.82699715579967));
#32638=CARTESIAN_POINT('Ctrl Pts',(34.3856952723259,-30.4628072232849,1.66999702844742));
#32639=CARTESIAN_POINT('Ctrl Pts',(38.4455009300555,-31.9846950327841,1.51299690109516));
#32640=CARTESIAN_POINT('Ctrl Pts',(39.4156911220303,-36.2104525763381,1.35599677374291));
#32641=CARTESIAN_POINT('Ctrl Pts',(36.4262922006151,-39.3507517662898,1.19899664639066));
#32642=CARTESIAN_POINT('Ctrl Pts',(32.1579163760677,-38.5897584050265,1.04199651903841));
#32643=CARTESIAN_POINT('Ctrl Pts',(30.4380783060842,-34.6096567130058,0.884996391686151));
#32644=CARTESIAN_POINT('Ctrl Pts',(32.8089307843264,-30.9798565386092,0.727996264333898));
#32645=CARTESIAN_POINT('Ctrl Pts',(37.1445932353457,-30.9543998746739,0.570996136981644));
#32646=CARTESIAN_POINT('Ctrl Pts',(39.5570632317115,-34.5577947844858,0.413996009629391));
#32647=CARTESIAN_POINT('Ctrl Pts',(37.8834023235315,-38.5554565496905,0.256995882277137));
#32648=CARTESIAN_POINT('Ctrl Pts',(33.6237080097094,-39.3694803559713,0.0999957549248841));
#32649=CARTESIAN_POINT('Ctrl Pts',(30.5990147253931,-36.25593736721,-0.0570043724273687));
#32650=CARTESIAN_POINT('Ctrl Pts',(31.2139036219321,-33.4450410745538,-0.161671123995539));
#32651=CARTESIAN_POINT('Ctrl Pts',(32.0447369588746,-32.4732906012887,-0.214004499779624));
#32652=CARTESIAN_POINT('Ctrl Pts',(34.0436614793107,-38.5772044012455,8.21400449977962));
#32653=CARTESIAN_POINT('Ctrl Pts',(32.8674040627957,-38.2627408840732,8.16167112399554));
#32654=CARTESIAN_POINT('Ctrl Pts',(30.8685126334489,-36.3883889838178,8.05700437242737));
#32655=CARTESIAN_POINT('Ctrl Pts',(31.5627790219617,-32.3131721085722,7.90000424507511));
#32656=CARTESIAN_POINT('Ctrl Pts',(35.3449918552448,-30.6541785967763,7.74300411772285));
#32657=CARTESIAN_POINT('Ctrl Pts',(38.8150196175374,-32.8887825696523,7.58600399037061));
#32658=CARTESIAN_POINT('Ctrl Pts',(38.8654849576371,-37.0181865264902,7.42900386301835));
#32659=CARTESIAN_POINT('Ctrl Pts',(35.4490366362965,-39.3370439123355,7.2720037356661));
#32660=CARTESIAN_POINT('Ctrl Pts',(31.6302785827036,-37.7672392586828,7.11500360831385));
#32661=CARTESIAN_POINT('Ctrl Pts',(30.833010365982,-33.715822580173,6.95800348096159));
#32662=CARTESIAN_POINT('Ctrl Pts',(33.7724069885036,-30.8160404426151,6.80100335360934));
#32663=CARTESIAN_POINT('Ctrl Pts',(37.8125557027003,-31.6680051565476,6.64400322625708));
#32664=CARTESIAN_POINT('Ctrl Pts',(39.3306797610333,-35.5078263540035,6.48700309890484));
#32665=CARTESIAN_POINT('Ctrl Pts',(36.9654312899929,-38.892262501369,6.33000297155257));
#32666=CARTESIAN_POINT('Ctrl Pts',(32.8377669106638,-38.7864756245362,6.17300284420034));
#32667=CARTESIAN_POINT('Ctrl Pts',(30.6489951112531,-35.2853166994296,6.01600271684807));
#32668=CARTESIAN_POINT('Ctrl Pts',(32.3618124158715,-31.5283130573969,5.85900258949582));
#32669=CARTESIAN_POINT('Ctrl Pts',(36.4403172018384,-30.8844036554483,5.70200246214356));
#32670=CARTESIAN_POINT('Ctrl Pts',(39.2272760504595,-33.9309893499606,5.54500233479132));
#32671=CARTESIAN_POINT('Ctrl Pts',(38.2235957533972,-37.9361669657214,5.38800220743906));
#32672=CARTESIAN_POINT('Ctrl Pts',(34.3292862962461,-39.3084555865154,5.23100208008681));
#32673=CARTESIAN_POINT('Ctrl Pts',(31.0364122131721,-36.8173107039871,5.07400195273455));
#32674=CARTESIAN_POINT('Ctrl Pts',(31.2977253426618,-32.6965659012732,4.9170018253823));
#32675=CARTESIAN_POINT('Ctrl Pts',(34.8789036658794,-30.6413325418211,4.76000169803005));
#32676=CARTESIAN_POINT('Ctrl Pts',(38.5686702383762,-32.4945581128583,4.60300157067779));
#32677=CARTESIAN_POINT('Ctrl Pts',(39.0583759695033,-36.5944374574263,4.44600144332554));
#32678=CARTESIAN_POINT('Ctrl Pts',(35.9088970356414,-39.2645694390062,4.28900131597328));
#32679=CARTESIAN_POINT('Ctrl Pts',(31.9444014097886,-38.1106210914121,4.13200118862103));
#32680=CARTESIAN_POINT('Ctrl Pts',(30.7198903541289,-34.1673489697591,3.97500106126878));
#32681=CARTESIAN_POINT('Ctrl Pts',(33.333394679337,-30.9707230144056,3.81800093391652));
#32682=CARTESIAN_POINT('Ctrl Pts',(37.4413599842507,-31.3871883881407,3.66100080656427));
#32683=CARTESIAN_POINT('Ctrl Pts',(39.3601343700882,-35.0432965921423,3.50400067921202));
#32684=CARTESIAN_POINT('Ctrl Pts',(37.36913443668,-38.6605803302294,3.34700055185977));
#32685=CARTESIAN_POINT('Ctrl Pts',(33.2537089261905,-38.9953865609073,3.19000042450751));
#32686=CARTESIAN_POINT('Ctrl Pts',(30.7041993732481,-35.7474913470507,3.03300029715526));
#32687=CARTESIAN_POINT('Ctrl Pts',(32.006775457378,-31.8293134417253,2.876000169803));
#32688=CARTESIAN_POINT('Ctrl Pts',(35.9934046984909,-30.7543206507168,2.71900004245075));
#32689=CARTESIAN_POINT('Ctrl Pts',(39.0892384284232,-33.4864691439573,2.5619999150985));
#32690=CARTESIAN_POINT('Ctrl Pts',(38.5182128045439,-37.5758155165195,2.40499978774624));
#32691=CARTESIAN_POINT('Ctrl Pts',(34.7923720562983,-39.3554029197635,2.24799966039399));
#32692=CARTESIAN_POINT('Ctrl Pts',(31.2527131770338,-37.2294597164554,2.09099953304174));
#32693=CARTESIAN_POINT('Ctrl Pts',(31.073282543194,-33.1043366326688,1.93399940568948));
#32694=CARTESIAN_POINT('Ctrl Pts',(34.4149767184733,-30.6790770320082,1.77699927833723));
#32695=CARTESIAN_POINT('Ctrl Pts',(38.2812676995604,-32.1284225446167,1.61999915098497));
#32696=CARTESIAN_POINT('Ctrl Pts',(39.2052128105854,-36.1527551497494,1.46299902363272));
#32697=CARTESIAN_POINT('Ctrl Pts',(36.3583065635504,-39.1433688538583,1.30599889628047));
#32698=CARTESIAN_POINT('Ctrl Pts',(32.2933871201978,-38.4186489984343,1.14899876892821));
#32699=CARTESIAN_POINT('Ctrl Pts',(30.655526843254,-34.6282628142162,0.991998641575962));
#32700=CARTESIAN_POINT('Ctrl Pts',(32.9133702788538,-31.1714806771949,0.834998514223709));
#32701=CARTESIAN_POINT('Ctrl Pts',(37.0423690646695,-31.1472374304784,0.677998386871454));
#32702=CARTESIAN_POINT('Ctrl Pts',(39.3398462779774,-34.5788729361276,0.520998259519202));
#32703=CARTESIAN_POINT('Ctrl Pts',(37.7459620824681,-38.385982175167,0.363998132166948));
#32704=CARTESIAN_POINT('Ctrl Pts',(33.6893103369932,-39.1612047266757,0.206998004814695));
#32705=CARTESIAN_POINT('Ctrl Pts',(30.8087920679866,-36.1960718628018,0.0499978774624421));
#32706=CARTESIAN_POINT('Ctrl Pts',(31.3943716733879,-33.5191597390956,-0.0546688741057282));
#32707=CARTESIAN_POINT('Ctrl Pts',(32.1856025125517,-32.5937287191406,-0.107002249889813));
#32708=CARTESIAN_POINT('Ctrl Pts',(34.0915279074966,-38.398159017342,8.32100674966943));
#32709=CARTESIAN_POINT('Ctrl Pts',(32.9741442474368,-38.0994349533405,8.26867337388535));
#32710=CARTESIAN_POINT('Ctrl Pts',(31.0753008565035,-36.3188976686085,8.16400662231718));
#32711=CARTESIAN_POINT('Ctrl Pts',(31.73481798886,-32.4476525791699,8.00700649496493));
#32712=CARTESIAN_POINT('Ctrl Pts',(35.3277244049576,-30.8716946160581,7.85000636761267));
#32713=CARTESIAN_POINT('Ctrl Pts',(38.6240711629891,-32.9944527223528,7.69300624026043));
#32714=CARTESIAN_POINT('Ctrl Pts',(38.6720106238885,-36.9171727344635,7.53600611290815));
#32715=CARTESIAN_POINT('Ctrl Pts',(35.4265615613737,-39.1199672219399,7.37900598555592));
#32716=CARTESIAN_POINT('Ctrl Pts',(31.7989390776415,-37.628734057456,7.22200585820365));
#32717=CARTESIAN_POINT('Ctrl Pts',(31.0415755400842,-33.7800979229667,7.06500573085141));
#32718=CARTESIAN_POINT('Ctrl Pts',(33.8338501819494,-31.0254549912856,6.90800560349915));
#32719=CARTESIAN_POINT('Ctrl Pts',(37.6717823335954,-31.8347773699841,6.75100547614689));
#32720=CARTESIAN_POINT('Ctrl Pts',(39.1139216076251,-35.4824087501123,6.59400534879465));
#32721=CARTESIAN_POINT('Ctrl Pts',(36.8670579905162,-38.6974479043702,6.43700522144239));
#32722=CARTESIAN_POINT('Ctrl Pts',(32.9459904869947,-38.5969558471367,6.28000509409014));
#32723=CARTESIAN_POINT('Ctrl Pts',(30.8667705731195,-35.2710360958482,6.12300496673788));
#32724=CARTESIAN_POINT('Ctrl Pts',(32.4938583533767,-31.7020771065563,5.96600483938563));
#32725=CARTESIAN_POINT('Ctrl Pts',(36.3682267878111,-31.0903965048492,5.80900471203338));
#32726=CARTESIAN_POINT('Ctrl Pts',(39.0156934349799,-33.9844952167673,5.65200458468112));
#32727=CARTESIAN_POINT('Ctrl Pts',(38.0622491054349,-37.789206635079,5.49500445732887));
#32728=CARTESIAN_POINT('Ctrl Pts',(34.3628566990267,-39.0928097922045,5.33800432997662));
#32729=CARTESIAN_POINT('Ctrl Pts',(31.234796766395,-36.7263511008529,5.18100420262436));
#32730=CARTESIAN_POINT('Ctrl Pts',(31.4830307132771,-32.8118568369433,5.02400407527211));
#32731=CARTESIAN_POINT('Ctrl Pts',(34.8849647507938,-30.8594915287904,4.86700394791986));
#32732=CARTESIAN_POINT('Ctrl Pts',(38.3900520043628,-32.6199598943095,4.7100038205676));
#32733=CARTESIAN_POINT('Ctrl Pts',(38.8552471007052,-36.5146330530217,4.55300369321535));
#32734=CARTESIAN_POINT('Ctrl Pts',(35.8634051373818,-39.0511202237127,4.39600356586309));
#32735=CARTESIAN_POINT('Ctrl Pts',(32.0973395036949,-37.9549290243621,4.23900343851084));
#32736=CARTESIAN_POINT('Ctrl Pts',(30.9341173841603,-34.2090246210904,4.08200331115859));
#32737=CARTESIAN_POINT('Ctrl Pts',(33.4168112124683,-31.1723954277819,3.92500318380634));
#32738=CARTESIAN_POINT('Ctrl Pts',(37.319165614962,-31.5680159756812,3.76800305645408));
#32739=CARTESIAN_POINT('Ctrl Pts',(39.141901961593,-35.0411295214099,3.61100292910183));
#32740=CARTESIAN_POINT('Ctrl Pts',(37.2505550833205,-38.4773618341581,3.45400280174957));
#32741=CARTESIAN_POINT('Ctrl Pts',(33.3411138716861,-38.7954104230071,3.29700267439732));
#32742=CARTESIAN_POINT('Ctrl Pts',(30.9192117645227,-35.7100780879284,3.14000254704507));
#32743=CARTESIAN_POINT('Ctrl Pts',(32.1565916202891,-31.988011891237,2.98300241969282));
#32744=CARTESIAN_POINT('Ctrl Pts',(35.9436830427893,-30.9668243837322,2.82600229234056));
#32745=CARTESIAN_POINT('Ctrl Pts',(38.8845648391714,-33.5622240303919,2.66900216498831));
#32746=CARTESIAN_POINT('Ctrl Pts',(38.3421200540082,-37.4468914109081,2.51200203763606));
#32747=CARTESIAN_POINT('Ctrl Pts',(34.802764200755,-39.1374073286946,2.3550019102838));
#32748=CARTESIAN_POINT('Ctrl Pts',(31.4402714858577,-37.1178713289729,2.19800178293155));
#32749=CARTESIAN_POINT('Ctrl Pts',(31.2698216714276,-33.1992179246737,2.04100165557929));
#32750=CARTESIAN_POINT('Ctrl Pts',(34.4442581646208,-30.8953468407316,1.88400152822704));
#32751=CARTESIAN_POINT('Ctrl Pts',(38.1170344690652,-32.2721500564494,1.72700140087478));
#32752=CARTESIAN_POINT('Ctrl Pts',(38.9947344991405,-36.0950577231607,1.57000127352253));
#32753=CARTESIAN_POINT('Ctrl Pts',(36.2903209264856,-38.9359859414268,1.41300114617028));
#32754=CARTESIAN_POINT('Ctrl Pts',(32.428857864328,-38.247539591842,1.25600101881803));
#32755=CARTESIAN_POINT('Ctrl Pts',(30.8729753804238,-34.6468689154266,1.09900089146577));
#32756=CARTESIAN_POINT('Ctrl Pts',(33.0178097733811,-31.3631048157807,0.942000764113519));
#32757=CARTESIAN_POINT('Ctrl Pts',(36.9401448939934,-31.3400749862829,0.785000636761266));
#32758=CARTESIAN_POINT('Ctrl Pts',(39.1226293242432,-34.5999510877694,0.628000509409013));
#32759=CARTESIAN_POINT('Ctrl Pts',(37.6085218414048,-38.2165078006437,0.471000382056759));
#32760=CARTESIAN_POINT('Ctrl Pts',(33.754912664277,-38.9529290973799,0.314000254704506));
#32761=CARTESIAN_POINT('Ctrl Pts',(31.0185694105801,-36.1362063583937,0.157000127352253));
#32762=CARTESIAN_POINT('Ctrl Pts',(31.5748397248436,-33.5932784036374,0.0523333757840826));
#32763=CARTESIAN_POINT('Ctrl Pts',(32.3264680662287,-32.7141668369925,-2.22044604925031E-15));
#32764=CARTESIAN_POINT('Ctrl Pts',(32.3264680662287,-32.7141668369925,-2.27595720048157E-15));
#32765=CARTESIAN_POINT('Ctrl Pts',(32.2493253090815,-32.7912797983002,-2.16394166852401E-15));
#32766=CARTESIAN_POINT('Ctrl Pts',(32.1762949026186,-32.8720149145437,3.46363794187806E-16));
#32767=CARTESIAN_POINT('Ctrl Pts',(32.1073691591848,-32.9559536860909,1.66533453693773E-16));
#32768=CARTESIAN_POINT('Ctrl Pts',(32.0366835341849,-33.0420356669728,-1.78884963425382E-17));
#32769=CARTESIAN_POINT('Ctrl Pts',(31.9703144812951,-33.1314874423946,-2.24888209125886E-15));
#32770=CARTESIAN_POINT('Ctrl Pts',(31.9082835820817,-33.2239037683368,-2.33146835171283E-15));
#32771=CARTESIAN_POINT('Ctrl Pts',(31.8449616802408,-33.3182434860262,-2.41577341812641E-15));
#32772=CARTESIAN_POINT('Ctrl Pts',(31.7861599686898,-33.4156730215343,-2.34515801197777E-15));
#32773=CARTESIAN_POINT('Ctrl Pts',(31.7319381963941,-33.5158007480848,-2.77555756156289E-15));
#32774=CARTESIAN_POINT('Ctrl Pts',(31.6801489223982,-33.611436542441,-3.18664851741706E-15));
#32775=CARTESIAN_POINT('Ctrl Pts',(31.6325378836028,-33.7095346984804,-3.69832300465041E-15));
#32776=CARTESIAN_POINT('Ctrl Pts',(31.5891926568309,-33.8097785742014,-3.99680288865056E-15));
#32777=CARTESIAN_POINT('Ctrl Pts',(31.5821541452564,-33.8260564375806,-4.04527083482939E-15));
#32778=CARTESIAN_POINT('Ctrl Pts',(31.5752281942475,-33.8423909194022,-5.19848407519141E-15));
#32779=CARTESIAN_POINT('Ctrl Pts',(31.568415272417,-33.8587807065962,-5.21804821573824E-15));
#32780=CARTESIAN_POINT('Ctrl Pts',(31.561906348996,-33.8744391674425,-5.23673938757109E-15));
#32781=CARTESIAN_POINT('Ctrl Pts',(31.5555036120846,-33.8901409126424,-5.57046258471252E-15));
#32782=CARTESIAN_POINT('Ctrl Pts',(31.5492092706946,-33.9058793019477,-5.49560397189452E-15));
#32783=CARTESIAN_POINT('Ctrl Pts',(31.5058237133564,-34.0143606742329,-4.97961946494936E-15));
#32784=CARTESIAN_POINT('Ctrl Pts',(31.4675520206245,-34.1246590298884,-6.38605598306829E-15));
#32785=CARTESIAN_POINT('Ctrl Pts',(31.4344228151864,-34.2363425690307,-5.19029264012261E-15));
#32786=CARTESIAN_POINT('Ctrl Pts',(31.4008590997118,-34.3494909069217,-3.9788461207494E-15));
#32787=CARTESIAN_POINT('Ctrl Pts',(31.3725732548101,-34.4640617531158,-1.67269218670119E-15));
#32788=CARTESIAN_POINT('Ctrl Pts',(31.3496376837557,-34.5796386183165,-1.85962356624714E-15));
#32789=CARTESIAN_POINT('Ctrl Pts',(31.3256626239872,-34.7004536721242,-2.05502707229468E-15));
#32790=CARTESIAN_POINT('Ctrl Pts',(31.3075330179638,-34.8223688186784,-6.90474885500916E-16));
#32791=CARTESIAN_POINT('Ctrl Pts',(31.2953872940185,-34.9449317101526,1.11022302462516E-16));
#32792=CARTESIAN_POINT('Ctrl Pts',(31.2862780010595,-35.0368538787582,7.12145193435089E-16));
#32793=CARTESIAN_POINT('Ctrl Pts',(31.2805357649583,-35.1291410005731,-7.33619512718545E-16));
#32794=CARTESIAN_POINT('Ctrl Pts',(31.2782421142109,-35.2216056948398,-3.88578058618805E-16));
#32795=CARTESIAN_POINT('Ctrl Pts',(31.2776945327762,-35.2436805246709,-3.0620357564075E-16));
#32796=CARTESIAN_POINT('Ctrl Pts',(31.2773436607928,-35.2657700018002,-4.90649572448904E-16));
#32797=CARTESIAN_POINT('Ctrl Pts',(31.2771907100455,-35.287842514156,-5.27355936696949E-16));
#32798=CARTESIAN_POINT('Ctrl Pts',(31.2763557493203,-35.4083367336975,-7.27736602069211E-16));
#32799=CARTESIAN_POINT('Ctrl Pts',(31.2814089690861,-35.5284761575602,-1.32546033095374E-15));
#32800=CARTESIAN_POINT('Ctrl Pts',(31.2924193361456,-35.6478347566642,-1.0547118733939E-15));
#32801=CARTESIAN_POINT('Ctrl Pts',(31.3033590399359,-35.7664273260093,-7.85701048289603E-16));
#32802=CARTESIAN_POINT('Ctrl Pts',(31.3201794237171,-35.8842499373544,-3.19095490877261E-16));
#32803=CARTESIAN_POINT('Ctrl Pts',(31.3429975699143,-36.0008975571309,1.94289029309402E-16));
#32804=CARTESIAN_POINT('Ctrl Pts',(31.3458712257766,-36.0155878441288,2.58943292776536E-16));
#32805=CARTESIAN_POINT('Ctrl Pts',(31.3488400749734,-36.030259502248,-2.41414676176044E-15));
#32806=CARTESIAN_POINT('Ctrl Pts',(31.3519044105546,-36.0449117261916,-2.44249065417534E-15));
#32807=CARTESIAN_POINT('Ctrl Pts',(31.375814852164,-36.1592403092631,-2.71916393553799E-15));
#32808=CARTESIAN_POINT('Ctrl Pts',(31.4055345217229,-36.272386206175,5.65793814005205E-16));
#32809=CARTESIAN_POINT('Ctrl Pts',(31.4407572695548,-36.384082920097,4.44089209850063E-16));
#32810=CARTESIAN_POINT('Ctrl Pts',(31.4627225424769,-36.453738155898,3.68192949317207E-16));
#32811=CARTESIAN_POINT('Ctrl Pts',(31.4868289857256,-36.52282973013,-1.13814971295829E-15));
#32812=CARTESIAN_POINT('Ctrl Pts',(31.513012205469,-36.5912908274846,-1.69309011255336E-15));
#32813=CARTESIAN_POINT('Ctrl Pts',(31.5219624105717,-36.6146928715758,-1.88278528544959E-15));
#32814=CARTESIAN_POINT('Ctrl Pts',(31.531155343526,-36.6380212260425,4.03667916851762E-15));
#32815=CARTESIAN_POINT('Ctrl Pts',(31.5405886194687,-36.6612731534534,4.32986979603811E-15));
#32816=CARTESIAN_POINT('Ctrl Pts',(31.5473370498667,-36.6779072490427,4.53961416853196E-15));
#32817=CARTESIAN_POINT('Ctrl Pts',(31.5542090296369,-36.6945033501966,3.07759665647771E-15));
#32818=CARTESIAN_POINT('Ctrl Pts',(31.561196617679,-36.7110441569158,2.94209101525666E-15));
#32819=CARTESIAN_POINT('Ctrl Pts',(31.6071179522689,-36.8197477489354,2.0515691568155E-15));
#32820=CARTESIAN_POINT('Ctrl Pts',(31.6580923235038,-36.9262249725842,4.21341387307547E-15));
#32821=CARTESIAN_POINT('Ctrl Pts',(31.7137612878297,-37.0302214764794,3.42781358853017E-15));
#32822=CARTESIAN_POINT('Ctrl Pts',(31.7713455134326,-37.1377959250922,2.61518514166327E-15));
#32823=CARTESIAN_POINT('Ctrl Pts',(31.8339530898433,-37.2427167108642,9.07249106506457E-16));
#32824=CARTESIAN_POINT('Ctrl Pts',(31.9012426720394,-37.3446949826671,6.80011602582908E-16));
#32825=CARTESIAN_POINT('Ctrl Pts',(31.9691654564611,-37.4476328810058,4.50635769240332E-16));
#32826=CARTESIAN_POINT('Ctrl Pts',(32.0418592122967,-37.5475733704053,-1.57902851375934E-15));
#32827=CARTESIAN_POINT('Ctrl Pts',(32.1190233809196,-37.6442010945393,-1.81799020282369E-15));
#32828=CARTESIAN_POINT('Ctrl Pts',(32.1734366012044,-37.712339269715,-1.98649684598102E-15));
#32829=CARTESIAN_POINT('Ctrl Pts',(32.2300738179544,-37.7788298007494,1.23701449661782E-16));
#32830=CARTESIAN_POINT('Ctrl Pts',(32.2888426956766,-37.8435536257978,-3.88578058618805E-16));
#32831=CARTESIAN_POINT('Ctrl Pts',(32.3150744390812,-37.8724433857632,-6.17236238483284E-16));
#32832=CARTESIAN_POINT('Ctrl Pts',(32.3417310110036,-37.9009810526196,1.30430196317008E-16));
#32833=CARTESIAN_POINT('Ctrl Pts',(32.3688048104485,-37.9291554653168,-2.77555756156289E-17));
#32834=CARTESIAN_POINT('Ctrl Pts',(32.3804263297313,-37.9412494265322,-9.56573491554205E-17));
#32835=CARTESIAN_POINT('Ctrl Pts',(32.392123309834,-37.9532749179279,-6.28475541027777E-16));
#32836=CARTESIAN_POINT('Ctrl Pts',(32.4038886430803,-37.9652246721857,-5.96744875736022E-16));
#32837=CARTESIAN_POINT('Ctrl Pts',(32.4923309120516,-38.05505326931,-3.5821937240873E-16));
#32838=CARTESIAN_POINT('Ctrl Pts',(32.5847325176906,-38.1407092470896,2.11600168392725E-15));
#32839=CARTESIAN_POINT('Ctrl Pts',(32.6807647145451,-38.221874449736,1.96370697480575E-15));
#32840=CARTESIAN_POINT('Ctrl Pts',(32.7628051861864,-38.2912140225467,1.8336013417573E-15));
#32841=CARTESIAN_POINT('Ctrl Pts',(32.8474963866317,-38.3572760203649,1.20960812321559E-15));
#32842=CARTESIAN_POINT('Ctrl Pts',(32.9346575664231,-38.4198445069104,5.62050406216485E-16));
#32843=CARTESIAN_POINT('Ctrl Pts',(32.973768957553,-38.4479205443796,2.71475138541893E-16));
#32844=CARTESIAN_POINT('Ctrl Pts',(33.0133779626213,-38.4752928979382,3.47992543175087E-15));
#32845=CARTESIAN_POINT('Ctrl Pts',(33.0534694930906,-38.5019407001488,3.78169717762944E-15));
#32846=CARTESIAN_POINT('Ctrl Pts',(33.0807047104967,-38.5200432439556,3.98669855846499E-15));
#32847=CARTESIAN_POINT('Ctrl Pts',(33.108168250427,-38.5378147929466,1.27528005472796E-15));
#32848=CARTESIAN_POINT('Ctrl Pts',(33.1358254185318,-38.5552300293176,1.47104550762833E-15));
#32849=CARTESIAN_POINT('Ctrl Pts',(33.2426299049644,-38.6224829515854,2.22703862229035E-15));
#32850=CARTESIAN_POINT('Ctrl Pts',(33.3523811032195,-38.6844690524263,5.56024339803508E-15));
#32851=CARTESIAN_POINT('Ctrl Pts',(33.4647770313827,-38.7408546683214,3.76781938982163E-15));
#32852=CARTESIAN_POINT('Ctrl Pts',(33.5668706528472,-38.7920719305417,2.13969049592827E-15));
#32853=CARTESIAN_POINT('Ctrl Pts',(33.6711471781243,-38.8386683831236,1.86420798495096E-15));
#32854=CARTESIAN_POINT('Ctrl Pts',(33.7774036389012,-38.880364855251,2.14498557804532E-15));
#32855=CARTESIAN_POINT('Ctrl Pts',(33.8328341927383,-38.9021165541705,2.26717202503918E-15));
#32856=CARTESIAN_POINT('Ctrl Pts',(33.8888038950002,-38.9225342787199,1.50877474080585E-16));
#32857=CARTESIAN_POINT('Ctrl Pts',(33.94526862329,-38.9416301412996,1.94289029309402E-16));
#32858=CARTESIAN_POINT('Ctrl Pts',(31.4846885160394,-34.9971888045819,7.11258330249198));
#32859=CARTESIAN_POINT('Ctrl Pts',(31.4819573643756,-34.6461972356202,7.09672411194512));
#32860=CARTESIAN_POINT('Ctrl Pts',(31.5304047798457,-34.2959415119622,7.08086492139826));
#32861=CARTESIAN_POINT('Ctrl Pts',(31.6331819033213,-33.9624301234347,7.0650057308514));
#32862=CARTESIAN_POINT('Ctrl Pts',(31.9723337540393,-32.8618836124063,7.01267235506732));
#32863=CARTESIAN_POINT('Ctrl Pts',(32.9030919679943,-31.943669301846,6.96033897928324));
#32864=CARTESIAN_POINT('Ctrl Pts',(34.0081264335795,-31.6194492096822,6.90800560349915));
#32865=CARTESIAN_POINT('Ctrl Pts',(35.1131608991647,-31.2952291175184,6.85567222771506));
#32866=CARTESIAN_POINT('Ctrl Pts',(36.3924716163801,-31.5650032437512,6.80333885193098));
#32867=CARTESIAN_POINT('Ctrl Pts',(37.2724835206594,-32.3078288702224,6.75100547614689));
#32868=CARTESIAN_POINT('Ctrl Pts',(38.1524954249387,-33.0506544966935,6.69867210036281));
#32869=CARTESIAN_POINT('Ctrl Pts',(38.6332085162819,-34.2665316234029,6.64633872457873));
#32870=CARTESIAN_POINT('Ctrl Pts',(38.4990877924354,-35.4103100458006,6.59400534879464));
#32871=CARTESIAN_POINT('Ctrl Pts',(38.3649670685888,-36.5540884681983,6.54167197301056));
#32872=CARTESIAN_POINT('Ctrl Pts',(37.6160125295525,-37.6257681862843,6.48933859722647));
#32873=CARTESIAN_POINT('Ctrl Pts',(36.5880240094475,-38.1448593691216,6.43700522144239));
#32874=CARTESIAN_POINT('Ctrl Pts',(35.5600354893424,-38.663950551959,6.3846718456583));
#32875=CARTESIAN_POINT('Ctrl Pts',(34.2530129881685,-38.6304531995479,6.33233846987422));
#32876=CARTESIAN_POINT('Ctrl Pts',(33.2529650852691,-38.0593845647942,6.28000509409014));
#32877=CARTESIAN_POINT('Ctrl Pts',(32.2529171823696,-37.4883159300405,6.22767171830605));
#32878=CARTESIAN_POINT('Ctrl Pts',(31.5598438777445,-36.3796760129444,6.17533834252196));
#32879=CARTESIAN_POINT('Ctrl Pts',(31.4844885221415,-35.230529556181,6.12300496673788));
#32880=CARTESIAN_POINT('Ctrl Pts',(31.4794864356562,-35.1542492451791,6.11953107865591));
#32881=CARTESIAN_POINT('Ctrl Pts',(31.4772062002897,-35.0777904501775,6.11605719057394));
#32882=CARTESIAN_POINT('Ctrl Pts',(31.4775766908735,-35.0013091813966,6.11258330249198));
#32883=CARTESIAN_POINT('Origin',(-35.,35.,10.2084234471775));
#32884=CARTESIAN_POINT('Ctrl Pts',(-39.0784090602678,35.0020440536088,7.70842344717747));
#32885=CARTESIAN_POINT('Ctrl Pts',(-39.0792531838394,35.133112279499,7.70328437820512));
#32886=CARTESIAN_POINT('Ctrl Pts',(-39.0145240110799,36.5980970201662,7.64581193344869));
#32887=CARTESIAN_POINT('Ctrl Pts',(-37.2468179015868,39.238437726829,7.53600611290815));
#32888=CARTESIAN_POINT('Ctrl Pts',(-32.7044909023729,39.2117683922069,7.37900598555592));
#32889=CARTESIAN_POINT('Ctrl Pts',(-30.2206292307696,35.4089492839864,7.22200585820365));
#32890=CARTESIAN_POINT('Ctrl Pts',(-32.0224452414743,31.2391318114334,7.0650057308514));
#32891=CARTESIAN_POINT('Ctrl Pts',(-36.4942780330333,30.4418647129305,6.90800560349915));
#32892=CARTESIAN_POINT('Ctrl Pts',(-38.8653529438983,32.9326279141667,6.7891448422745));
#32893=CARTESIAN_POINT('Ctrl Pts',(-39.0751757451768,34.6330161300415,6.72261745683394));
#32894=CARTESIAN_POINT('Ctrl Pts',(-39.0721136942453,34.9965451882256,6.70842344717746));
#32895=CARTESIAN_POINT('Ctrl Pts',(-39.0691248821302,34.9959228837483,7.79157655282255));
#32896=CARTESIAN_POINT('Ctrl Pts',(-39.0629617588157,35.8984240805364,7.75638428364687));
#32897=CARTESIAN_POINT('Ctrl Pts',(-38.3270254278953,38.1550448362135,7.6688586386871));
#32898=CARTESIAN_POINT('Ctrl Pts',(-34.6204731393245,39.7808563212243,7.52899961794324));
#32899=CARTESIAN_POINT('Ctrl Pts',(-30.8030827008644,37.3225569109026,7.37199949059099));
#32900=CARTESIAN_POINT('Ctrl Pts',(-30.7475658132336,32.7797862032913,7.21499936323873));
#32901=CARTESIAN_POINT('Ctrl Pts',(-34.5060130464714,30.2288015790917,7.05799923588648));
#32902=CARTESIAN_POINT('Ctrl Pts',(-38.2826807551488,31.7813043056651,6.91685829908108));
#32903=CARTESIAN_POINT('Ctrl Pts',(-39.0636920303636,34.0684206251935,6.82805073805977));
#32904=CARTESIAN_POINT('Ctrl Pts',(-39.070966199943,35.0032555604945,6.79157655282255));
#32905=CARTESIAN_POINT('Ctrl Pts',(-32.3264680662287,37.2858331630075,8.));
#32906=CARTESIAN_POINT('Ctrl Pts',(-31.5748397248436,36.4067215963625,7.94766662421592));
#32907=CARTESIAN_POINT('Ctrl Pts',(-31.0185734566188,33.863789346735,7.84299987264775));
#32908=CARTESIAN_POINT('Ctrl Pts',(-33.7549107807148,31.0470722659105,7.68599974529549));
#32909=CARTESIAN_POINT('Ctrl Pts',(-37.6085229887763,31.7834906538058,7.52899961794324));
#32910=CARTESIAN_POINT('Ctrl Pts',(-39.122629437071,35.4000496587684,7.37199949059099));
#32911=CARTESIAN_POINT('Ctrl Pts',(-36.9401453219176,38.6599250531781,7.21499936323873));
#32912=CARTESIAN_POINT('Ctrl Pts',(-33.0178094388356,38.6368958683166,7.05799923588648));
#32913=CARTESIAN_POINT('Ctrl Pts',(-30.8729749157314,35.3531309945801,6.90099910853423));
#32914=CARTESIAN_POINT('Ctrl Pts',(-32.4288575271599,31.7524600826604,6.74399898118197));
#32915=CARTESIAN_POINT('Ctrl Pts',(-36.2903210951748,31.0640135332596,6.58699885382972));
#32916=CARTESIAN_POINT('Ctrl Pts',(-38.9947349861635,33.9049421642868,6.42999872647747));
#32917=CARTESIAN_POINT('Ctrl Pts',(-38.1170348549754,37.7278502673058,6.27299859912521));
#32918=CARTESIAN_POINT('Ctrl Pts',(-34.4442580951562,39.1046536709688,6.11599847177296));
#32919=CARTESIAN_POINT('Ctrl Pts',(-31.2698212127753,36.8007822935419,5.95899834442071));
#32920=CARTESIAN_POINT('Ctrl Pts',(-31.4402710474498,32.8821284121656,5.80199821706844));
#32921=CARTESIAN_POINT('Ctrl Pts',(-34.8027641765881,30.8625921610582,5.6449980897162));
#32922=CARTESIAN_POINT('Ctrl Pts',(-38.3421204653421,32.553108288411,5.48799796236394));
#32923=CARTESIAN_POINT('Ctrl Pts',(-38.884565317352,36.4377761463179,5.33099783501169));
#32924=CARTESIAN_POINT('Ctrl Pts',(-35.9436831589371,39.0331761128571,5.17399770765944));
#32925=CARTESIAN_POINT('Ctrl Pts',(-32.1565912702954,38.0119884794394,5.01699758030718));
#32926=CARTESIAN_POINT('Ctrl Pts',(-30.9192112622106,34.2899218247053,4.85999745295493));
#32927=CARTESIAN_POINT('Ctrl Pts',(-33.3411136674927,31.2045891097909,4.70299732560268));
#32928=CARTESIAN_POINT('Ctrl Pts',(-37.2505553603438,31.522637737819,4.54599719825043));
#32929=CARTESIAN_POINT('Ctrl Pts',(-39.1419024714255,34.9588704735221,4.38899707089817));
#32930=CARTESIAN_POINT('Ctrl Pts',(-37.3191659004311,38.4319844467691,4.23199694354592));
#32931=CARTESIAN_POINT('Ctrl Pts',(-33.4168110175916,38.8276050433616,4.07499681619367));
#32932=CARTESIAN_POINT('Ctrl Pts',(-30.9341168836852,35.7909754762728,3.91799668884141));
#32933=CARTESIAN_POINT('Ctrl Pts',(-32.0973391464029,32.0450706119108,3.76099656148916));
#32934=CARTESIAN_POINT('Ctrl Pts',(-35.8634052436587,30.9488792776308,3.6039964341369));
#32935=CARTESIAN_POINT('Ctrl Pts',(-38.8552475752543,33.4853667605377,3.44699630678465));
#32936=CARTESIAN_POINT('Ctrl Pts',(-38.390052421646,37.3800403986573,3.2899961794324));
#32937=CARTESIAN_POINT('Ctrl Pts',(-34.8849647366394,39.1405089808617,3.13299605208014));
#32938=CARTESIAN_POINT('Ctrl Pts',(-31.4830302803583,37.1881434324151,2.97599592472789));
#32939=CARTESIAN_POINT('Ctrl Pts',(-31.2347963029507,33.2736486866154,2.81899579737564));
#32940=CARTESIAN_POINT('Ctrl Pts',(-34.3628566205626,30.9071897040694,2.66199567002338));
#32941=CARTESIAN_POINT('Ctrl Pts',(-38.0622494824414,32.2107930214718,2.50499554267113));
#32942=CARTESIAN_POINT('Ctrl Pts',(-39.0156939291453,36.0155049084671,2.34799541531888));
#32943=CARTESIAN_POINT('Ctrl Pts',(-36.368226956474,38.9096039759392,2.19099528796663));
#32944=CARTESIAN_POINT('Ctrl Pts',(-32.4938580444355,38.2979233002502,2.03399516061437));
#32945=CARTESIAN_POINT('Ctrl Pts',(-30.8667700651969,34.7289638691476,1.87699503326212));
#32946=CARTESIAN_POINT('Ctrl Pts',(-32.9459902326247,31.4030437132317,1.71999490590986));
#32947=CARTESIAN_POINT('Ctrl Pts',(-36.8670582231188,31.3025516345889,1.56299477855761));
#32948=CARTESIAN_POINT('Ctrl Pts',(-39.1139221090429,34.517591201676,1.40599465120536));
#32949=CARTESIAN_POINT('Ctrl Pts',(-37.6717826711976,38.1652229986406,1.2489945238531));
#32950=CARTESIAN_POINT('Ctrl Pts',(-33.8338500234071,38.9745455371789,1.09199439650085));
#32951=CARTESIAN_POINT('Ctrl Pts',(-31.041575077848,36.2199021542904,0.934994269148598));
#32952=CARTESIAN_POINT('Ctrl Pts',(-31.7989386437116,32.3712657534865,0.777994141796342));
#32953=CARTESIAN_POINT('Ctrl Pts',(-35.4265616731752,30.8800320247936,0.620994014444089));
#32954=CARTESIAN_POINT('Ctrl Pts',(-38.6720109988941,33.0828274754107,0.463993887091835));
#32955=CARTESIAN_POINT('Ctrl Pts',(-38.6240716788406,37.0055467263343,0.306993759739582));
#32956=CARTESIAN_POINT('Ctrl Pts',(-35.3277244750448,39.1283073075518,0.149993632387328));
#32957=CARTESIAN_POINT('Ctrl Pts',(-31.734817208837,37.552345230412,-0.00700649496492534));
#32958=CARTESIAN_POINT('Ctrl Pts',(-31.0753017580586,33.6811081626476,-0.164006622317179));
#32959=CARTESIAN_POINT('Ctrl Pts',(-32.9741442474368,31.9005650466595,-0.268673373885348));
#32960=CARTESIAN_POINT('Ctrl Pts',(-34.0915279074966,31.601840982658,-0.321006749669432));
#32961=CARTESIAN_POINT('Ctrl Pts',(-32.1856025125516,37.4062712808594,8.10700224988981));
#32962=CARTESIAN_POINT('Ctrl Pts',(-31.3943716733878,36.4808402609044,8.05466887410573));
#32963=CARTESIAN_POINT('Ctrl Pts',(-30.8087963272068,33.8039236160346,7.95000212253756));
#32964=CARTESIAN_POINT('Ctrl Pts',(-33.6893083541881,30.8387967084451,7.79300199518531));
#32965=CARTESIAN_POINT('Ctrl Pts',(-37.7459632902934,31.614016197849,7.63600186783304));
#32966=CARTESIAN_POINT('Ctrl Pts',(-39.3398463967498,35.4211278497445,7.47900174048081));
#32967=CARTESIAN_POINT('Ctrl Pts',(-37.0423695151407,38.8527626110617,7.32200161312853));
#32968=CARTESIAN_POINT('Ctrl Pts',(-32.9133699266814,38.8285200429468,7.1650014857763));
#32969=CARTESIAN_POINT('Ctrl Pts',(-30.6555263540774,35.3717370910488,7.00800135842403));
#32970=CARTESIAN_POINT('Ctrl Pts',(-32.2933867652647,31.5813506589181,6.85100123107178));
#32971=CARTESIAN_POINT('Ctrl Pts',(-36.3583067411276,30.8566305931499,6.69400110371953));
#32972=CARTESIAN_POINT('Ctrl Pts',(-39.2052133232691,33.8472447317679,6.53700097636727));
#32973=CARTESIAN_POINT('Ctrl Pts',(-38.2812681058037,37.8715777961968,6.38000084901503));
#32974=CARTESIAN_POINT('Ctrl Pts',(-34.4149766453488,39.3209235066531,6.22300072166276));
#32975=CARTESIAN_POINT('Ctrl Pts',(-31.0732820603757,36.8956635970443,6.06600059431052));
#32976=CARTESIAN_POINT('Ctrl Pts',(-31.2527127155268,32.770540011044,5.90900046695826));
#32977=CARTESIAN_POINT('Ctrl Pts',(-34.7923720308581,30.644596543105,5.75200033960601));
#32978=CARTESIAN_POINT('Ctrl Pts',(-38.5182132375505,32.424184166957,5.59500021225375));
#32979=CARTESIAN_POINT('Ctrl Pts',(-39.0892389317987,36.5135310420632,5.43800008490151));
#32980=CARTESIAN_POINT('Ctrl Pts',(-35.9934048207584,39.2456798720372,5.28099995754924));
#32981=CARTESIAN_POINT('Ctrl Pts',(-32.0067750889435,38.1706869484817,5.12399983019699));
#32982=CARTESIAN_POINT('Ctrl Pts',(-30.7041988444697,34.2525085609798,4.96699970284475));
#32983=CARTESIAN_POINT('Ctrl Pts',(-33.2537087112384,31.0046129472743,4.80999957549248));
#32984=CARTESIAN_POINT('Ctrl Pts',(-37.3691347282993,31.3394192191957,4.65299944814024));
#32985=CARTESIAN_POINT('Ctrl Pts',(-39.3601349067833,34.9567034025226,4.49599932078798));
#32986=CARTESIAN_POINT('Ctrl Pts',(-37.4413602847608,38.6128120565681,4.33899919343573));
#32987=CARTESIAN_POINT('Ctrl Pts',(-33.3333944741925,39.0292774815619,4.18199906608348));
#32988=CARTESIAN_POINT('Ctrl Pts',(-30.7198898272843,35.8326511327341,4.02499893873122));
#32989=CARTESIAN_POINT('Ctrl Pts',(-31.9444010336713,31.8893785256963,3.86799881137897));
#32990=CARTESIAN_POINT('Ctrl Pts',(-35.9088971475179,30.7354300360637,3.71099868402671));
#32991=CARTESIAN_POINT('Ctrl Pts',(-39.0583764690558,33.4055623463097,3.55399855667446));
#32992=CARTESIAN_POINT('Ctrl Pts',(-38.5686706776456,37.5054421955447,3.39699842932221));
#32993=CARTESIAN_POINT('Ctrl Pts',(-34.8789036509792,39.3586679946839,3.23999830196995));
#32994=CARTESIAN_POINT('Ctrl Pts',(-31.297724886933,37.3034343822775,3.0829981746177));
#32995=CARTESIAN_POINT('Ctrl Pts',(-31.0364117253094,33.1826890722831,2.92599804726545));
#32996=CARTESIAN_POINT('Ctrl Pts',(-34.3292862136479,30.6915438832177,2.76899791991319));
#32997=CARTESIAN_POINT('Ctrl Pts',(-38.2235961502677,32.0638326727334,2.61199779256094));
#32998=CARTESIAN_POINT('Ctrl Pts',(-39.2272765706619,36.0690107818723,2.45499766520869));
#32999=CARTESIAN_POINT('Ctrl Pts',(-36.440317379388,39.1155968506723,2.29799753785644));
#33000=CARTESIAN_POINT('Ctrl Pts',(-32.3618120906526,38.4716873708438,2.14099741050418));
#33001=CARTESIAN_POINT('Ctrl Pts',(-30.6489945765686,34.714683263722,1.98399728315193));
#33002=CARTESIAN_POINT('Ctrl Pts',(-32.8377666428914,31.2135239126685,1.82699715579967));
#33003=CARTESIAN_POINT('Ctrl Pts',(-36.965431534851,31.1077370132983,1.66999702844742));
#33004=CARTESIAN_POINT('Ctrl Pts',(-39.3306802888702,34.4921735952445,1.51299690109517));
#33005=CARTESIAN_POINT('Ctrl Pts',(-37.8125560580904,38.3319952314996,1.35599677374291));
#33006=CARTESIAN_POINT('Ctrl Pts',(-33.7724068216079,39.1839601136936,1.19899664639066));
#33007=CARTESIAN_POINT('Ctrl Pts',(-30.8330098793911,36.2841775011547,1.04199651903841));
#33008=CARTESIAN_POINT('Ctrl Pts',(-31.6302781259105,32.2327605422985,0.884996391686154));
#33009=CARTESIAN_POINT('Ctrl Pts',(-35.4490367539887,30.6629552947093,0.7279962643339));
#33010=CARTESIAN_POINT('Ctrl Pts',(-38.8654853524014,32.981813694442,0.570996136981647));
#33011=CARTESIAN_POINT('Ctrl Pts',(-38.8150201605686,37.1112168499867,0.413996009629392));
#33012=CARTESIAN_POINT('Ctrl Pts',(-35.3449919290248,39.3458234281866,0.256995882277139));
#33013=CARTESIAN_POINT('Ctrl Pts',(-31.5627782008402,37.6868255855989,0.0999957549248854));
#33014=CARTESIAN_POINT('Ctrl Pts',(-30.8685135825059,33.611617154681,-0.0570043724273683));
#33015=CARTESIAN_POINT('Ctrl Pts',(-32.8674040627957,31.7372591159268,-0.161671123995537));
#33016=CARTESIAN_POINT('Ctrl Pts',(-34.0436614793107,31.4227955987545,-0.214004499779622));
#33017=CARTESIAN_POINT('Ctrl Pts',(-32.0447369588746,37.5267093987113,8.21400449977962));
#33018=CARTESIAN_POINT('Ctrl Pts',(-31.2139036219321,36.5549589254462,8.16167112399554));
#33019=CARTESIAN_POINT('Ctrl Pts',(-30.5990191977949,33.7440578853343,8.05700437242737));
#33020=CARTESIAN_POINT('Ctrl Pts',(-33.6237059276614,30.6305211509797,7.90000424507511));
#33021=CARTESIAN_POINT('Ctrl Pts',(-37.8834035918105,31.4445417418923,7.74300411772286));
#33022=CARTESIAN_POINT('Ctrl Pts',(-39.5570633564287,35.4422060407206,7.58600399037061));
#33023=CARTESIAN_POINT('Ctrl Pts',(-37.1445937083637,39.0456001689453,7.42900386301835));
#33024=CARTESIAN_POINT('Ctrl Pts',(-32.8089304145272,39.0201442175769,7.27200373566611));
#33025=CARTESIAN_POINT('Ctrl Pts',(-30.4380777924235,35.3903431875176,7.11500360831384));
#33026=CARTESIAN_POINT('Ctrl Pts',(-32.1579160033695,31.4102412351758,6.9580034809616));
#33027=CARTESIAN_POINT('Ctrl Pts',(-36.4262923870805,30.6492476530402,6.80100335360934));
#33028=CARTESIAN_POINT('Ctrl Pts',(-39.4156916603747,33.7895472992489,6.64400322625709));
#33029=CARTESIAN_POINT('Ctrl Pts',(-38.4455013566321,38.0153053250877,6.48700309890483));
#33030=CARTESIAN_POINT('Ctrl Pts',(-34.3856951955414,39.5371933423375,6.33000297155258));
#33031=CARTESIAN_POINT('Ctrl Pts',(-30.876742907976,36.9905449005467,6.17300284420033));
#33032=CARTESIAN_POINT('Ctrl Pts',(-31.0651543836038,32.6589516099224,6.01600271684807));
#33033=CARTESIAN_POINT('Ctrl Pts',(-34.781979885128,30.4266009251517,5.85900258949583));
#33034=CARTESIAN_POINT('Ctrl Pts',(-38.694306009759,32.295260045503,5.70200246214356));
#33035=CARTESIAN_POINT('Ctrl Pts',(-39.2939125462453,36.5892859378086,5.54500233479132));
#33036=CARTESIAN_POINT('Ctrl Pts',(-36.0431264825797,39.4581836312174,5.38800220743905));
#33037=CARTESIAN_POINT('Ctrl Pts',(-31.8569589075916,38.3293854175239,5.23100208008681));
#33038=CARTESIAN_POINT('Ctrl Pts',(-30.4891864267288,34.2150952972543,5.07400195273455));
#33039=CARTESIAN_POINT('Ctrl Pts',(-33.166303754984,30.8046367847576,4.9170018253823));
#33040=CARTESIAN_POINT('Ctrl Pts',(-37.487714096255,31.1562007005724,4.76000169803004));
#33041=CARTESIAN_POINT('Ctrl Pts',(-39.578367342141,34.9545363315231,4.60300157067779));
#33042=CARTESIAN_POINT('Ctrl Pts',(-37.5635546690906,38.7936396663671,4.44600144332554));
#33043=CARTESIAN_POINT('Ctrl Pts',(-33.2499779307934,39.2309499197622,4.28900131597329));
#33044=CARTESIAN_POINT('Ctrl Pts',(-30.5056627708833,35.8743267891954,4.13200118862103));
#33045=CARTESIAN_POINT('Ctrl Pts',(-31.7914629209398,31.7336864394819,3.97500106126878));
#33046=CARTESIAN_POINT('Ctrl Pts',(-35.9543890513771,30.5219807944966,3.81800093391652));
#33047=CARTESIAN_POINT('Ctrl Pts',(-39.2615053628575,33.3257579320817,3.66100080656427));
#33048=CARTESIAN_POINT('Ctrl Pts',(-38.747288933645,37.630843992432,3.50400067921202));
#33049=CARTESIAN_POINT('Ctrl Pts',(-34.8728425653191,39.5768270085061,3.34700055185976));
#33050=CARTESIAN_POINT('Ctrl Pts',(-31.1124194935077,37.4187253321399,3.19000042450751));
#33051=CARTESIAN_POINT('Ctrl Pts',(-30.8380271476682,33.0917294579507,3.03300029715526));
#33052=CARTESIAN_POINT('Ctrl Pts',(-34.2957158067332,30.4758980623661,2.87600016980301));
#33053=CARTESIAN_POINT('Ctrl Pts',(-38.3849428180941,31.916872323995,2.71900004245075));
#33054=CARTESIAN_POINT('Ctrl Pts',(-39.4388592121786,36.1225166552775,2.5619999150985));
#33055=CARTESIAN_POINT('Ctrl Pts',(-36.5124078023019,39.3215897254055,2.40499978774625));
#33056=CARTESIAN_POINT('Ctrl Pts',(-32.2297661368697,38.6454514414374,2.24799966039399));
#33057=CARTESIAN_POINT('Ctrl Pts',(-30.4312190879402,34.7004026582963,2.09099953304174));
#33058=CARTESIAN_POINT('Ctrl Pts',(-32.7295430531581,31.0240041121053,1.93399940568948));
#33059=CARTESIAN_POINT('Ctrl Pts',(-37.0638048465832,30.9129223920078,1.77699927833723));
#33060=CARTESIAN_POINT('Ctrl Pts',(-39.5474384686975,34.466755988813,1.61999915098498));
#33061=CARTESIAN_POINT('Ctrl Pts',(-37.9533294449832,38.4987674643586,1.46299902363273));
#33062=CARTESIAN_POINT('Ctrl Pts',(-33.7109636198088,39.3933746902084,1.30599889628047));
#33063=CARTESIAN_POINT('Ctrl Pts',(-30.6244446809342,36.348452848019,1.14899876892822));
#33064=CARTESIAN_POINT('Ctrl Pts',(-31.4616176081094,32.0942553311105,0.991998641575964));
#33065=CARTESIAN_POINT('Ctrl Pts',(-35.4715118348024,30.445878564625,0.834998514223711));
#33066=CARTESIAN_POINT('Ctrl Pts',(-39.0589597059086,32.8807999134734,0.677998386871457));
#33067=CARTESIAN_POINT('Ctrl Pts',(-39.0059686422967,37.2168869736391,0.520998259519203));
#33068=CARTESIAN_POINT('Ctrl Pts',(-35.3622593830049,39.5633395488214,0.36399813216695));
#33069=CARTESIAN_POINT('Ctrl Pts',(-31.3907391928433,37.8213059407857,0.206998004814696));
#33070=CARTESIAN_POINT('Ctrl Pts',(-30.6617254069532,33.5421261467143,0.0499978774624425));
#33071=CARTESIAN_POINT('Ctrl Pts',(-32.7606638781546,31.573953185194,-0.0546688741057264));
#33072=CARTESIAN_POINT('Ctrl Pts',(-33.9957950511247,31.243750214851,-0.107002249889811));
#33073=CARTESIAN_POINT('Ctrl Pts',(-31.9038714051976,37.6471475165632,8.32100674966943));
#33074=CARTESIAN_POINT('Ctrl Pts',(-31.0334355704763,36.629077589988,8.26867337388535));
#33075=CARTESIAN_POINT('Ctrl Pts',(-30.3892420683829,33.6841921546339,8.16400662231718));
#33076=CARTESIAN_POINT('Ctrl Pts',(-33.5581035011348,30.4222455935143,8.00700649496493));
#33077=CARTESIAN_POINT('Ctrl Pts',(-38.0208438933277,31.2750672859355,7.85000636761266));
#33078=CARTESIAN_POINT('Ctrl Pts',(-39.7742803161076,35.4632842316967,7.69300624026044));
#33079=CARTESIAN_POINT('Ctrl Pts',(-37.2468179015868,39.238437726829,7.53600611290815));
#33080=CARTESIAN_POINT('Ctrl Pts',(-32.7044909023729,39.2117683922069,7.37900598555592));
#33081=CARTESIAN_POINT('Ctrl Pts',(-30.2206292307696,35.4089492839864,7.22200585820365));
#33082=CARTESIAN_POINT('Ctrl Pts',(-32.0224452414743,31.2391318114334,7.0650057308514));
#33083=CARTESIAN_POINT('Ctrl Pts',(-36.4942780330333,30.4418647129305,6.90800560349915));
#33084=CARTESIAN_POINT('Ctrl Pts',(-39.6261699974803,33.7318498667299,6.7510054761469));
#33085=CARTESIAN_POINT('Ctrl Pts',(-38.6097346074605,38.1590328539788,6.59400534879465));
#33086=CARTESIAN_POINT('Ctrl Pts',(-34.3564137457339,39.7534631780217,6.4370052214424));
#33087=CARTESIAN_POINT('Ctrl Pts',(-30.6802037555765,37.0854262040492,6.28000509409013));
#33088=CARTESIAN_POINT('Ctrl Pts',(-30.8775960516807,32.5473632088007,6.12300496673789));
#33089=CARTESIAN_POINT('Ctrl Pts',(-34.7715877393978,30.2086053071985,5.96600483938563));
#33090=CARTESIAN_POINT('Ctrl Pts',(-38.8703987819675,32.166335924049,5.80900471203337));
#33091=CARTESIAN_POINT('Ctrl Pts',(-39.4985861606919,36.6650408335539,5.65200458468113));
#33092=CARTESIAN_POINT('Ctrl Pts',(-36.092848144401,39.6706873903976,5.49500445732886));
#33093=CARTESIAN_POINT('Ctrl Pts',(-31.7071427262397,38.4880838865661,5.33800432997662));
#33094=CARTESIAN_POINT('Ctrl Pts',(-30.2741740089879,34.1776820335287,5.18100420262436));
#33095=CARTESIAN_POINT('Ctrl Pts',(-33.0788987987297,30.6046606222411,5.02400407527212));
#33096=CARTESIAN_POINT('Ctrl Pts',(-37.6062934642105,30.9729821819491,4.86700394791985));
#33097=CARTESIAN_POINT('Ctrl Pts',(-39.7965997774987,34.9523692605237,4.7100038205676));
#33098=CARTESIAN_POINT('Ctrl Pts',(-37.6857490534203,38.974467276166,4.55300369321535));
#33099=CARTESIAN_POINT('Ctrl Pts',(-33.1665613873943,39.4326223579625,4.3960035658631));
#33100=CARTESIAN_POINT('Ctrl Pts',(-30.2914357144823,35.9160024456566,4.23900343851084));
#33101=CARTESIAN_POINT('Ctrl Pts',(-31.6385248082081,31.5779943532675,4.08200331115859));
#33102=CARTESIAN_POINT('Ctrl Pts',(-35.9998809552364,30.3085315529294,3.92500318380634));
#33103=CARTESIAN_POINT('Ctrl Pts',(-39.464634256659,33.2459535178537,3.76800305645409));
#33104=CARTESIAN_POINT('Ctrl Pts',(-38.9259071896446,37.7562457893193,3.61100292910183));
#33105=CARTESIAN_POINT('Ctrl Pts',(-34.866781479659,39.7949860223284,3.45400280174958));
#33106=CARTESIAN_POINT('Ctrl Pts',(-30.9271141000824,37.5340162820022,3.29700267439732));
#33107=CARTESIAN_POINT('Ctrl Pts',(-30.6396425700269,33.0007698436185,3.14000254704507));
#33108=CARTESIAN_POINT('Ctrl Pts',(-34.2621453998186,30.2602522415144,2.98300241969281));
#33109=CARTESIAN_POINT('Ctrl Pts',(-38.5462894859204,31.7699119752566,2.82600229234057));
#33110=CARTESIAN_POINT('Ctrl Pts',(-39.6504418536953,36.1760225286826,2.66900216498831));
#33111=CARTESIAN_POINT('Ctrl Pts',(-36.5844982252159,39.5275826001387,2.51200203763606));
#33112=CARTESIAN_POINT('Ctrl Pts',(-32.0977201830868,38.819215512031,2.3550019102838));
#33113=CARTESIAN_POINT('Ctrl Pts',(-30.2134435993119,34.6861220528707,2.19800178293155));
#33114=CARTESIAN_POINT('Ctrl Pts',(-32.6213194634248,30.8344843115421,2.04100165557929));
#33115=CARTESIAN_POINT('Ctrl Pts',(-37.1621781583154,30.7181077707172,1.88400152822704));
#33116=CARTESIAN_POINT('Ctrl Pts',(-39.7641966485248,34.4413383823816,1.72700140087479));
#33117=CARTESIAN_POINT('Ctrl Pts',(-38.0941028318759,38.6655396972175,1.57000127352254));
#33118=CARTESIAN_POINT('Ctrl Pts',(-33.6495204180096,39.602789266723,1.41300114617028));
#33119=CARTESIAN_POINT('Ctrl Pts',(-30.4158794824773,36.4127281948833,1.25600101881803));
#33120=CARTESIAN_POINT('Ctrl Pts',(-31.2929570903083,31.9557501199225,1.09900089146578));
#33121=CARTESIAN_POINT('Ctrl Pts',(-35.4939869156159,30.2288018345407,0.942000764113521));
#33122=CARTESIAN_POINT('Ctrl Pts',(-39.2524340594159,32.7797861325047,0.785000636761268));
#33123=CARTESIAN_POINT('Ctrl Pts',(-39.1969171240247,37.3225570972915,0.628000509409013));
#33124=CARTESIAN_POINT('Ctrl Pts',(-35.379526836985,39.7808556694562,0.471000382056761));
#33125=CARTESIAN_POINT('Ctrl Pts',(-31.2187001848465,37.9557862959725,0.314000254704507));
#33126=CARTESIAN_POINT('Ctrl Pts',(-30.4549372314006,33.4726351387477,0.157000127352253));
#33127=CARTESIAN_POINT('Ctrl Pts',(-32.6539236935135,31.4106472544613,0.0523333757840845));
#33128=CARTESIAN_POINT('Ctrl Pts',(-33.9479286229388,31.0647048309474,0.));
#33129=CARTESIAN_POINT('Ctrl Pts',(-33.9479286229388,31.0647048309474,0.));
#33130=CARTESIAN_POINT('Ctrl Pts',(-33.8318205444026,31.104319484649,-6.12910217551102E-18));
#33131=CARTESIAN_POINT('Ctrl Pts',(-33.7179775273608,31.1494845452793,-1.6976040424202E-15));
#33132=CARTESIAN_POINT('Ctrl Pts',(-33.6066254658749,31.1998424056554,-1.16573417585641E-15));
#33133=CARTESIAN_POINT('Ctrl Pts',(-33.4927762352539,31.2513295858929,-6.21936653918048E-16));
#33134=CARTESIAN_POINT('Ctrl Pts',(-33.3815303134372,31.3082455820535,1.45039252013455E-15));
#33135=CARTESIAN_POINT('Ctrl Pts',(-33.2731534080755,31.3702567597409,9.99200722162641E-16));
#33136=CARTESIAN_POINT('Ctrl Pts',(-33.1592150345376,31.4354501023936,5.24855570462807E-16));
#33137=CARTESIAN_POINT('Ctrl Pts',(-33.0484467137175,31.5062753971616,-4.62145718692395E-16));
#33138=CARTESIAN_POINT('Ctrl Pts',(-32.9411963534997,31.5823911623814,-5.55111512312578E-16));
#33139=CARTESIAN_POINT('Ctrl Pts',(-32.8473522883091,31.6489924569487,-6.36456581730239E-16));
#33140=CARTESIAN_POINT('Ctrl Pts',(-32.7562019661932,31.7196453256574,-1.95036301750383E-15));
#33141=CARTESIAN_POINT('Ctrl Pts',(-32.6680099559688,31.7941431443398,-1.99840144432528E-15));
#33142=CARTESIAN_POINT('Ctrl Pts',(-32.6506336549248,31.8088213053349,-2.00786636256454E-15));
#33143=CARTESIAN_POINT('Ctrl Pts',(-32.6333722976869,31.8236487792666,-7.57847684029515E-16));
#33144=CARTESIAN_POINT('Ctrl Pts',(-32.6162280624477,31.8386240567023,-7.7715611723761E-16));
#33145=CARTESIAN_POINT('Ctrl Pts',(-32.6036937742642,31.8495726024021,-7.91272667951259E-16));
#33146=CARTESIAN_POINT('Ctrl Pts',(-32.5912233028683,31.8605991578939,4.81364284937086E-16));
#33147=CARTESIAN_POINT('Ctrl Pts',(-32.5788262971356,31.8716950114967,4.44089209850063E-16));
#33148=CARTESIAN_POINT('Ctrl Pts',(-32.4862471134748,31.9545573647705,1.6572392577578E-16));
#33149=CARTESIAN_POINT('Ctrl Pts',(-32.3976237822216,32.0414014202655,8.13390076176465E-16));
#33150=CARTESIAN_POINT('Ctrl Pts',(-32.3132177297223,32.1319062612438,6.38378239159465E-16));
#33151=CARTESIAN_POINT('Ctrl Pts',(-32.2290034543674,32.222205468154,4.63764042706654E-16));
#33152=CARTESIAN_POINT('Ctrl Pts',(-32.1489867981842,32.3161495489862,3.17588722629917E-16));
#33153=CARTESIAN_POINT('Ctrl Pts',(-32.0734678385385,32.4134518063003,8.88178419700125E-16));
#33154=CARTESIAN_POINT('Ctrl Pts',(-31.9989812077255,32.5094239615292,1.4509682715575E-15));
#33155=CARTESIAN_POINT('Ctrl Pts',(-31.9288697495096,32.6086637947563,-1.05272258015246E-15));
#33156=CARTESIAN_POINT('Ctrl Pts',(-31.8634674410238,32.710917033623,-1.02695629777827E-15));
#33157=CARTESIAN_POINT('Ctrl Pts',(-31.8101619976839,32.7942574287394,-1.00595576833249E-15));
#33158=CARTESIAN_POINT('Ctrl Pts',(-31.7599855228772,32.8796001211512,6.44886685271164E-16));
#33159=CARTESIAN_POINT('Ctrl Pts',(-31.7131447814318,32.9668132818295,6.10622663543836E-16));
#33160=CARTESIAN_POINT('Ctrl Pts',(-31.7012439418187,32.9889715527142,6.01917194448022E-16));
#33161=CARTESIAN_POINT('Ctrl Pts',(-31.6895585553312,33.0112505813609,1.19774783640231E-15));
#33162=CARTESIAN_POINT('Ctrl Pts',(-31.6780922762038,33.0336482309453,1.16573417585641E-15));
#33163=CARTESIAN_POINT('Ctrl Pts',(-31.6699364387253,33.0495794312833,1.14296321331454E-15));
#33164=CARTESIAN_POINT('Ctrl Pts',(-31.661895167037,33.0655634624947,-2.51368181031482E-15));
#33165=CARTESIAN_POINT('Ctrl Pts',(-31.6539721233883,33.0815939077556,-2.4980018054066E-15));
#33166=CARTESIAN_POINT('Ctrl Pts',(-31.6010112907938,33.1887478962384,-2.3931903021702E-15));
#33167=CARTESIAN_POINT('Ctrl Pts',(-31.5532893085976,33.2980517601776,-1.33576692347369E-15));
#33168=CARTESIAN_POINT('Ctrl Pts',(-31.5110849763849,33.409242888583,-1.0547118733939E-15));
#33169=CARTESIAN_POINT('Ctrl Pts',(-31.469716801377,33.5182310852453,-7.79225119096594E-16));
#33170=CARTESIAN_POINT('Ctrl Pts',(-31.4336495378063,33.6290331387016,-1.04560375035282E-15));
#33171=CARTESIAN_POINT('Ctrl Pts',(-31.4031939533011,33.7414155242157,-1.19348975147204E-15));
#33172=CARTESIAN_POINT('Ctrl Pts',(-31.3987398005021,33.7578515350533,-1.2151181935629E-15));
#33173=CARTESIAN_POINT('Ctrl Pts',(-31.3944057673546,33.7743213630571,-1.05328088726205E-15));
#33174=CARTESIAN_POINT('Ctrl Pts',(-31.390192920076,33.7908242908111,-1.11022302462516E-15));
#33175=CARTESIAN_POINT('Ctrl Pts',(-31.3605243708329,33.9070444840312,-1.45504712955035E-15));
#33176=CARTESIAN_POINT('Ctrl Pts',(-31.336861805495,34.0249066128039,2.32711961845814E-15));
#33177=CARTESIAN_POINT('Ctrl Pts',(-31.3191143685546,34.1439748333396,2.41473507855972E-15));
#33178=CARTESIAN_POINT('Ctrl Pts',(-31.3091308324304,34.2109547519018,2.46402175098999E-15));
#33179=CARTESIAN_POINT('Ctrl Pts',(-31.3010200590003,34.2783162816674,1.31577829093223E-15));
#33180=CARTESIAN_POINT('Ctrl Pts',(-31.2947729234008,34.3459803828548,1.66533453693773E-15));
#33181=CARTESIAN_POINT('Ctrl Pts',(-31.2918904510582,34.3772010754682,1.82662224956662E-15));
#33182=CARTESIAN_POINT('Ctrl Pts',(-31.2894048093972,34.4084861625173,5.36743605776751E-16));
#33183=CARTESIAN_POINT('Ctrl Pts',(-31.2873154495445,34.4398277448617,5.55111512312578E-16));
#33184=CARTESIAN_POINT('Ctrl Pts',(-31.2861143588149,34.4578447867584,5.6567049870877E-16));
#33185=CARTESIAN_POINT('Ctrl Pts',(-31.2850447395365,34.4758734447918,-4.83710549279582E-16));
#33186=CARTESIAN_POINT('Ctrl Pts',(-31.2841065224407,34.4939038782769,-4.44089209850063E-16));
#33187=CARTESIAN_POINT('Ctrl Pts',(-31.2777956059898,34.6151855728967,-1.77576305814986E-16));
#33188=CARTESIAN_POINT('Ctrl Pts',(-31.2774172190669,34.7366645735772,1.74591754833025E-15));
#33189=CARTESIAN_POINT('Ctrl Pts',(-31.2828131531898,34.8578936251582,1.77635683940025E-15));
#33190=CARTESIAN_POINT('Ctrl Pts',(-31.2880971535264,34.9766078894115,1.80616469483294E-15));
#33191=CARTESIAN_POINT('Ctrl Pts',(-31.2989188936952,35.0950833906807,2.23513941723243E-15));
#33192=CARTESIAN_POINT('Ctrl Pts',(-31.3151831802674,35.2128941454877,2.73392419813945E-15));
#33193=CARTESIAN_POINT('Ctrl Pts',(-31.3312885576294,35.3295538375714,3.22783563306706E-15));
#33194=CARTESIAN_POINT('Ctrl Pts',(-31.3527309988427,35.445562546077,2.65572620552751E-15));
#33195=CARTESIAN_POINT('Ctrl Pts',(-31.3794648565834,35.5604877518601,3.06699110552699E-15));
#33196=CARTESIAN_POINT('Ctrl Pts',(-31.3968717688464,35.6353176919788,3.33477333511016E-15));
#33197=CARTESIAN_POINT('Ctrl Pts',(-31.4165229425865,35.7096878616141,5.4636862845821E-16));
#33198=CARTESIAN_POINT('Ctrl Pts',(-31.4384155780607,35.7834719630247,4.85722573273506E-16));
#33199=CARTESIAN_POINT('Ctrl Pts',(-31.4458039236167,35.8083726853891,4.65255690113341E-16));
#33200=CARTESIAN_POINT('Ctrl Pts',(-31.45344761912,35.8332066040146,2.20922363074103E-15));
#33201=CARTESIAN_POINT('Ctrl Pts',(-31.4613467446,35.8579686875435,2.27595720048157E-15));
#33202=CARTESIAN_POINT('Ctrl Pts',(-31.4664331437066,35.8739134702743,2.31892823194254E-15));
#33203=CARTESIAN_POINT('Ctrl Pts',(-31.4716246609433,35.8898258563265,-1.15821499265833E-16));
#33204=CARTESIAN_POINT('Ctrl Pts',(-31.4769184371132,35.9056964793841,2.77555756156289E-17));
#33205=CARTESIAN_POINT('Ctrl Pts',(-31.5138161242914,36.0163149237837,1.02848961215397E-15));
#33206=CARTESIAN_POINT('Ctrl Pts',(-31.5557145226016,36.1250218909898,1.27042107846669E-15));
#33207=CARTESIAN_POINT('Ctrl Pts',(-31.6025488384922,36.2313981798515,1.95676808090184E-15));
#33208=CARTESIAN_POINT('Ctrl Pts',(-31.6406629331589,36.3179679496208,2.51532208404033E-15));
#33209=CARTESIAN_POINT('Ctrl Pts',(-31.6820469345646,36.4029939678578,-2.48735046316874E-16));
#33210=CARTESIAN_POINT('Ctrl Pts',(-31.7266869042645,36.4862346415976,-4.02455846426619E-16));
#33211=CARTESIAN_POINT('Ctrl Pts',(-31.748301897583,36.5265403725114,-4.76888559747074E-16));
#33212=CARTESIAN_POINT('Ctrl Pts',(-31.7706805448521,36.566427275075,1.22980137611631E-15));
#33213=CARTESIAN_POINT('Ctrl Pts',(-31.7938227368542,36.6058663963511,1.14491749414469E-15));
#33214=CARTESIAN_POINT('Ctrl Pts',(-31.8074091619825,36.6290204981016,1.09508347207335E-15));
#33215=CARTESIAN_POINT('Ctrl Pts',(-31.8212608195948,36.6520233300662,-7.62339319688486E-16));
#33216=CARTESIAN_POINT('Ctrl Pts',(-31.8353636346369,36.6748465408533,-5.68989300120393E-16));
#33217=CARTESIAN_POINT('Ctrl Pts',(-31.8937950765752,36.7694087337193,2.32107531151829E-16));
#33218=CARTESIAN_POINT('Ctrl Pts',(-31.9565777772527,36.8609657133175,3.78686475409805E-16));
#33219=CARTESIAN_POINT('Ctrl Pts',(-32.0236776904421,36.9491267660533,4.5102810375397E-17));
#33220=CARTESIAN_POINT('Ctrl Pts',(-32.0837084847486,37.0279998639616,-2.53337104489111E-16));
#33221=CARTESIAN_POINT('Ctrl Pts',(-32.1471953789829,37.1041548289018,-7.94184032652028E-16));
#33222=CARTESIAN_POINT('Ctrl Pts',(-32.2141374826654,37.1772853486058,-1.07986536379556E-15));
#33223=CARTESIAN_POINT('Ctrl Pts',(-32.2489924160368,37.2153624219495,-1.21791469682805E-15));
#33224=CARTESIAN_POINT('Ctrl Pts',(-32.2847844521695,37.2526190806637,6.40917790468134E-17));
#33225=CARTESIAN_POINT('Ctrl Pts',(-32.3214761820288,37.2890399271606,-2.77555756156289E-17));
#33226=CARTESIAN_POINT('Ctrl Pts',(-38.5163029138352,34.997016742257,6.38741669750802));
#33227=CARTESIAN_POINT('Ctrl Pts',(-38.5189470194328,34.6831064778252,6.4016107071645));
#33228=CARTESIAN_POINT('Ctrl Pts',(-38.4802904146781,34.3698362574768,6.41580471682098));
#33229=CARTESIAN_POINT('Ctrl Pts',(-38.3977159824674,34.0686054096188,6.42999872647747));
#33230=CARTESIAN_POINT('Ctrl Pts',(-38.0932636891673,32.9579659539444,6.48233210226155));
#33231=CARTESIAN_POINT('Ctrl Pts',(-37.1917923921711,32.010989743602,6.53466547804563));
#33232=CARTESIAN_POINT('Ctrl Pts',(-36.0974794823371,31.6522427299976,6.58699885382972));
#33233=CARTESIAN_POINT('Ctrl Pts',(-35.0031665725032,31.2934957163932,6.6393322296138));
#33234=CARTESIAN_POINT('Ctrl Pts',(-33.7160120498315,31.5229778995268,6.69166560539789));
#33235=CARTESIAN_POINT('Ctrl Pts',(-32.8131210199243,32.2378308097469,6.74399898118197));
#33236=CARTESIAN_POINT('Ctrl Pts',(-31.9102299900171,32.952683719967,6.79633235696605));
#33237=CARTESIAN_POINT('Ctrl Pts',(-31.3916024528742,34.1529073572735,6.84866573275014));
#33238=CARTESIAN_POINT('Ctrl Pts',(-31.4897611048202,35.3003133215496,6.90099910853422));
#33239=CARTESIAN_POINT('Ctrl Pts',(-31.5879197567661,36.4477192858256,6.95333248431831));
#33240=CARTESIAN_POINT('Ctrl Pts',(-32.3028645978009,37.5423075770711,7.00566586010239));
#33241=CARTESIAN_POINT('Ctrl Pts',(-33.3140596654986,38.0934399201708,7.05799923588648));
#33242=CARTESIAN_POINT('Ctrl Pts',(-34.3252547331963,38.6445722632704,7.11033261167056));
#33243=CARTESIAN_POINT('Ctrl Pts',(-35.6327000275569,38.6522486582243,7.16266598745464));
#33244=CARTESIAN_POINT('Ctrl Pts',(-36.6501700272628,38.1127742899662,7.21499936323873));
#33245=CARTESIAN_POINT('Ctrl Pts',(-37.6676400269687,37.5732999217082,7.26733273902281));
#33246=CARTESIAN_POINT('Ctrl Pts',(-38.3951347320199,36.4866747902383,7.3196661148069));
#33247=CARTESIAN_POINT('Ctrl Pts',(-38.5065310098296,35.3406023903429,7.37199949059099));
#33248=CARTESIAN_POINT('Ctrl Pts',(-38.5174699784391,35.2280595814352,7.37713855956333));
#33249=CARTESIAN_POINT('Ctrl Pts',(-38.5224679204996,35.1149435235394,7.38227762853568));
#33250=CARTESIAN_POINT('Ctrl Pts',(-38.521739013009,35.0017650567249,7.38741669750802));
#33251=CARTESIAN_POINT('Ctrl Pts',(-36.0520713770612,31.0647048309474,8.));
#33252=CARTESIAN_POINT('Ctrl Pts',(-37.3460763064866,31.4106472544613,7.94766662421592));
#33253=CARTESIAN_POINT('Ctrl Pts',(-39.5450624630061,33.4726371160361,7.84299987264775));
#33254=CARTESIAN_POINT('Ctrl Pts',(-38.7813000795415,37.9557855546777,7.6859997452955));
#33255=CARTESIAN_POINT('Ctrl Pts',(-34.6204731393245,39.7808563212243,7.52899961794324));
#33256=CARTESIAN_POINT('Ctrl Pts',(-30.8030827008644,37.3225569109026,7.37199949059099));
#33257=CARTESIAN_POINT('Ctrl Pts',(-30.7475658132336,32.7797862032913,7.21499936323873));
#33258=CARTESIAN_POINT('Ctrl Pts',(-34.5060130464714,30.2288015790917,7.05799923588648));
#33259=CARTESIAN_POINT('Ctrl Pts',(-38.707043056971,31.9557500555838,6.90099910853422));
#33260=CARTESIAN_POINT('Ctrl Pts',(-39.5841206744658,36.4127282212004,6.74399898118198));
#33261=CARTESIAN_POINT('Ctrl Pts',(-36.3504796357983,39.6027894460767,6.58699885382972));
#33262=CARTESIAN_POINT('Ctrl Pts',(-31.905897053523,38.6655398223873,6.42999872647746));
#33263=CARTESIAN_POINT('Ctrl Pts',(-30.2358031812474,34.4413383659989,6.27299859912522));
#33264=CARTESIAN_POINT('Ctrl Pts',(-32.8378217627235,30.7181076142107,6.11599847177296));
#33265=CARTESIAN_POINT('Ctrl Pts',(-37.3786806229274,30.8344841622903,5.95899834442071));
#33266=CARTESIAN_POINT('Ctrl Pts',(-39.7865565731199,34.68612204099,5.80199821706845));
#33267=CARTESIAN_POINT('Ctrl Pts',(-37.9022799217924,38.8192156501332,5.6449980897162));
#33268=CARTESIAN_POINT('Ctrl Pts',(-33.4155017175264,39.5275827633586,5.48799796236395));
#33269=CARTESIAN_POINT('Ctrl Pts',(-30.3495579785441,36.176022571197,5.33099783501169));
#33270=CARTESIAN_POINT('Ctrl Pts',(-31.4537103860929,31.7699118586619,5.17399770765944));
#33271=CARTESIAN_POINT('Ctrl Pts',(-35.7378546268185,30.2602520705083,5.01699758030719));
#33272=CARTESIAN_POINT('Ctrl Pts',(-39.3603575873042,33.0007697714678,4.85999745295493));
#33273=CARTESIAN_POINT('Ctrl Pts',(-39.0728860468858,37.5340163734447,4.70299732560268));
#33274=CARTESIAN_POINT('Ctrl Pts',(-35.1332185251462,39.7949861953461,4.54599719825043));
#33275=CARTESIAN_POINT('Ctrl Pts',(-31.0740926686951,37.7562458887763,4.38899707089817));
#33276=CARTESIAN_POINT('Ctrl Pts',(-30.5353655822401,33.2459534545604,4.23199694354592));
#33277=CARTESIAN_POINT('Ctrl Pts',(-34.0001190086845,30.3085313836444,4.07499681619366));
#33278=CARTESIAN_POINT('Ctrl Pts',(-38.3614753130862,31.5779942297887,3.91799668884141));
#33279=CARTESIAN_POINT('Ctrl Pts',(-39.70856445542,35.9160024787098,3.76099656148916));
#33280=CARTESIAN_POINT('Ctrl Pts',(-36.8334386787628,39.4326225179073,3.6039964341369));
#33281=CARTESIAN_POINT('Ctrl Pts',(-32.314250849668,38.9744674195804,3.44699630678465));
#33282=CARTESIAN_POINT('Ctrl Pts',(-30.2034000494222,34.9523692588031,3.2899961794324));
#33283=CARTESIAN_POINT('Ctrl Pts',(-32.3937064417451,30.9729820366429,3.13299605208014));
#33284=CARTESIAN_POINT('Ctrl Pts',(-36.9211012705904,30.6046604636344,2.97599592472789));
#33285=CARTESIAN_POINT('Ctrl Pts',(-39.7258261615381,34.1776820038694,2.81899579737564));
#33286=CARTESIAN_POINT('Ctrl Pts',(-38.2928573925768,38.4880840124043,2.66199567002338));
#33287=CARTESIAN_POINT('Ctrl Pts',(-33.9071518161688,39.6706875589806,2.50499554267113));
#33288=CARTESIAN_POINT('Ctrl Pts',(-30.5014136769744,36.6650408935442,2.34799541531887));
#33289=CARTESIAN_POINT('Ctrl Pts',(-31.1296010783918,32.1663358219723,2.19099528796663));
#33290=CARTESIAN_POINT('Ctrl Pts',(-35.2284122688067,30.2086051339802,2.03399516061437));
#33291=CARTESIAN_POINT('Ctrl Pts',(-39.1224040971504,32.5473631209192,1.87699503326212));
#33292=CARTESIAN_POINT('Ctrl Pts',(-39.319796400129,37.0854262781345,1.71999490590986));
#33293=CARTESIAN_POINT('Ctrl Pts',(-35.6435862778458,39.7534633517259,1.56299477855761));
#33294=CARTESIAN_POINT('Ctrl Pts',(-31.3902652615342,38.1590329639038,1.40599465120536));
#33295=CARTESIAN_POINT('Ctrl Pts',(-30.3738298371754,33.7318498284919,1.2489945238531));
#33296=CARTESIAN_POINT('Ctrl Pts',(-33.5057219097166,30.4418645346457,1.09199439650085));
#33297=CARTESIAN_POINT('Ctrl Pts',(-37.9775548729557,31.2391317008465,0.934994269148598));
#33298=CARTESIAN_POINT('Ctrl Pts',(-39.7793709270477,35.4089492535829,0.777994141796342));
#33299=CARTESIAN_POINT('Ctrl Pts',(-37.2955092110801,39.2117686241983,0.620994014444089));
#33300=CARTESIAN_POINT('Ctrl Pts',(-32.7531819533668,39.2384377406302,0.463993887091835));
#33301=CARTESIAN_POINT('Ctrl Pts',(-30.2257196451616,35.46328448449,0.306993759739582));
#33302=CARTESIAN_POINT('Ctrl Pts',(-31.9791557179606,31.2750667622313,0.149993632387329));
#33303=CARTESIAN_POINT('Ctrl Pts',(-36.4418971366481,30.4222460546565,-0.00700649496492604));
#33304=CARTESIAN_POINT('Ctrl Pts',(-39.6107565597589,33.6841906982476,-0.164006622317178));
#33305=CARTESIAN_POINT('Ctrl Pts',(-38.9665644295237,36.6290775899881,-0.268673373885348));
#33306=CARTESIAN_POINT('Ctrl Pts',(-38.0961285948024,37.6471475165632,-0.321006749669432));
#33307=CARTESIAN_POINT('Ctrl Pts',(-36.0042049488753,31.243750214851,8.10700224988981));
#33308=CARTESIAN_POINT('Ctrl Pts',(-37.2393361218455,31.5739531851941,8.05466887410573));
#33309=CARTESIAN_POINT('Ctrl Pts',(-39.3382743013571,33.5421280340415,7.95000212253756));
#33310=CARTESIAN_POINT('Ctrl Pts',(-38.6092610595157,37.8213052332178,7.79300199518531));
#33311=CARTESIAN_POINT('Ctrl Pts',(-34.6377405943825,39.5633401709358,7.63600186783305));
#33312=CARTESIAN_POINT('Ctrl Pts',(-30.9940311905596,37.2168867957304,7.4790017404808));
#33313=CARTESIAN_POINT('Ctrl Pts',(-30.941040172535,32.8807999810394,7.32200161312854));
#33314=CARTESIAN_POINT('Ctrl Pts',(-34.5284881290099,30.4458783207982,7.16500148577629));
#33315=CARTESIAN_POINT('Ctrl Pts',(-38.5383825324691,32.0942552696991,7.00800135842404));
#33316=CARTESIAN_POINT('Ctrl Pts',(-39.3755554688683,36.3484528731387,6.85100123107178));
#33317=CARTESIAN_POINT('Ctrl Pts',(-36.2890364315511,39.3933748614019,6.69400110371953));
#33318=CARTESIAN_POINT('Ctrl Pts',(-32.0466704456298,38.4987675838335,6.53700097636727));
#33319=CARTESIAN_POINT('Ctrl Pts',(-30.4525613688197,34.4667559731757,6.38000084901503));
#33320=CARTESIAN_POINT('Ctrl Pts',(-32.9361950780481,30.9129222426219,6.22300072166277));
#33321=CARTESIAN_POINT('Ctrl Pts',(-37.2704570292653,31.024003969644,6.06600059431052));
#33322=CARTESIAN_POINT('Ctrl Pts',(-39.5687810766463,34.7004026469562,5.90900046695827));
#33323=CARTESIAN_POINT('Ctrl Pts',(-37.7702339632379,38.6454515732563,5.752000339606));
#33324=CARTESIAN_POINT('Ctrl Pts',(-33.4875921430454,39.3215898811993,5.59500021225376));
#33325=CARTESIAN_POINT('Ctrl Pts',(-30.5611406276935,36.1225166958576,5.4380000849015));
#33326=CARTESIAN_POINT('Ctrl Pts',(-31.6150570597422,31.916872212705,5.28099995754925));
#33327=CARTESIAN_POINT('Ctrl Pts',(-35.7042842186919,30.4758978991403,5.123999830197));
#33328=CARTESIAN_POINT('Ctrl Pts',(-39.1619730025048,33.0917293890828,4.96699970284474));
#33329=CARTESIAN_POINT('Ctrl Pts',(-38.8875806467738,37.4187254194219,4.80999957549249));
#33330=CARTESIAN_POINT('Ctrl Pts',(-35.1271574392675,39.576827173652,4.65299944814024));
#33331=CARTESIAN_POINT('Ctrl Pts',(-31.2527109311398,37.6308440873639,4.49599932078798));
#33332=CARTESIAN_POINT('Ctrl Pts',(-30.7384944833714,33.3257578716681,4.33899919343573));
#33333=CARTESIAN_POINT('Ctrl Pts',(-34.0456109141852,30.5219806329136,4.18199906608347));
#33334=CARTESIAN_POINT('Ctrl Pts',(-38.208537194836,31.7336863216211,4.02499893873123));
#33335=CARTESIAN_POINT('Ctrl Pts',(-39.4943373912889,35.8743268207447,3.86799881137897));
#33336=CARTESIAN_POINT('Ctrl Pts',(-36.7500221323538,39.23095007243,3.71099868402672));
#33337=CARTESIAN_POINT('Ctrl Pts',(-32.4364452384069,38.7936398032564,3.55399855667446));
#33338=CARTESIAN_POINT('Ctrl Pts',(-30.4216324926546,34.9545363298808,3.39699842932221));
#33339=CARTESIAN_POINT('Ctrl Pts',(-32.5122858139794,31.1562005618773,3.23999830196995));
#33340=CARTESIAN_POINT('Ctrl Pts',(-36.8336963111821,30.8046366333671,3.0829981746177));
#33341=CARTESIAN_POINT('Ctrl Pts',(-39.5108137360388,34.2150952689444,2.92599804726545));
#33342=CARTESIAN_POINT('Ctrl Pts',(-38.1430412058191,38.3293855376367,2.7689979199132));
#33343=CARTESIAN_POINT('Ctrl Pts',(-33.9568734797841,39.4581837921304,2.61199779256094));
#33344=CARTESIAN_POINT('Ctrl Pts',(-30.7060872988067,36.5892859950694,2.45499766520869));
#33345=CARTESIAN_POINT('Ctrl Pts',(-31.3056938569536,32.2952599480705,2.29799753785643));
#33346=CARTESIAN_POINT('Ctrl Pts',(-35.2180201227033,30.4266007598144,2.14099741050418));
#33347=CARTESIAN_POINT('Ctrl Pts',(-38.9348457584559,32.6589515260392,1.98399728315193));
#33348=CARTESIAN_POINT('Ctrl Pts',(-39.1232572406452,36.9905449712614,1.82699715579967));
#33349=CARTESIAN_POINT('Ctrl Pts',(-35.6143048269655,39.5371935081385,1.66999702844742));
#33350=CARTESIAN_POINT('Ctrl Pts',(-31.554498518323,38.0153054300115,1.51299690109517));
#33351=CARTESIAN_POINT('Ctrl Pts',(-30.5843081818037,33.7895472627506,1.35599677374291));
#33352=CARTESIAN_POINT('Ctrl Pts',(-33.5737075582741,30.6492474828669,1.19899664639066));
#33353=CARTESIAN_POINT('Ctrl Pts',(-37.8420841058543,31.4102411296202,1.04199651903841));
#33354=CARTESIAN_POINT('Ctrl Pts',(-39.5619223582134,35.3903431584975,0.884996391686153));
#33355=CARTESIAN_POINT('Ctrl Pts',(-37.1910696937641,39.0201444390132,0.7279962643339));
#33356=CARTESIAN_POINT('Ctrl Pts',(-32.8554061531891,39.0456001821187,0.570996136981647));
#33357=CARTESIAN_POINT('Ctrl Pts',(-30.4429366066027,35.4422062820125,0.413996009629392));
#33358=CARTESIAN_POINT('Ctrl Pts',(-32.116596037163,31.4445412420153,0.25699588227714));
#33359=CARTESIAN_POINT('Ctrl Pts',(-36.3762946811041,30.6305215911411,0.0999957549248848));
#33360=CARTESIAN_POINT('Ctrl Pts',(-39.4009794927627,33.7440564952096,-0.057004372427367));
#33361=CARTESIAN_POINT('Ctrl Pts',(-38.7860963780679,36.5549589254462,-0.161671123995537));
#33362=CARTESIAN_POINT('Ctrl Pts',(-37.9552630411254,37.5267093987113,-0.214004499779622));
#33363=CARTESIAN_POINT('Ctrl Pts',(-35.9563385206894,31.4227955987545,8.21400449977962));
#33364=CARTESIAN_POINT('Ctrl Pts',(-37.1325959372044,31.7372591159268,8.16167112399554));
#33365=CARTESIAN_POINT('Ctrl Pts',(-39.1314861397082,33.6116189520467,8.05700437242738));
#33366=CARTESIAN_POINT('Ctrl Pts',(-38.4372220394899,37.6868249117579,7.90000424507511));
#33367=CARTESIAN_POINT('Ctrl Pts',(-34.6550080494404,39.3458240206473,7.74300411772287));
#33368=CARTESIAN_POINT('Ctrl Pts',(-31.1849796802547,37.1112166805582,7.5860039903706));
#33369=CARTESIAN_POINT('Ctrl Pts',(-31.1345145318363,32.9818137587874,7.42900386301836));
#33370=CARTESIAN_POINT('Ctrl Pts',(-34.5509632115484,30.6629550625048,7.2720037356661));
#33371=CARTESIAN_POINT('Ctrl Pts',(-38.3697220079671,32.2327604838143,7.11500360831385));
#33372=CARTESIAN_POINT('Ctrl Pts',(-39.166990263271,36.2841775250771,6.95800348096159));
#33373=CARTESIAN_POINT('Ctrl Pts',(-36.2275932273038,39.1839602767271,6.80100335360935));
#33374=CARTESIAN_POINT('Ctrl Pts',(-32.1874438377366,38.3319953452796,6.64400322625709));
#33375=CARTESIAN_POINT('Ctrl Pts',(-30.6693195563919,34.4921735803525,6.48700309890483));
#33376=CARTESIAN_POINT('Ctrl Pts',(-33.0345683933729,31.1077368710331,6.33000297155259));
#33377=CARTESIAN_POINT('Ctrl Pts',(-37.1622334356032,31.2135237769978,6.17300284420032));
#33378=CARTESIAN_POINT('Ctrl Pts',(-39.3510055801728,34.7146832529224,6.01600271684808));
#33379=CARTESIAN_POINT('Ctrl Pts',(-37.6381880046832,38.4716874963794,5.85900258949581));
#33380=CARTESIAN_POINT('Ctrl Pts',(-33.5596825685645,39.11559699904,5.70200246214357));
#33381=CARTESIAN_POINT('Ctrl Pts',(-30.7727232768428,36.0690108205182,5.54500233479131));
#33382=CARTESIAN_POINT('Ctrl Pts',(-31.7764037333916,32.0638325667482,5.38800220743906));
#33383=CARTESIAN_POINT('Ctrl Pts',(-35.6707138105653,30.6915437277723,5.23100208008681));
#33384=CARTESIAN_POINT('Ctrl Pts',(-38.9635884177054,33.1826890066978,5.07400195273455));
#33385=CARTESIAN_POINT('Ctrl Pts',(-38.7022752466618,37.3034344653991,4.9170018253823));
#33386=CARTESIAN_POINT('Ctrl Pts',(-35.1210963533887,39.3586681519579,4.76000169803004));
#33387=CARTESIAN_POINT('Ctrl Pts',(-31.4313291935845,37.5054422859516,4.6030015706778));
#33388=CARTESIAN_POINT('Ctrl Pts',(-30.9416233845026,33.4055622887757,4.44600144332554));
#33389=CARTESIAN_POINT('Ctrl Pts',(-34.091102819686,30.7354298821828,4.28900131597329));
#33390=CARTESIAN_POINT('Ctrl Pts',(-38.0555990765859,31.8893784134534,4.13200118862103));
#33391=CARTESIAN_POINT('Ctrl Pts',(-39.2801103271579,35.8326511627796,3.97500106126878));
#33392=CARTESIAN_POINT('Ctrl Pts',(-36.6666055859447,39.0292776269525,3.81800093391652));
#33393=CARTESIAN_POINT('Ctrl Pts',(-32.5586396271459,38.6128121869325,3.66100080656428));
#33394=CARTESIAN_POINT('Ctrl Pts',(-30.639864935887,34.9567034009586,3.50400067921202));
#33395=CARTESIAN_POINT('Ctrl Pts',(-32.6308651862137,31.3394190871117,3.34700055185977));
#33396=CARTESIAN_POINT('Ctrl Pts',(-36.7462913517739,31.0046128030999,3.19000042450751));
#33397=CARTESIAN_POINT('Ctrl Pts',(-39.2958013105393,34.2525085340193,3.03300029715526));
#33398=CARTESIAN_POINT('Ctrl Pts',(-37.9932250190614,38.1706870628692,2.876000169803));
#33399=CARTESIAN_POINT('Ctrl Pts',(-34.0065951433993,39.2456800252801,2.71900004245075));
#33400=CARTESIAN_POINT('Ctrl Pts',(-30.9107609206391,36.5135310965947,2.5619999150985));
#33401=CARTESIAN_POINT('Ctrl Pts',(-31.4817866355154,32.4241840741688,2.40499978774625));
#33402=CARTESIAN_POINT('Ctrl Pts',(-35.2076279765999,30.6445963856486,2.24799966039399));
#33403=CARTESIAN_POINT('Ctrl Pts',(-38.7472874197615,32.7705399311592,2.09099953304174));
#33404=CARTESIAN_POINT('Ctrl Pts',(-38.9267180811614,36.8956636643883,1.93399940568948));
#33405=CARTESIAN_POINT('Ctrl Pts',(-35.5850233760853,39.3209236645512,1.77699927833723));
#33406=CARTESIAN_POINT('Ctrl Pts',(-31.7187317751118,37.8715778961193,1.61999915098498));
#33407=CARTESIAN_POINT('Ctrl Pts',(-30.7947865264321,33.8472446970093,1.46299902363273));
#33408=CARTESIAN_POINT('Ctrl Pts',(-33.6416932068317,30.8566304310881,1.30599889628047));
#33409=CARTESIAN_POINT('Ctrl Pts',(-37.7066133387528,31.581350558394,1.14899876892822));
#33410=CARTESIAN_POINT('Ctrl Pts',(-39.3444737893792,35.371737063412,0.991998641575963));
#33411=CARTESIAN_POINT('Ctrl Pts',(-37.086630176448,38.8285202538281,0.834998514223711));
#33412=CARTESIAN_POINT('Ctrl Pts',(-32.9576303530114,38.8527626236071,0.677998386871457));
#33413=CARTESIAN_POINT('Ctrl Pts',(-30.6601535680437,35.421128079535,0.520998259519203));
#33414=CARTESIAN_POINT('Ctrl Pts',(-32.2540363563655,31.6140157217992,0.36399813216695));
#33415=CARTESIAN_POINT('Ctrl Pts',(-36.31069222556,30.8387971276259,0.206998004814696));
#33416=CARTESIAN_POINT('Ctrl Pts',(-39.1912024257666,33.8039222921716,0.0499978774624438));
#33417=CARTESIAN_POINT('Ctrl Pts',(-38.6056283266121,36.4808402609044,-0.0546688741057268));
#33418=CARTESIAN_POINT('Ctrl Pts',(-37.8143974874483,37.4062712808594,-0.107002249889811));
#33419=CARTESIAN_POINT('Ctrl Pts',(-35.9084720925035,31.6018409826581,8.32100674966943));
#33420=CARTESIAN_POINT('Ctrl Pts',(-37.0258557525633,31.9005650466595,8.26867337388535));
#33421=CARTESIAN_POINT('Ctrl Pts',(-38.9246979780591,33.681109870052,8.16400662231719));
#33422=CARTESIAN_POINT('Ctrl Pts',(-38.2651830194642,37.552344590298,8.00700649496492));
#33423=CARTESIAN_POINT('Ctrl Pts',(-34.6722755044984,39.1283078703588,7.85000636761267));
#33424=CARTESIAN_POINT('Ctrl Pts',(-31.3759281699498,37.005546565386,7.69300624026042));
#33425=CARTESIAN_POINT('Ctrl Pts',(-31.3279888911377,33.0828275365354,7.53600611290817));
#33426=CARTESIAN_POINT('Ctrl Pts',(-34.5734382940869,30.8800318042114,7.37900598555591));
#33427=CARTESIAN_POINT('Ctrl Pts',(-38.2010614834652,32.3712656979296,7.22200585820366));
#33428=CARTESIAN_POINT('Ctrl Pts',(-38.9584250576736,36.2199021770154,7.06500573085141));
#33429=CARTESIAN_POINT('Ctrl Pts',(-36.1661500230565,38.9745456920523,6.90800560349915));
#33430=CARTESIAN_POINT('Ctrl Pts',(-32.3282172298434,38.1652231067258,6.7510054761469));
#33431=CARTESIAN_POINT('Ctrl Pts',(-30.8860777439641,34.5175911875294,6.59400534879464));
#33432=CARTESIAN_POINT('Ctrl Pts',(-33.1329417086976,31.3025514994443,6.43700522144239));
#33433=CARTESIAN_POINT('Ctrl Pts',(-37.0540098419411,31.4030435843515,6.28000509409013));
#33434=CARTESIAN_POINT('Ctrl Pts',(-39.1332300836993,34.7289638588885,6.12300496673789));
#33435=CARTESIAN_POINT('Ctrl Pts',(-37.5061420461286,38.2979234195025,5.96600483938563));
#33436=CARTESIAN_POINT('Ctrl Pts',(-33.6317729940835,38.9096041168808,5.80900471203338));
#33437=CARTESIAN_POINT('Ctrl Pts',(-30.9843059259921,36.0155049451787,5.65200458468113));
#33438=CARTESIAN_POINT('Ctrl Pts',(-31.937750407041,32.2107929207913,5.49500445732887));
#33439=CARTESIAN_POINT('Ctrl Pts',(-35.6371434024388,30.9071895564043,5.33800432997662));
#33440=CARTESIAN_POINT('Ctrl Pts',(-38.765203832906,33.2736486243128,5.18100420262436));
#33441=CARTESIAN_POINT('Ctrl Pts',(-38.5169698465499,37.1881435113763,5.02400407527211));
#33442=CARTESIAN_POINT('Ctrl Pts',(-35.1150352675099,39.1405091302639,4.86700394791986));
#33443=CARTESIAN_POINT('Ctrl Pts',(-31.6099474560293,37.3800404845393,4.7100038205676));
#33444=CARTESIAN_POINT('Ctrl Pts',(-31.1447522856339,33.4853667058834,4.55300369321536));
#33445=CARTESIAN_POINT('Ctrl Pts',(-34.1365947251866,30.9488791314519,4.39600356586309));
#33446=CARTESIAN_POINT('Ctrl Pts',(-37.9026609583357,32.0450705052858,4.23900343851085));
#33447=CARTESIAN_POINT('Ctrl Pts',(-39.0658832630269,35.7909755048144,4.08200331115859));
#33448=CARTESIAN_POINT('Ctrl Pts',(-36.5831890395356,38.8276051814752,3.92500318380634));
#33449=CARTESIAN_POINT('Ctrl Pts',(-32.6808340158849,38.4319845706085,3.76800305645408));
#33450=CARTESIAN_POINT('Ctrl Pts',(-30.8580973791193,34.9588704720363,3.61100292910183));
#33451=CARTESIAN_POINT('Ctrl Pts',(-32.7494445584481,31.522637612346,3.45400280174958));
#33452=CARTESIAN_POINT('Ctrl Pts',(-36.6588863923657,31.2045889728327,3.29700267439732));
#33453=CARTESIAN_POINT('Ctrl Pts',(-39.0807888850399,34.2899217990943,3.14000254704507));
#33454=CARTESIAN_POINT('Ctrl Pts',(-37.8434088323037,38.0119885881016,2.98300241969281));
#33455=CARTESIAN_POINT('Ctrl Pts',(-34.0563168070145,39.0331762584299,2.82600229234057));
#33456=CARTESIAN_POINT('Ctrl Pts',(-31.1154345424715,36.4377761981199,2.66900216498831));
#33457=CARTESIAN_POINT('Ctrl Pts',(-31.6578794140771,32.553108200267,2.51200203763606));
#33458=CARTESIAN_POINT('Ctrl Pts',(-35.1972358304966,30.8625920114828,2.3550019102838));
#33459=CARTESIAN_POINT('Ctrl Pts',(-38.559729081067,32.8821283362792,2.19800178293155));
#33460=CARTESIAN_POINT('Ctrl Pts',(-38.7301789216776,36.8007823575152,2.04100165557929));
#33461=CARTESIAN_POINT('Ctrl Pts',(-35.555741925205,39.1046538209638,1.88400152822704));
#33462=CARTESIAN_POINT('Ctrl Pts',(-31.8829650319005,37.727850362227,1.72700140087479));
#33463=CARTESIAN_POINT('Ctrl Pts',(-31.0052648710604,33.904942131268,1.57000127352254));
#33464=CARTESIAN_POINT('Ctrl Pts',(-33.7096788553892,31.0640133793093,1.41300114617028));
#33465=CARTESIAN_POINT('Ctrl Pts',(-37.5711425716514,31.7524599871677,1.25600101881803));
#33466=CARTESIAN_POINT('Ctrl Pts',(-39.127025220545,35.3531309683265,1.09900089146578));
#33467=CARTESIAN_POINT('Ctrl Pts',(-36.982190659132,38.6368960686431,0.942000764113521));
#33468=CARTESIAN_POINT('Ctrl Pts',(-33.0598545528336,38.6599250650956,0.785000636761268));
#33469=CARTESIAN_POINT('Ctrl Pts',(-30.8773705294847,35.4000498770575,0.628000509409013));
#33470=CARTESIAN_POINT('Ctrl Pts',(-32.391476675568,31.7834902015831,0.471000382056762));
#33471=CARTESIAN_POINT('Ctrl Pts',(-36.2450897700159,31.0470726641105,0.314000254704506));
#33472=CARTESIAN_POINT('Ctrl Pts',(-38.9814253587705,33.8637880891336,0.157000127352255));
#33473=CARTESIAN_POINT('Ctrl Pts',(-38.4251602751564,36.4067215963626,0.0523333757840841));
#33474=CARTESIAN_POINT('Ctrl Pts',(-37.6735319337713,37.2858331630075,0.));
#33475=CARTESIAN_POINT('Ctrl Pts',(-37.6735319337713,37.2858331630075,0.));
#33476=CARTESIAN_POINT('Ctrl Pts',(-37.7506745369995,37.2087203555594,1.28363488612132E-16));
#33477=CARTESIAN_POINT('Ctrl Pts',(-37.8237047828546,37.1279853831031,-1.45961390077584E-15));
#33478=CARTESIAN_POINT('Ctrl Pts',(-37.8926303634218,37.044046747423,-1.27675647831893E-15));
#33479=CARTESIAN_POINT('Ctrl Pts',(-37.9633158416367,36.9579648812288,-1.08923010211539E-15));
#33480=CARTESIAN_POINT('Ctrl Pts',(-38.0296847428869,36.8685132102372,2.69373606469353E-15));
#33481=CARTESIAN_POINT('Ctrl Pts',(-38.0917154903142,36.776096981172,2.1094237467878E-15));
#33482=CARTESIAN_POINT('Ctrl Pts',(-38.1550372699928,36.6817573135345,1.51295026561079E-15));
#33483=CARTESIAN_POINT('Ctrl Pts',(-38.2138388545422,36.5843278170101,-6.22870230136456E-16));
#33484=CARTESIAN_POINT('Ctrl Pts',(-38.2680604999532,36.4842001218513,-1.22124532708767E-15));
#33485=CARTESIAN_POINT('Ctrl Pts',(-38.3198497467852,36.3885641838418,-1.7927771454093E-15));
#33486=CARTESIAN_POINT('Ctrl Pts',(-38.3674607433557,36.2904658682844,-1.21061342909026E-15));
#33487=CARTESIAN_POINT('Ctrl Pts',(-38.4108059167409,36.1902218218841,-1.49880108324396E-15));
#33488=CARTESIAN_POINT('Ctrl Pts',(-38.4178437109143,36.1739455698685,-1.54559303803029E-15));
#33489=CARTESIAN_POINT('Ctrl Pts',(-38.4247689668943,36.1576127105175,5.76904931418396E-16));
#33490=CARTESIAN_POINT('Ctrl Pts',(-38.4315812162273,36.1412245565248,6.10622663543836E-16));
#33491=CARTESIAN_POINT('Ctrl Pts',(-38.4380909127403,36.1255642505548,6.42842888099819E-16));
#33492=CARTESIAN_POINT('Ctrl Pts',(-38.4444943995979,36.1098606451587,1.94214412995646E-15));
#33493=CARTESIAN_POINT('Ctrl Pts',(-38.4507894645608,36.0941203888398,1.88737914186277E-15));
#33494=CARTESIAN_POINT('Ctrl Pts',(-38.4941748650482,35.9856390104596,1.50994047282167E-15));
#33495=CARTESIAN_POINT('Ctrl Pts',(-38.5324464076346,35.8753406458803,4.14672721999528E-16));
#33496=CARTESIAN_POINT('Ctrl Pts',(-38.5655754746426,35.7636570985597,-1.11022302462516E-16));
#33497=CARTESIAN_POINT('Ctrl Pts',(-38.599139072954,35.6505086745683,-6.43612508853869E-16));
#33498=CARTESIAN_POINT('Ctrl Pts',(-38.6274248054533,35.535937741082,5.81275891054099E-16));
#33499=CARTESIAN_POINT('Ctrl Pts',(-38.6503602739825,35.4203607919199,1.85962356624714E-15));
#33500=CARTESIAN_POINT('Ctrl Pts',(-38.6743352598313,35.2995454827809,3.19591052212541E-15));
#33501=CARTESIAN_POINT('Ctrl Pts',(-38.692464786516,35.1776300814803,-8.4407659709162E-16));
#33502=CARTESIAN_POINT('Ctrl Pts',(-38.7046104310317,35.0550669428354,-1.38777878078145E-15));
#33503=CARTESIAN_POINT('Ctrl Pts',(-38.7137196644185,34.9631445888517,-1.79555541854881E-15));
#33504=CARTESIAN_POINT('Ctrl Pts',(-38.7194618408911,34.8708572859148,2.82896256593911E-15));
#33505=CARTESIAN_POINT('Ctrl Pts',(-38.721755434165,34.7783924177428,2.94209101525666E-15));
#33506=CARTESIAN_POINT('Ctrl Pts',(-38.7223030074901,34.7563173201712,2.96909934400004E-15));
#33507=CARTESIAN_POINT('Ctrl Pts',(-38.7226538674535,34.7342275752707,-2.60000342473094E-16));
#33508=CARTESIAN_POINT('Ctrl Pts',(-38.7228068022813,34.7121547959299,-2.77555756156289E-16));
#33509=CARTESIAN_POINT('Ctrl Pts',(-38.7236416666969,34.5916604762348,-3.73389977849103E-16));
#33510=CARTESIAN_POINT('Ctrl Pts',(-38.7185883671926,34.4715209673338,1.72146304164403E-15));
#33511=CARTESIAN_POINT('Ctrl Pts',(-38.7075779418993,34.3521623032552,1.58206781009085E-15));
#33512=CARTESIAN_POINT('Ctrl Pts',(-38.6966381726954,34.2335695874665,1.44356710546673E-15));
#33513=CARTESIAN_POINT('Ctrl Pts',(-38.6798177366068,34.1157468505408,1.14312909921041E-17));
#33514=CARTESIAN_POINT('Ctrl Pts',(-38.6569995558515,33.9990991317786,-2.77555756156289E-16));
#33515=CARTESIAN_POINT('Ctrl Pts',(-38.654125907022,33.9844088905153,-3.13949862184534E-16));
#33516=CARTESIAN_POINT('Ctrl Pts',(-38.6511570658937,33.9697372784049,2.13659354022824E-15));
#33517=CARTESIAN_POINT('Ctrl Pts',(-38.6480927394297,33.9550851007466,2.1094237467878E-15));
#33518=CARTESIAN_POINT('Ctrl Pts',(-38.6241822697972,33.8407564046822,1.89676768741005E-15));
#33519=CARTESIAN_POINT('Ctrl Pts',(-38.5944625878303,33.7276104213963,7.3858195394121E-16));
#33520=CARTESIAN_POINT('Ctrl Pts',(-38.5592398399973,33.6159136444833,2.4980018054066E-16));
#33521=CARTESIAN_POINT('Ctrl Pts',(-38.5372745858279,33.5462584288701,-5.50089711192647E-17));
#33522=CARTESIAN_POINT('Ctrl Pts',(-38.5131681698132,33.4771668829623,6.13912691963219E-16));
#33523=CARTESIAN_POINT('Ctrl Pts',(-38.4869849848521,33.408705821156,6.93889390390723E-16));
#33524=CARTESIAN_POINT('Ctrl Pts',(-38.478035242453,33.3853049679579,7.21226433226402E-16));
#33525=CARTESIAN_POINT('Ctrl Pts',(-38.4688427975352,33.3619777978058,1.17968218996551E-15));
#33526=CARTESIAN_POINT('Ctrl Pts',(-38.4594100345669,33.3387270476804,1.30451205393456E-15));
#33527=CARTESIAN_POINT('Ctrl Pts',(-38.4526611227965,33.3220917032197,1.39382477610025E-15));
#33528=CARTESIAN_POINT('Ctrl Pts',(-38.4457886431155,33.3054943585584,8.23245697379087E-16));
#33529=CARTESIAN_POINT('Ctrl Pts',(-38.4388005380928,33.2889523169239,7.49400541621981E-16));
#33530=CARTESIAN_POINT('Ctrl Pts',(-38.3928792100309,33.1802486671866,2.64137711097381E-16));
#33531=CARTESIAN_POINT('Ctrl Pts',(-38.3419048511529,33.0737714082961,1.17255001397609E-15));
#33532=CARTESIAN_POINT('Ctrl Pts',(-38.2862359020984,32.9697748885158,9.43689570931383E-16));
#33533=CARTESIAN_POINT('Ctrl Pts',(-38.2286517312081,32.8622004961707,7.06955465363536E-16));
#33534=CARTESIAN_POINT('Ctrl Pts',(-38.1660442194156,32.7572797837933,2.65690729149937E-16));
#33535=CARTESIAN_POINT('Ctrl Pts',(-38.0987547078419,32.6553015987604,4.44089209850063E-16));
#33536=CARTESIAN_POINT('Ctrl Pts',(-38.0308320192805,32.5523638252493,6.24166374344619E-16));
#33537=CARTESIAN_POINT('Ctrl Pts',(-37.9581383688774,32.4524234721426,-1.26765506881022E-15));
#33538=CARTESIAN_POINT('Ctrl Pts',(-37.8809743110047,32.3557958917759,-1.62370117351429E-15));
#33539=CARTESIAN_POINT('Ctrl Pts',(-37.82656120339,32.2876578612733,-1.87477110872936E-15));
#33540=CARTESIAN_POINT('Ctrl Pts',(-37.7699241047827,32.2211674765398,1.39931090156461E-15));
#33541=CARTESIAN_POINT('Ctrl Pts',(-37.7111553490298,32.1564437978227,1.60982338570648E-15));
#33542=CARTESIAN_POINT('Ctrl Pts',(-37.6849229569216,32.1275533287794,1.70378906452554E-15));
#33543=CARTESIAN_POINT('Ctrl Pts',(-37.6582657142846,32.0990149717255,2.33543966985802E-16));
#33544=CARTESIAN_POINT('Ctrl Pts',(-37.6311912225754,32.0708398884709,3.05311331771918E-16));
#33545=CARTESIAN_POINT('Ctrl Pts',(-37.6195692277271,32.0587454537553,3.36118186902312E-16));
#33546=CARTESIAN_POINT('Ctrl Pts',(-37.6078717672662,32.0467194961249,-1.14899013469077E-15));
#33547=CARTESIAN_POINT('Ctrl Pts',(-37.5961059477358,32.034769281675,-1.17961196366423E-15));
#33548=CARTESIAN_POINT('Ctrl Pts',(-37.5076636824121,31.9449409416833,-1.40979260818075E-15));
#33549=CARTESIAN_POINT('Ctrl Pts',(-37.4152620841693,31.8592852286376,-2.45663089159861E-15));
#33550=CARTESIAN_POINT('Ctrl Pts',(-37.3192298936088,31.778120294682,-2.019218126037E-15));
#33551=CARTESIAN_POINT('Ctrl Pts',(-37.2371898445147,31.7087813040001,-1.64553754506066E-15));
#33552=CARTESIAN_POINT('Ctrl Pts',(-37.1524990927587,31.6427198578901,-2.42654488972963E-15));
#33553=CARTESIAN_POINT('Ctrl Pts',(-37.0653383821438,31.5801518871639,-2.52575738102223E-15));
#33554=CARTESIAN_POINT('Ctrl Pts',(-37.0262273476737,31.5520761860535,-2.57027632928952E-15));
#33555=CARTESIAN_POINT('Ctrl Pts',(-36.9866187071144,31.524704156366,-1.17712968719052E-15));
#33556=CARTESIAN_POINT('Ctrl Pts',(-36.946527548351,31.4980566647868,-6.31439345255558E-16));
#33557=CARTESIAN_POINT('Ctrl Pts',(-36.9192934800282,31.479954927928,-2.60749933581654E-16));
#33558=CARTESIAN_POINT('Ctrl Pts',(-36.89183110785,31.4621841581827,-1.11508673223599E-15));
#33559=CARTESIAN_POINT('Ctrl Pts',(-36.8641751230777,31.4447696709256,-1.17267306976032E-15));
#33560=CARTESIAN_POINT('Ctrl Pts',(-36.757370770553,31.3775168483861,-1.39506513224507E-15));
#33561=CARTESIAN_POINT('Ctrl Pts',(-36.6476196941272,31.3155308365787,-2.17833836995006E-15));
#33562=CARTESIAN_POINT('Ctrl Pts',(-36.5352238715355,31.2591452947779,-6.38378239159465E-16));
#33563=CARTESIAN_POINT('Ctrl Pts',(-36.4331301648989,31.2079280090246,7.60430312613923E-16));
#33564=CARTESIAN_POINT('Ctrl Pts',(-36.3288535333025,31.1613315369686,5.40797342115576E-17));
#33565=CARTESIAN_POINT('Ctrl Pts',(-36.2225969429285,31.1196350477066,-1.58727198051878E-16));
#33566=CARTESIAN_POINT('Ctrl Pts',(-36.1671664218874,31.0978833792477,-2.38185072021888E-16));
#33567=CARTESIAN_POINT('Ctrl Pts',(-36.1111967480356,31.0774656809663,2.2162435752245E-16));
#33568=CARTESIAN_POINT('Ctrl Pts',(-36.0547320440516,31.0583698407596,1.38777878078145E-16));
#33569=CARTESIAN_POINT('Ctrl Pts',(-38.5153120432796,35.002811202661,7.11258330249199));
#33570=CARTESIAN_POINT('Ctrl Pts',(-38.5180431912138,35.3538028140734,7.09672411194513));
#33571=CARTESIAN_POINT('Ctrl Pts',(-38.4695957643305,35.7040585809451,7.08086492139827));
#33572=CARTESIAN_POINT('Ctrl Pts',(-38.3668186228693,36.0375700163406,7.06500573085141));
#33573=CARTESIAN_POINT('Ctrl Pts',(-38.0276667128012,37.1381166820277,7.01267235506732));
#33574=CARTESIAN_POINT('Ctrl Pts',(-37.0969083679288,38.05633118704,6.96033897928324));
#33575=CARTESIAN_POINT('Ctrl Pts',(-35.9918737299572,38.3805513419917,6.90800560349915));
#33576=CARTESIAN_POINT('Ctrl Pts',(-34.8868390919855,38.7047714969434,6.85567222771507));
#33577=CARTESIAN_POINT('Ctrl Pts',(-33.6075281609145,38.4349973018346,6.80333885193099));
#33578=CARTESIAN_POINT('Ctrl Pts',(-32.7275161143991,37.6921715510808,6.7510054761469));
#33579=CARTESIAN_POINT('Ctrl Pts',(-31.8475040678837,36.949345800327,6.69867210036282));
#33580=CARTESIAN_POINT('Ctrl Pts',(-31.3667909059239,35.7334684939282,6.64633872457873));
#33581=CARTESIAN_POINT('Ctrl Pts',(-31.5009116523996,34.5896898927146,6.59400534879465));
#33582=CARTESIAN_POINT('Ctrl Pts',(-31.6350323988753,33.445911291501,6.54167197301056));
#33583=CARTESIAN_POINT('Ctrl Pts',(-32.3839870537864,32.3742313954726,6.48933859722648));
#33584=CARTESIAN_POINT('Ctrl Pts',(-33.4119757367826,31.8551401282763,6.43700522144239));
#33585=CARTESIAN_POINT('Ctrl Pts',(-34.4399644197788,31.33604886108,6.38467184565831));
#33586=CARTESIAN_POINT('Ctrl Pts',(-35.74698713086,31.3695462227158,6.33233846987422));
#33587=CARTESIAN_POINT('Ctrl Pts',(-36.7470351933603,31.9406149492898,6.28000509409014));
#33588=CARTESIAN_POINT('Ctrl Pts',(-37.7470832558605,32.5116836758639,6.22767171830605));
#33589=CARTESIAN_POINT('Ctrl Pts',(-38.4401566697799,33.6203237673762,6.17533834252197));
#33590=CARTESIAN_POINT('Ctrl Pts',(-38.5155120371445,34.769470406568,6.12300496673789));
#33591=CARTESIAN_POINT('Ctrl Pts',(-38.5205141244106,34.8457507296795,6.11953107865592));
#33592=CARTESIAN_POINT('Ctrl Pts',(-38.5227943601281,34.922209536826,6.11605719057395));
#33593=CARTESIAN_POINT('Ctrl Pts',(-38.5224238694764,34.9986908177615,6.11258330249199));
#33594=CARTESIAN_POINT('Origin',(35.,-35.,4.));
#33595=CARTESIAN_POINT('Origin',(-35.,-35.,4.));
#33596=CARTESIAN_POINT('Origin',(-35.,35.,4.));
#33597=CARTESIAN_POINT('Origin',(35.,35.,4.));
#33598=CARTESIAN_POINT('Origin',(50.,50.,0.));
#33599=CARTESIAN_POINT('',(50.,50.,0.));
#33600=CARTESIAN_POINT('',(-50.,50.,0.));
#33601=CARTESIAN_POINT('',(50.,50.,0.));
#33602=CARTESIAN_POINT('',(-50.,50.,0.));
#33603=CARTESIAN_POINT('',(50.,50.,0.));
#33604=CARTESIAN_POINT('Origin',(50.,-50.,0.));
#33605=CARTESIAN_POINT('',(50.,-50.,0.));
#33606=CARTESIAN_POINT('',(50.,-50.,0.));
#33607=CARTESIAN_POINT('',(50.,-50.,0.));
#33608=CARTESIAN_POINT('Origin',(-50.,-50.,0.));
#33609=CARTESIAN_POINT('',(-50.,-50.,0.));
#33610=CARTESIAN_POINT('',(-50.,-50.,0.));
#33611=CARTESIAN_POINT('',(-50.,-50.,0.));
#33612=CARTESIAN_POINT('Origin',(-50.,50.,0.));
#33613=CARTESIAN_POINT('',(-50.,50.,0.));
#33614=CARTESIAN_POINT('Origin',(0.,0.,0.));
#97434=UNCERTAINTY_MEASURE_WITH_UNIT(LENGTH_MEASURE(0.01),#97476,
'DISTANCE_ACCURACY_VALUE',
'Maximum model space distance between geometric entities at asserted c
onnectivities');
#97452=UNCERTAINTY_MEASURE_WITH_UNIT(LENGTH_MEASURE(0.01),#97476,
'DISTANCE_ACCURACY_VALUE',
'Maximum model space distance between geometric entities at asserted c
onnectivities');
#97457=(
GEOMETRIC_REPRESENTATION_CONTEXT(3)
GLOBAL_UNCERTAINTY_ASSIGNED_CONTEXT((#97434))
GLOBAL_UNIT_ASSIGNED_CONTEXT((#97476,#97478,#97479))
REPRESENTATION_CONTEXT('','3D')
);
#97475=(
GEOMETRIC_REPRESENTATION_CONTEXT(3)
GLOBAL_UNCERTAINTY_ASSIGNED_CONTEXT((#97452))
GLOBAL_UNIT_ASSIGNED_CONTEXT((#97476,#97478,#97479))
REPRESENTATION_CONTEXT('','3D')
);
#97476=(
LENGTH_UNIT()
NAMED_UNIT(*)
SI_UNIT(.MILLI.,.METRE.)
);
#97478=(
NAMED_UNIT(*)
PLANE_ANGLE_UNIT()
SI_UNIT($,.RADIAN.)
);
#97479=(
NAMED_UNIT(*)
SI_UNIT($,.STERADIAN.)
SOLID_ANGLE_UNIT()
);
#97484=SHAPE_DEFINITION_REPRESENTATION(#97506,#97607);
#97506=PRODUCT_DEFINITION_SHAPE('',$,#97630);
#97607=SHAPE_REPRESENTATION('',(#22082),#97457);
#97625=PRODUCT_DEFINITION_CONTEXT('part definition',#97693,'design');
#97630=PRODUCT_DEFINITION('Corner plate','Corner plate',#97652,#97625);
#97652=PRODUCT_DEFINITION_FORMATION('',$,#97699);
#97693=APPLICATION_CONTEXT(
'Core Data for Automotive Mechanical Design Process');
#97694=PRODUCT_CONTEXT('part definition',#97693,'mechanical');
#97699=PRODUCT('Corner plate','Corner plate',
'Weld rails to upper face. Four M8x1 attachment taps on 70 mm square p
attern match the leg plate clearance holes.',(#97694));
#97719=PRESENTATION_STYLE_ASSIGNMENT((#97726));
#97726=SURFACE_STYLE_USAGE(.BOTH.,#97733);
#97733=SURFACE_SIDE_STYLE('',(#97740));
#97740=SURFACE_STYLE_FILL_AREA(#97747);
#97747=FILL_AREA_STYLE('Sky blue',(#97754));
#97754=FILL_AREA_STYLE_COLOUR('Sky blue',#97761);
#97761=COLOUR_RGB('Sky blue',0.317647058823529,0.686274509803922,0.890196078431372);
ENDSEC;
END-ISO-10303-21;
